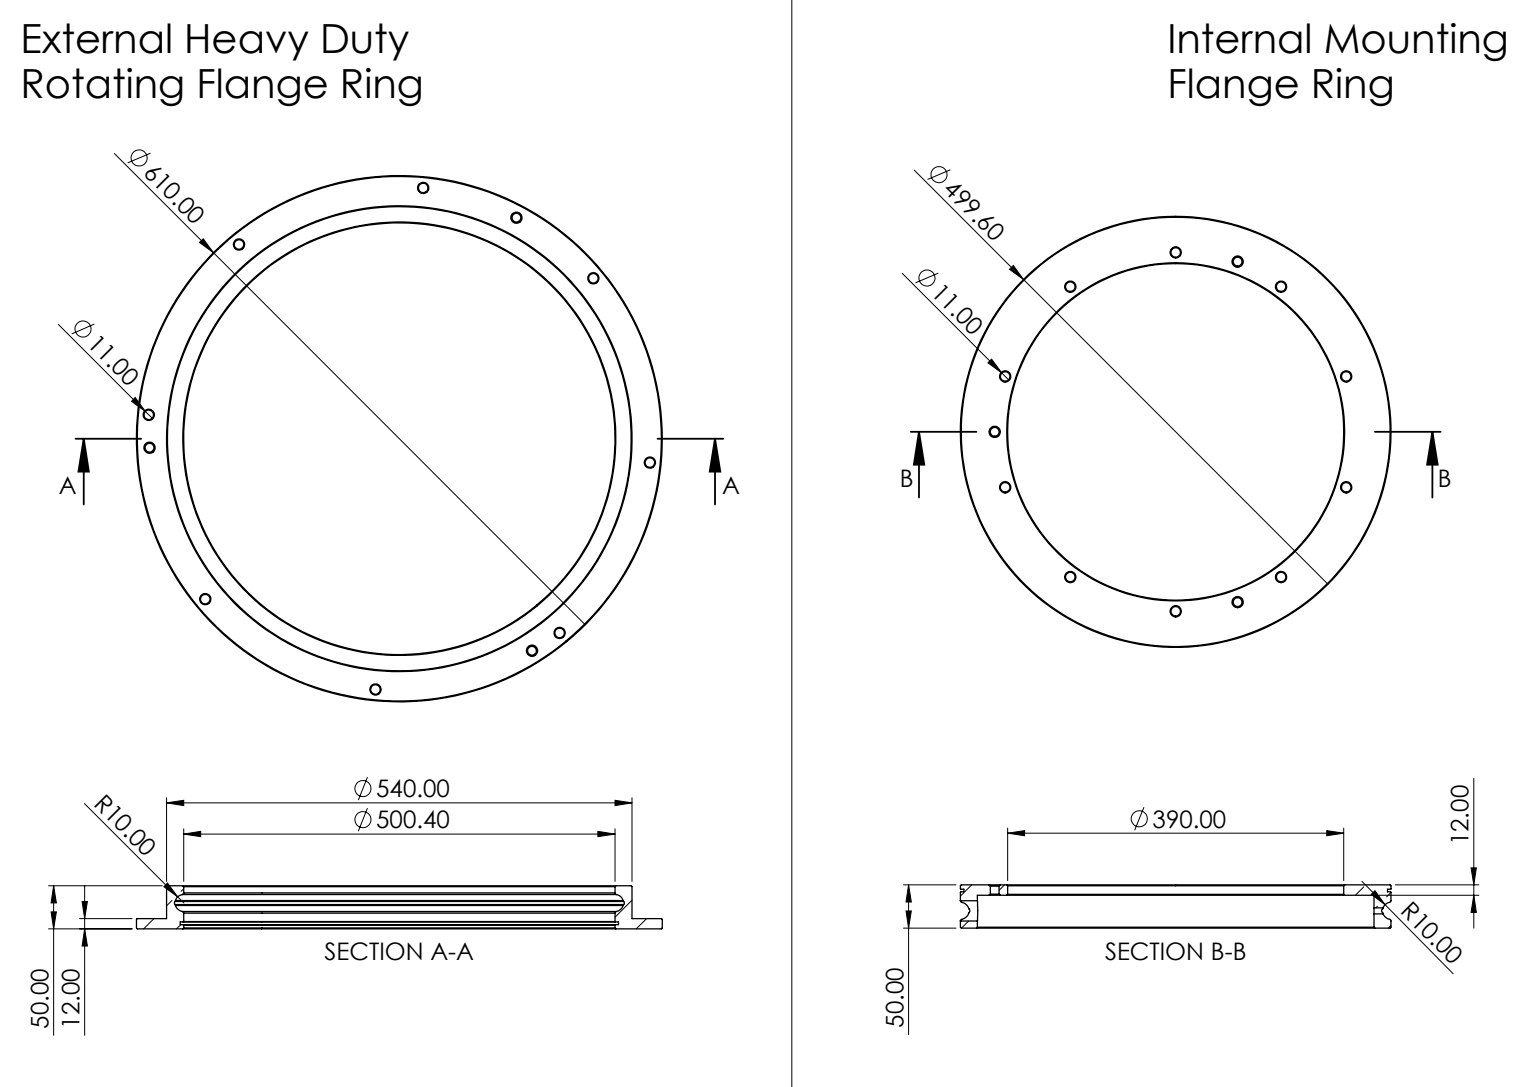
ISO-10303-21;
HEADER;
FILE_DESCRIPTION (('STEP AP214'),
    '1' );
FILE_NAME ('Internal Mounting Flange Ring.step',
    '2026-10-09T12:49:55',
    ( '' ),
    ( '' ),
    'SwSTEP 2.0',
    'SolidWorks 2026',
    '' );
FILE_SCHEMA (( 'AUTOMOTIVE_DESIGN' ));
ENDSEC;

DATA;
#5=TOROIDAL_SURFACE ( 'NONE', #5776, 250.0000000000000000, 10.00000000000000000 ) ;
#9=ORIENTED_EDGE ( 'NONE', *, *, #8914, .T. ) ;
#13=ADVANCED_FACE ( 'NONE', ( #7160 ), #9859, .F. ) ;
#18=CYLINDRICAL_SURFACE ( 'NONE', #6462, 5.500000000000005329 ) ;
#20=CARTESIAN_POINT ( 'NONE',  ( -243.1949234122827193, -7.480730365350286348, 9.061063672199042074 ) ) ;
#22=ORIENTED_EDGE ( 'NONE', *, *, #3438, .F. ) ;
#23=CARTESIAN_POINT ( 'NONE',  ( -230.0000000000000000, 18.00000000000000000, 0.000000000000000000 ) ) ;
#24=LINE ( 'NONE', #4986, #10827 ) ;
#25=CARTESIAN_POINT ( 'NONE',  ( 0.000000000000000000, 22.00000000000000000, 0.000000000000000000 ) ) ;
#28=DIRECTION ( 'NONE',  ( 0.000000000000000000, 1.000000000000000000, 0.000000000000000000 ) ) ;
#29=PLANE ( 'NONE',  #10608 ) ;
#33=CARTESIAN_POINT ( 'NONE',  ( 122.2593324768346008, 18.00000000000000000, 161.7755348299889988 ) ) ;
#36=CARTESIAN_POINT ( 'NONE',  ( -244.7823818444411188, 8.610125652527095497, 7.996289171610727387 ) ) ;
#37=EDGE_LOOP ( 'NONE', ( #12294, #12083 ) ) ;
#43=CARTESIAN_POINT ( 'NONE',  ( 6.735557395310442023E-16, 19.00000000000000000, 213.5000000000000000 ) ) ;
#44=ORIENTED_EDGE ( 'NONE', *, *, #3957, .F. ) ;
#49=CYLINDRICAL_SURFACE ( 'NONE', #12751, 249.7999999999999829 ) ;
#50=CARTESIAN_POINT ( 'NONE',  ( 6.735557395310442023E-16, 19.00000000000000000, -202.4999999999999716 ) ) ;
#58=VERTEX_POINT ( 'NONE', #5076 ) ;
#59=EDGE_CURVE ( 'NONE', #2857, #11921, #819, .T. ) ;
#61=CARTESIAN_POINT ( 'NONE',  ( -249.1369139485392168, 10.36343465138863529, -5.538914405136962316 ) ) ;
#68=DIRECTION ( 'NONE',  ( 8.659560562354926695E-17, 0.7071067811865480168, -0.7071067811865470176 ) ) ;
#70=AXIS2_PLACEMENT_3D ( 'NONE', #7490, #8365, #9292 ) ;
#71=CARTESIAN_POINT ( 'NONE',  ( -245.4148443366356389, -8.946846751066603431, -7.616852152915439156 ) ) ;
#73=CARTESIAN_POINT ( 'NONE',  ( -229.7583704989254443, -5.204493534573133573, 10.54155285988093382 ) ) ;
#78=ORIENTED_EDGE ( 'NONE', *, *, #7931, .F. ) ;
#82=FACE_OUTER_BOUND ( 'NONE', #8092, .T. ) ;
#84=CIRCLE ( 'NONE', #11996, 6.500000000000005329 ) ;
#88=CONICAL_SURFACE ( 'NONE', #12605, 5.500000000000005329, 0.7853981633974461696 ) ;
#89=CARTESIAN_POINT ( 'NONE',  ( -243.1551830321760690, -7.446108171798711872, 9.089443071778552152 ) ) ;
#91=FACE_BOUND ( 'NONE', #3077, .T. ) ;
#98=FACE_BOUND ( 'NONE', #10727, .T. ) ;
#102=CARTESIAN_POINT ( 'NONE',  ( -243.6022064859786269, 7.815160994106106429, 8.774769236968495534 ) ) ;
#103=CONICAL_SURFACE ( 'NONE', #1806, 5.500000000000005329, 0.7853981633974461696 ) ;
#105=EDGE_LOOP ( 'NONE', ( #5377, #568, #8957, #6732 ) ) ;
#107=EDGE_CURVE ( 'NONE', #6490, #4415, #2518, .T. ) ;
#108=EDGE_LOOP ( 'NONE', ( #11966, #7349 ) ) ;
#111=ORIENTED_EDGE ( 'NONE', *, *, #3767, .F. ) ;
#116=CARTESIAN_POINT ( 'NONE',  ( 239.1963018252363042, 1.024882057239583366, 3.346595946712579206 ) ) ;
#117=EDGE_CURVE ( 'NONE', #171, #5643, #5501, .T. ) ;
#119=EDGE_CURVE ( 'NONE', #4577, #1020, #8907, .T. ) ;
#120=CARTESIAN_POINT ( 'NONE',  ( -238.7109915777814138, -2.671037648644427152E-08, -11.74999999995326050 ) ) ;
#121=DIRECTION ( 'NONE',  ( 0.000000000000000000, 1.000000000000000000, 0.000000000000000000 ) ) ;
#127=CIRCLE ( 'NONE', #974, 239.8169934640564804 ) ;
#131=EDGE_LOOP ( 'NONE', ( #6897, #5787, #9258, #12917 ) ) ;
#134=DIRECTION ( 'NONE',  ( 0.000000000000000000, 0.000000000000000000, 1.000000000000000000 ) ) ;
#135=EDGE_CURVE ( 'NONE', #12433, #12610, #12359, .T. ) ;
#136=CARTESIAN_POINT ( 'NONE',  ( -243.1925160140377216, -7.478514340598183097, -9.062807757124144103 ) ) ;
#137=ADVANCED_FACE ( 'NONE', ( #98, #7027 ), #29, .F. ) ;
#139=CARTESIAN_POINT ( 'NONE',  ( 240.4181131690920097, 2.891045149275324633, 1.982248008065000233 ) ) ;
#143=ORIENTED_EDGE ( 'NONE', *, *, #1183, .T. ) ;
#144=ORIENTED_EDGE ( 'NONE', *, *, #3305, .F. ) ;
#146=FACE_OUTER_BOUND ( 'NONE', #6350, .T. ) ;
#147=CARTESIAN_POINT ( 'NONE',  ( 239.5387464286556565, -1.581210110862248941, -3.124650852508605858 ) ) ;
#149=DIRECTION ( 'NONE',  ( 0.000000000000000000, 1.000000000000000000, 0.000000000000000000 ) ) ;
#150=CARTESIAN_POINT ( 'NONE',  ( 0.000000000000000000, -9.830508068699650437, 0.000000000000000000 ) ) ;
#152=CARTESIAN_POINT ( 'NONE',  ( -246.6649006625763718, -9.461692665201230312, 6.966985664009688328 ) ) ;
#154=EDGE_LOOP ( 'NONE', ( #1351, #3008, #4241, #9314 ) ) ;
#155=CARTESIAN_POINT ( 'NONE',  ( 240.6084075703383292, -3.437342788167941698, 0.6677429272691086659 ) ) ;
#156=CARTESIAN_POINT ( 'NONE',  ( 229.9948761773756587, -3.146545554286515056, -1.549783278019676303 ) ) ;
#157=VERTEX_POINT ( 'NONE', #8121 ) ;
#158=VERTEX_POINT ( 'NONE', #1956 ) ;
#159=CARTESIAN_POINT ( 'NONE',  ( 122.2593324768334071, 18.00000000000000000, -168.2755348299895104 ) ) ;
#160=DIRECTION ( 'NONE',  ( 0.000000000000000000, 1.000000000000000000, 0.000000000000000000 ) ) ;
#166=CARTESIAN_POINT ( 'NONE',  ( -242.4885533041308179, 6.811171349317773682, 9.574815119040657407 ) ) ;
#167=VERTEX_POINT ( 'NONE', #4213 ) ;
#171=VERTEX_POINT ( 'NONE', #8621 ) ;
#176=ADVANCED_FACE ( 'NONE', ( #6424 ), #11036, .F. ) ;
#178=DIRECTION ( 'NONE',  ( 0.000000000000000000, 0.000000000000000000, 1.000000000000000000 ) ) ;
#180=LINE ( 'NONE', #8188, #691 ) ;
#184=EDGE_LOOP ( 'NONE', ( #4999, #5010, #6703, #1968 ) ) ;
#185=DIRECTION ( 'NONE',  ( 0.000000000000000000, 0.000000000000000000, 1.000000000000000000 ) ) ;
#186=DIRECTION ( 'NONE',  ( 0.000000000000000000, 1.000000000000000000, 0.000000000000000000 ) ) ;
#188=CIRCLE ( 'NONE', #5900, 6.499999999999999112 ) ;
#189=EDGE_LOOP ( 'NONE', ( #9728, #4932, #9679, #1428 ) ) ;
#192=AXIS2_PLACEMENT_3D ( 'NONE', #6124, #12263, #134 ) ;
#196=CARTESIAN_POINT ( 'NONE',  ( -246.9758887735252699, -9.561393943077655777, -6.829510937495726353 ) ) ;
#197=CIRCLE ( 'NONE', #11695, 196.0000000000000000 ) ;
#199=CARTESIAN_POINT ( 'NONE',  ( 240.6075165363340318, 3.437532598196324063, 0.7648284528981581509 ) ) ;
#200=EDGE_CURVE ( 'NONE', #7619, #9887, #12317, .T. ) ;
#201=EDGE_CURVE ( 'NONE', #6448, #6354, #188, .T. ) ;
#203=CIRCLE ( 'NONE', #9142, 2.000000000000001776 ) ;
#207=CARTESIAN_POINT ( 'NONE',  ( -248.9051445890450225, 10.17462340872661741, 5.878044170807267044 ) ) ;
#208=DIRECTION ( 'NONE',  ( 0.000000000000000000, 0.7071067811865480168, 0.7071067811865470176 ) ) ;
#209=DIRECTION ( 'NONE',  ( 8.659560562354913137E-17, -0.7071067811865489050, 0.7071067811865460184 ) ) ;
#211=DIRECTION ( 'NONE',  ( 0.000000000000000000, 0.000000000000000000, 1.000000000000000000 ) ) ;
#215=ORIENTED_EDGE ( 'NONE', *, *, #11212, .T. ) ;
#216=DIRECTION ( 'NONE',  ( 0.000000000000000000, 0.000000000000000000, 1.000000000000000000 ) ) ;
#218=EDGE_CURVE ( 'NONE', #9833, #1462, #5421, .T. ) ;
#221=ORIENTED_EDGE ( 'NONE', *, *, #12738, .T. ) ;
#223=FACE_OUTER_BOUND ( 'NONE', #154, .T. ) ;
#224=DIRECTION ( 'NONE',  ( 0.000000000000000000, 0.000000000000000000, 1.000000000000000000 ) ) ;
#228=DIRECTION ( 'NONE',  ( 0.000000000000000000, 0.000000000000000000, 1.000000000000000000 ) ) ;
#234=ORIENTED_EDGE ( 'NONE', *, *, #10382, .T. ) ;
#238=DIRECTION ( 'NONE',  ( 0.000000000000000000, 1.000000000000000000, 0.000000000000000000 ) ) ;
#243=DIRECTION ( 'NONE',  ( 0.000000000000000000, -0.7071067811865489050, -0.7071067811865460184 ) ) ;
#247=AXIS2_PLACEMENT_3D ( 'NONE', #6656, #10577, #2507 ) ;
#248=CARTESIAN_POINT ( 'NONE',  ( -249.2724874750463755, -10.50618518648515476, 5.261424415983393388 ) ) ;
#249=ORIENTED_EDGE ( 'NONE', *, *, #11663, .F. ) ;
#254=DIRECTION ( 'NONE',  ( 0.000000000000000000, 0.000000000000000000, 1.000000000000000000 ) ) ;
#259=CARTESIAN_POINT ( 'NONE',  ( -229.9627996858143888, 10.99879348686639879, 4.151745503392231029 ) ) ;
#260=AXIS2_PLACEMENT_3D ( 'NONE', #6805, #2654, #10860 ) ;
#261=FILL_AREA_STYLE_COLOUR ( '', #9272 ) ;
#265=AXIS2_PLACEMENT_3D ( 'NONE', #9269, #11198, #3992 ) ;
#267=ORIENTED_EDGE ( 'NONE', *, *, #6171, .T. ) ;
#273=CARTESIAN_POINT ( 'NONE',  ( -249.2624683435426789, 10.49496574114239422, 5.283769351005206616 ) ) ;
#274=CARTESIAN_POINT ( 'NONE',  ( 122.2593324768334071, 30.00000000000000000, -161.7755348299894820 ) ) ;
#281=AXIS2_PLACEMENT_3D ( 'NONE', #8351, #12412, #4459 ) ;
#287=CARTESIAN_POINT ( 'NONE',  ( 0.000000000000000000, 2.772967769359004908, 0.000000000000000000 ) ) ;
#288=EDGE_LOOP ( 'NONE', ( #12624, #10639, #6520, #4840 ) ) ;
#293=AXIS2_PLACEMENT_3D ( 'NONE', #2741, #11961, #3821 ) ;
#295=CIRCLE ( 'NONE', #1567, 239.8169934640465044 ) ;
#297=ADVANCED_FACE ( 'NONE', ( #1482 ), #8875, .F. ) ;
#301=DIRECTION ( 'NONE',  ( 0.000000000000000000, 1.000000000000000000, 0.000000000000000000 ) ) ;
#305=CIRCLE ( 'NONE', #7745, 5.099999999999993427 ) ;
#306=EDGE_CURVE ( 'NONE', #11150, #4193, #9937, .T. ) ;
#309=ORIENTED_EDGE ( 'NONE', *, *, #7048, .F. ) ;
#310=ORIENTED_EDGE ( 'NONE', *, *, #416, .T. ) ;
#311=AXIS2_PLACEMENT_3D ( 'NONE', #3386, #11606, #6408 ) ;
#312=FACE_OUTER_BOUND ( 'NONE', #9369, .T. ) ;
#315=CARTESIAN_POINT ( 'NONE',  ( 239.0883580245759390, 0.7438334345102074474, -3.420275401504354829 ) ) ;
#316=CARTESIAN_POINT ( 'NONE',  ( -238.9443187634071535, 1.049086267421483143, -11.70307442294971345 ) ) ;
#323=DIRECTION ( 'NONE',  ( 0.000000000000000000, 1.000000000000000000, 0.000000000000000000 ) ) ;
#325=CIRCLE ( 'NONE', #4146, 5.500000000000005329 ) ;
#331=FACE_OUTER_BOUND ( 'NONE', #10588, .T. ) ;
#333=( NAMED_UNIT ( * ) PLANE_ANGLE_UNIT ( ) SI_UNIT ( $, .RADIAN. ) );
#334=PRODUCT ( 'Internal Mounting Flange Ring', 'Internal Mounting Flange Ring', '', ( #7461 ) ) ;
#336=CARTESIAN_POINT ( 'NONE',  ( 240.5727840947670870, 3.342302961292221486, -1.043131940273720026 ) ) ;
#338=CARTESIAN_POINT ( 'NONE',  ( -122.2593324768321992, 29.00000000000000000, 168.2755348299905052 ) ) ;
#339=EDGE_LOOP ( 'NONE', ( #8886, #5505, #9, #5827 ) ) ;
#340=CIRCLE ( 'NONE', #3522, 6.500000000000005329 ) ;
#342=CARTESIAN_POINT ( 'NONE',  ( -210.0000000000000000, 30.00000000000000000, -5.100000000000000533 ) ) ;
#343=DIRECTION ( 'NONE',  ( 0.000000000000000000, 1.000000000000000000, 0.000000000000000000 ) ) ;
#345=DIRECTION ( 'NONE',  ( 0.000000000000000000, 0.000000000000000000, -1.000000000000000000 ) ) ;
#349=LINE ( 'NONE', #3328, #6709 ) ;
#351=CARTESIAN_POINT ( 'NONE',  ( 240.5500529090736279, -3.279976618992322734, -1.225241158514834394 ) ) ;
#359=FACE_OUTER_BOUND ( 'NONE', #11465, .T. ) ;
#362=CARTESIAN_POINT ( 'NONE',  ( -240.4375400852135556, 3.701007121351563622, 11.16264886369179443 ) ) ;
#368=VERTEX_POINT ( 'NONE', #8676 ) ;
#369=ORIENTED_EDGE ( 'NONE', *, *, #5052, .F. ) ;
#371=EDGE_CURVE ( 'NONE', #12258, #9610, #11751, .T. ) ;
#374=CARTESIAN_POINT ( 'NONE',  ( 239.0381261355853724, 0.5585874493560030185, -3.455211367196914463 ) ) ;
#375=EDGE_CURVE ( 'NONE', #2492, #808, #9229, .T. ) ;
#376=CARTESIAN_POINT ( 'NONE',  ( -239.2060318623362321, 1.486384198450626526, -11.65560593358670260 ) ) ;
#381=AXIS2_PLACEMENT_3D ( 'NONE', #10792, #6742, #6676 ) ;
#382=ORIENTED_EDGE ( 'NONE', *, *, #554, .T. ) ;
#387=DIRECTION ( 'NONE',  ( 0.000000000000000000, -1.000000000000000000, 0.000000000000000000 ) ) ;
#389=DIRECTION ( 'NONE',  ( 0.000000000000000000, 0.000000000000000000, 1.000000000000000000 ) ) ;
#390=CARTESIAN_POINT ( 'NONE',  ( -240.6618454235819513, -4.173161342500063320, -10.98396364135015801 ) ) ;
#396=B_SPLINE_CURVE_WITH_KNOTS ( 'NONE', 3,
 ( #120, #5441, #9444, #12376, #8383, #5564, #11439, #6316, #7439, #3497, #2434, #11511, #3229, #10634, #316, #12444, #9502, #1502, #2297, #10366, #3424, #12572, #7508, #376, #1376, #7310, #1308, #6515, #11576, #6574, #4424 ),
 .UNSPECIFIED., .F., .F.,
 ( 4, 2, 1, 1, 1, 2, 2, 2, 2, 1, 1, 2, 2, 2, 1, 1, 2, 2, 4 ),
 ( 0.5000762880526811172, 0.5039819420522705373, 0.5078875960518599575, 0.5156989040510386868, 0.5313215200493963675, 0.5625667520461116178, 0.6250572160395442278, 0.7500381440264094479, 0.7578494520255938394, 0.7656607600247783418, 0.7812833760231472358, 0.8125286080198849126, 0.8750190720133503852, 0.8789247260129398054, 0.8828303800125294476, 0.8906416880116931889, 0.9062643040100208935, 0.9375095360066760808, 1.000000000000000000 ),
 .UNSPECIFIED. ) ;
#397=AXIS2_PLACEMENT_3D ( 'NONE', #3303, #10513, #5447 ) ;
#398=AXIS2_PLACEMENT_3D ( 'NONE', #10071, #9274, #3936 ) ;
#400=DIRECTION ( 'NONE',  ( 0.000000000000000000, 1.000000000000000000, 0.000000000000000000 ) ) ;
#404=LINE ( 'NONE', #12663, #505 ) ;
#405=CYLINDRICAL_SURFACE ( 'NONE', #4254, 11.75000000000000000 ) ;
#407=VECTOR ( 'NONE', #3982, 1000.000000000000114 ) ;
#408=FACE_OUTER_BOUND ( 'NONE', #8960, .T. ) ;
#412=CARTESIAN_POINT ( 'NONE',  ( 240.6009466513765176, -3.417710891889066627, 0.7616916526936037268 ) ) ;
#416=EDGE_CURVE ( 'NONE', #3329, #13033, #7804, .T. ) ;
#421=DIRECTION ( 'NONE',  ( 0.000000000000000000, -1.000000000000000000, 0.000000000000000000 ) ) ;
#422=B_SPLINE_CURVE_WITH_KNOTS ( 'NONE', 3,
 ( #8574, #10632, #5371, #1500, #4556, #3352, #6315, #2239, #11641, #2496, #2295, #7568, #6573, #3423, #441, #6379, #10365, #12442, #4490, #4368, #9501, #315, #7375, #5563, #10436, #374, #8447, #12501, #7437 ),
 .UNSPECIFIED., .F., .F.,
 ( 4, 2, 2, 1, 1, 2, 2, 2, 1, 1, 2, 2, 2, 1, 2, 2, 4 ),
 ( 0.000000000000000000, 0.06264877319316634885, 0.09397315978975546991, 0.1096353530880500721, 0.1174664497371907118, 0.1213819980617677902, 0.1252975463863448546, 0.1879463195796756692, 0.2192707061763410903, 0.2349328994746693877, 0.2427639961238378385, 0.2505950927730062894, 0.3132438659663454028, 0.3445682525630119897, 0.3602304458613453941, 0.3758926391596786876, 0.5011901855463575250 ),
 .UNSPECIFIED. ) ;
#428=EDGE_CURVE ( 'NONE', #612, #7121, #6260, .T. ) ;
#430=AXIS2_PLACEMENT_3D ( 'NONE', #11339, #3065, #7146 ) ;
#433=AXIS2_PLACEMENT_3D ( 'NONE', #11650, #1512, #3568 ) ;
#434=ORIENTED_EDGE ( 'NONE', *, *, #4249, .F. ) ;
#437=EDGE_LOOP ( 'NONE', ( #12968, #8052, #6929, #11620 ) ) ;
#441=CARTESIAN_POINT ( 'NONE',  ( 239.2626306339685982, 1.161280184642565771, -3.302084438317430148 ) ) ;
#443=DIRECTION ( 'NONE',  ( 0.000000000000000000, 0.000000000000000000, 1.000000000000000000 ) ) ;
#448=CIRCLE ( 'NONE', #4682, 5.499999999999998224 ) ;
#451=ORIENTED_EDGE ( 'NONE', *, *, #6978, .F. ) ;
#456=CARTESIAN_POINT ( 'NONE',  ( 0.000000000000000000, 25.50000000000000000, 0.000000000000000000 ) ) ;
#457=CARTESIAN_POINT ( 'NONE',  ( -229.8300945347042159, 7.760684502249874051, 8.855560954721353184 ) ) ;
#460=ADVANCED_FACE ( 'NONE', ( #6754 ), #4532, .F. ) ;
#463=CARTESIAN_POINT ( 'NONE',  ( 71.82423009839129691, 30.00000000000000000, -197.3354503650404865 ) ) ;
#464=EDGE_CURVE ( 'NONE', #12890, #3753, #4734, .T. ) ;
#465=CIRCLE ( 'NONE', #8338, 6.500000000000005329 ) ;
#466=DIRECTION ( 'NONE',  ( 0.000000000000000000, 0.000000000000000000, 1.000000000000000000 ) ) ;
#468=VERTEX_POINT ( 'NONE', #9561 ) ;
#470=DIRECTION ( 'NONE',  ( 0.000000000000000000, 0.000000000000000000, 1.000000000000000000 ) ) ;
#473=CIRCLE ( 'NONE', #10902, 5.500000000000005329 ) ;
#476=CARTESIAN_POINT ( 'NONE',  ( -240.1208361041844910, 2.772967769358964940, -11.41810622433052025 ) ) ;
#478=CARTESIAN_POINT ( 'NONE',  ( 229.9948475045917462, 3.144455231364676084, -1.553991905490903713 ) ) ;
#479=CIRCLE ( 'NONE', #696, 5.500000000000005329 ) ;
#482=FACE_OUTER_BOUND ( 'NONE', #9432, .T. ) ;
#483=DIRECTION ( 'NONE',  ( 8.659560562354939021E-17, 0.7071067811865470176, -0.7071067811865480168 ) ) ;
#485=ORIENTED_EDGE ( 'NONE', *, *, #1724, .F. ) ;
#486=ORIENTED_EDGE ( 'NONE', *, *, #7148, .F. ) ;
#492=DIRECTION ( 'NONE',  ( 0.000000000000000000, 0.000000000000000000, 1.000000000000000000 ) ) ;
#497=VERTEX_POINT ( 'NONE', #8948 ) ;
#499=ORIENTED_EDGE ( 'NONE', *, *, #7130, .T. ) ;
#501=ORIENTED_EDGE ( 'NONE', *, *, #11632, .T. ) ;
#502=ORIENTED_EDGE ( 'NONE', *, *, #3627, .F. ) ;
#505=VECTOR ( 'NONE', #4454, 1000.000000000000000 ) ;
#506=DIRECTION ( 'NONE',  ( 0.000000000000000000, 0.000000000000000000, -1.000000000000000000 ) ) ;
#508=AXIS2_PLACEMENT_3D ( 'NONE', #7743, #6880, #10941 ) ;
#510=DIRECTION ( 'NONE',  ( 0.000000000000000000, -1.000000000000000000, 0.000000000000000000 ) ) ;
#513=AXIS2_PLACEMENT_3D ( 'NONE', #12749, #7424, #11499 ) ;
#516=ORIENTED_EDGE ( 'NONE', *, *, #3019, .F. ) ;
#517=CARTESIAN_POINT ( 'NONE',  ( -243.5599937619014952, 7.782121691016424592, -8.802892736592429657 ) ) ;
#519=EDGE_CURVE ( 'NONE', #3488, #167, #5232, .T. ) ;
#524=DIRECTION ( 'NONE',  ( 0.000000000000000000, 0.000000000000000000, -1.000000000000000000 ) ) ;
#528=AXIS2_PLACEMENT_3D ( 'NONE', #5634, #4617, #3756 ) ;
#532=ORIENTED_EDGE ( 'NONE', *, *, #8990, .T. ) ;
#533=CARTESIAN_POINT ( 'NONE',  ( -122.2593324768359935, 29.00000000000000000, -162.7755348299880040 ) ) ;
#534=VERTEX_POINT ( 'NONE', #9137 ) ;
#540=DIRECTION ( 'NONE',  ( 1.000000000000000000, 0.000000000000000000, 0.000000000000000000 ) ) ;
#544=DIRECTION ( 'NONE',  ( 0.000000000000000000, 0.7071067811865280328, 0.7071067811865670016 ) ) ;
#546=CARTESIAN_POINT ( 'NONE',  ( 229.9884017560907807, 2.634578860511305631, -2.315394940318573624 ) ) ;
#548=AXIS2_PLACEMENT_3D ( 'NONE', #622, #3812, #2548 ) ;
#550=DIRECTION ( 'NONE',  ( 8.659560562354926695E-17, 0.7071067811865480168, -0.7071067811865470176 ) ) ;
#551=EDGE_LOOP ( 'NONE', ( #10115, #7698 ) ) ;
#552=VERTEX_POINT ( 'NONE', #6014 ) ;
#553=CARTESIAN_POINT ( 'NONE',  ( 7.347880794884118750E-16, 29.00000000000000000, 202.4999999999999716 ) ) ;
#554=EDGE_CURVE ( 'NONE', #12610, #6169, #9285, .T. ) ;
#560=FACE_OUTER_BOUND ( 'NONE', #6115, .T. ) ;
#563=FACE_OUTER_BOUND ( 'NONE', #5860, .T. ) ;
#568=ORIENTED_EDGE ( 'NONE', *, *, #1085, .T. ) ;
#569=DIRECTION ( 'NONE',  ( 0.000000000000000000, 0.000000000000000000, 1.000000000000000000 ) ) ;
#570=FACE_OUTER_BOUND ( 'NONE', #8193, .T. ) ;
#572=ORIENTED_EDGE ( 'NONE', *, *, #10231, .F. ) ;
#573=DIRECTION ( 'NONE',  ( 0.000000000000000000, 0.000000000000000000, 1.000000000000000000 ) ) ;
#574=EDGE_LOOP ( 'NONE', ( #7370, #1369 ) ) ;
#576=CARTESIAN_POINT ( 'NONE',  ( -244.2253259530033063, 8.263305842943061919, -8.353459642338018298 ) ) ;
#578=ADVANCED_FACE ( 'NONE', ( #10195 ), #8912, .T. ) ;
#579=EDGE_CURVE ( 'NONE', #3020, #10014, #12322, .T. ) ;
#580=CARTESIAN_POINT ( 'NONE',  ( 240.3599429726558299, -2.697249171038460069, -2.233886006210043629 ) ) ;
#583=DIRECTION ( 'NONE',  ( 0.000000000000000000, 1.000000000000000000, 0.000000000000000000 ) ) ;
#588=DIRECTION ( 'NONE',  ( 0.000000000000000000, 1.000000000000000000, 0.000000000000000000 ) ) ;
#589=ORIENTED_EDGE ( 'NONE', *, *, #10916, .T. ) ;
#590=ORIENTED_EDGE ( 'NONE', *, *, #10836, .F. ) ;
#593=AXIS2_PLACEMENT_3D ( 'NONE', #7570, #8695, #1632 ) ;
#596=CARTESIAN_POINT ( 'NONE',  ( 0.000000000000000000, 9.830508068699479907, 0.000000000000000000 ) ) ;
#602=ADVANCED_FACE ( 'NONE', ( #12211 ), #1031, .T. ) ;
#608=CARTESIAN_POINT ( 'NONE',  ( -248.8555022324198092, 10.14371006999433789, -5.930260235961137383 ) ) ;
#610=CARTESIAN_POINT ( 'NONE',  ( 197.8197553893920144, 18.00000000000000000, 64.27553482998850143 ) ) ;
#611=EDGE_LOOP ( 'NONE', ( #7240, #5539, #12625, #572 ) ) ;
#612=VERTEX_POINT ( 'NONE', #7075 ) ;
#618=AXIS2_PLACEMENT_3D ( 'NONE', #4311, #11452, #1830 ) ;
#621=DIRECTION ( 'NONE',  ( 0.000000000000000000, 1.000000000000000000, 0.000000000000000000 ) ) ;
#622=CARTESIAN_POINT ( 'NONE',  ( 0.000000000000000000, -2.957522019940860139E-14, 0.000000000000000000 ) ) ;
#623=AXIS2_PLACEMENT_3D ( 'NONE', #5398, #3520, #1527 ) ;
#624=EDGE_CURVE ( 'NONE', #1954, #9495, #12952, .T. ) ;
#625=ORIENTED_EDGE ( 'NONE', *, *, #1514, .F. ) ;
#627=DIRECTION ( 'NONE',  ( 0.000000000000000000, 1.000000000000000000, 0.000000000000000000 ) ) ;
#629=ORIENTED_EDGE ( 'NONE', *, *, #6249, .T. ) ;
#632=AXIS2_PLACEMENT_3D ( 'NONE', #23, #5012, #3948 ) ;
#636=CIRCLE ( 'NONE', #9776, 6.500000000000005329 ) ;
#638=CARTESIAN_POINT ( 'NONE',  ( -247.4721532356705040, 9.698102444925263299, 6.633777139661048317 ) ) ;
#640=EDGE_LOOP ( 'NONE', ( #3400, #6010, #3951, #10562, #8054 ) ) ;
#642=ORIENTED_EDGE ( 'NONE', *, *, #9370, .T. ) ;
#643=CARTESIAN_POINT ( 'NONE',  ( -242.9854649084194023, 7.295305385232032869, -9.211094753746992936 ) ) ;
#646=CARTESIAN_POINT ( 'NONE',  ( 122.2593324768346008, 18.00000000000000000, 168.2755348299889988 ) ) ;
#649=CARTESIAN_POINT ( 'NONE',  ( 0.000000000000000000, -2.957522019940860139E-14, -241.5000000000000000 ) ) ;
#650=CARTESIAN_POINT ( 'NONE',  ( -230.0000324180956568, 11.75063456719393606, -0.7654011193310154004 ) ) ;
#651=CONICAL_SURFACE ( 'NONE', #1504, 5.099999999999993427, 0.7853981633974461696 ) ;
#654=ORIENTED_EDGE ( 'NONE', *, *, #2803, .T. ) ;
#659=TOROIDAL_SURFACE ( 'NONE', #5728, 241.5000000000000000, 2.500000000000000000 ) ;
#661=ORIENTED_EDGE ( 'NONE', *, *, #5302, .F. ) ;
#662=DIRECTION ( 'NONE',  ( 0.000000000000000000, -1.000000000000000000, 0.000000000000000000 ) ) ;
#672=CARTESIAN_POINT ( 'NONE',  ( -229.9566917300585942, -10.87227007594808192, -4.504975736512506046 ) ) ;
#674=CARTESIAN_POINT ( 'NONE',  ( -249.7825649081718780, 11.59499477621177910, 1.902498382194837578 ) ) ;
#675=CARTESIAN_POINT ( 'NONE',  ( 0.000000000000000000, 2.772967769359004908, -240.3921568627450256 ) ) ;
#677=DIRECTION ( 'NONE',  ( 0.000000000000000000, 0.000000000000000000, -1.000000000000000000 ) ) ;
#678=VERTEX_POINT ( 'NONE', #11072 ) ;
#682=ADVANCED_FACE ( 'NONE', ( #146 ), #11138, .F. ) ;
#687=CARTESIAN_POINT ( 'NONE',  ( 240.3826708216974737, -2.772967769359219847, 2.135567781667135012 ) ) ;
#691=VECTOR ( 'NONE', #2042, 1000.000000000000000 ) ;
#692=LINE ( 'NONE', #9946, #1305 ) ;
#694=ORIENTED_EDGE ( 'NONE', *, *, #9006, .T. ) ;
#696=AXIS2_PLACEMENT_3D ( 'NONE', #9666, #11747, #10546 ) ;
#698=ORIENTED_EDGE ( 'NONE', *, *, #11298, .T. ) ;
#700=AXIS2_PLACEMENT_3D ( 'NONE', #1617, #9734, #9880 ) ;
#703=CARTESIAN_POINT ( 'NONE',  ( -239.6752751780965411, 1.974315850608226564, -11.58364238450999828 ) ) ;
#704=VECTOR ( 'NONE', #243, 1000.000000000000114 ) ;
#709=ORIENTED_EDGE ( 'NONE', *, *, #6978, .T. ) ;
#714=CARTESIAN_POINT ( 'NONE',  ( -243.2974363841306342, 7.571041528465444870, -8.986772684112915854 ) ) ;
#717=CARTESIAN_POINT ( 'NONE',  ( 0.000000000000000000, -9.830508068699650437, 0.000000000000000000 ) ) ;
#719=FACE_OUTER_BOUND ( 'NONE', #9816, .T. ) ;
#721=CARTESIAN_POINT ( 'NONE',  ( -229.8304973814411198, 7.772590954318897793, -8.845180372341092223 ) ) ;
#722=FACE_BOUND ( 'NONE', #905, .T. ) ;
#731=AXIS2_PLACEMENT_3D ( 'NONE', #10333, #9339, #1339 ) ;
#732=CARTESIAN_POINT ( 'NONE',  ( -249.5790707039662948, -10.95560708710130271, -4.250203459824828833 ) ) ;
#733=ORIENTED_EDGE ( 'NONE', *, *, #1557, .F. ) ;
#734=CIRCLE ( 'NONE', #3057, 245.7999999999999829 ) ;
#737=CARTESIAN_POINT ( 'NONE',  ( 0.000000000000000000, -9.830508068699650437, 248.1666666666509968 ) ) ;
#739=CARTESIAN_POINT ( 'NONE',  ( -240.1208361041844910, 2.772967769358974710, 11.41810622433049893 ) ) ;
#742=CARTESIAN_POINT ( 'NONE',  ( 71.82423009839129691, 30.00000000000000000, 202.4354503650404808 ) ) ;
#744=CARTESIAN_POINT ( 'NONE',  ( 230.0000029335025147, 3.500192773088487641, 0.2278275254128714344 ) ) ;
#746=CARTESIAN_POINT ( 'NONE',  ( -249.7834965322842322, 11.60135170607461319, 1.863160430829968517 ) ) ;
#749=ORIENTED_EDGE ( 'NONE', *, *, #1670, .T. ) ;
#754=ADVANCED_FACE ( 'NONE', ( #2461 ), #10175, .T. ) ;
#755=EDGE_CURVE ( 'NONE', #10156, #9288, #11337, .T. ) ;
#759=CYLINDRICAL_SURFACE ( 'NONE', #5399, 5.499999999999998224 ) ;
#760=CARTESIAN_POINT ( 'NONE',  ( 240.1689872792136384, 2.295088600363839770, -2.642490611638467879 ) ) ;
#762=EDGE_LOOP ( 'NONE', ( #5995, #10511, #5433, #10109 ) ) ;
#763=EDGE_CURVE ( 'NONE', #157, #9833, #7746, .T. ) ;
#765=ORIENTED_EDGE ( 'NONE', *, *, #8990, .F. ) ;
#766=ORIENTED_EDGE ( 'NONE', *, *, #2370, .F. ) ;
#768=ORIENTED_EDGE ( 'NONE', *, *, #6579, .T. ) ;
#771=DIRECTION ( 'NONE',  ( 0.000000000000000000, 0.7071067811865480168, 0.7071067811865470176 ) ) ;
#772=CARTESIAN_POINT ( 'NONE',  ( -247.3964713742791446, 9.678883351029913484, 6.661754107376391509 ) ) ;
#773=ORIENTED_EDGE ( 'NONE', *, *, #9622, .T. ) ;
#777=ADVANCED_FACE ( 'NONE', ( #6476 ), #6340, .T. ) ;
#778=CARTESIAN_POINT ( 'NONE',  ( -238.7109915794538892, 0.3295697628469637097, 11.74999996399578350 ) ) ;
#781=DIRECTION ( 'NONE',  ( 0.000000000000000000, 1.000000000000000000, 0.000000000000000000 ) ) ;
#782=FACE_OUTER_BOUND ( 'NONE', #10358, .T. ) ;
#783=FACE_BOUND ( 'NONE', #7105, .T. ) ;
#787=ORIENTED_EDGE ( 'NONE', *, *, #3681, .T. ) ;
#789=VERTEX_POINT ( 'NONE', #6537 ) ;
#790=EDGE_CURVE ( 'NONE', #1462, #3155, #6053, .T. ) ;
#792=CARTESIAN_POINT ( 'NONE',  ( -248.3468897632307062, -9.892776367366600709, -6.340645126513342333 ) ) ;
#793=ORIENTED_EDGE ( 'NONE', *, *, #10673, .F. ) ;
#796=CARTESIAN_POINT ( 'NONE',  ( 122.2593324768334071, 18.00000000000000000, -174.7755348299895104 ) ) ;
#799=CIRCLE ( 'NONE', #8038, 5.499999999999998224 ) ;
#800=CARTESIAN_POINT ( 'NONE',  ( 2.400307726328812375E-14, 30.00000000000000000, -196.0000000000000000 ) ) ;
#802=CARTESIAN_POINT ( 'NONE',  ( 2.822810872034648951E-14, -19.00000000000000000, 230.0000000000000000 ) ) ;
#804=CARTESIAN_POINT ( 'NONE',  ( -249.7894049735008650, 11.64306034551006164, 1.598052593220072648 ) ) ;
#805=AXIS2_PLACEMENT_3D ( 'NONE', #6711, #10765, #10635 ) ;
#808=VERTEX_POINT ( 'NONE', #10590 ) ;
#812=DIRECTION ( 'NONE',  ( 0.000000000000000000, 0.000000000000000000, 1.000000000000000000 ) ) ;
#816=EDGE_CURVE ( 'NONE', #2672, #10498, #2429, .T. ) ;
#817=FACE_BOUND ( 'NONE', #8599, .T. ) ;
#818=ADVANCED_FACE ( 'NONE', ( #7398, #11406 ), #2262, .F. ) ;
#819=CIRCLE ( 'NONE', #1885, 248.7999999999999829 ) ;
#822=CIRCLE ( 'NONE', #397, 6.500000000000005329 ) ;
#826=FACE_OUTER_BOUND ( 'NONE', #9682, .T. ) ;
#827=ORIENTED_EDGE ( 'NONE', *, *, #946, .T. ) ;
#835=CIRCLE ( 'NONE', #6157, 248.1666666666679930 ) ;
#839=AXIS2_PLACEMENT_3D ( 'NONE', #4366, #3158, #8314 ) ;
#840=CARTESIAN_POINT ( 'NONE',  ( -239.1986675888292382, 1.476433811303769383, 11.65687006326614039 ) ) ;
#841=ORIENTED_EDGE ( 'NONE', *, *, #4349, .T. ) ;
#843=CARTESIAN_POINT ( 'NONE',  ( 240.3318468624802620, -2.620158398456138737, -2.323190430600380108 ) ) ;
#844=CARTESIAN_POINT ( 'NONE',  ( 0.000000000000000000, -19.00000000000000000, 0.000000000000000000 ) ) ;
#845=CARTESIAN_POINT ( 'NONE',  ( 0.000000000000000000, 21.50000000000000000, 0.000000000000000000 ) ) ;
#846=EDGE_CURVE ( 'NONE', #5331, #11051, #9586, .T. ) ;
#847=CARTESIAN_POINT ( 'NONE',  ( -229.6996680450365886, 0.7763087779090785956, -11.75000000000000178 ) ) ;
#849=DIRECTION ( 'NONE',  ( 0.000000000000000000, -1.000000000000000000, 0.000000000000000000 ) ) ;
#854=CARTESIAN_POINT ( 'NONE',  ( -238.7109915777963636, -0.006372640623321836582, -11.74999999916455984 ) ) ;
#858=CARTESIAN_POINT ( 'NONE',  ( -249.2136238162158577, -10.44210856422258082, -5.387711592263697113 ) ) ;
#861=LINE ( 'NONE', #4921, #12650 ) ;
#869=CARTESIAN_POINT ( 'NONE',  ( -229.9163789481184494, -9.982432720316847252, 6.209677335868705406 ) ) ;
#870=EDGE_CURVE ( 'NONE', #678, #3753, #734, .T. ) ;
#872=DIRECTION ( 'NONE',  ( 0.000000000000000000, -1.000000000000000000, 0.000000000000000000 ) ) ;
#874=ORIENTED_EDGE ( 'NONE', *, *, #3863, .F. ) ;
#880=CARTESIAN_POINT ( 'NONE',  ( 0.000000000000000000, 30.00000000000000000, -208.0000000000000000 ) ) ;
#882=CARTESIAN_POINT ( 'NONE',  ( -245.3969493176729486, -8.938055201230712399, 7.627167029050283986 ) ) ;
#889=VERTEX_POINT ( 'NONE', #7468 ) ;
#892=DIRECTION ( 'NONE',  ( 0.000000000000000000, -1.000000000000000000, 0.000000000000000000 ) ) ;
#897=DIRECTION ( 'NONE',  ( 0.000000000000000000, 0.000000000000000000, 1.000000000000000000 ) ) ;
#899=CARTESIAN_POINT ( 'NONE',  ( -246.6923348789300974, 9.470909649984781353, 6.954450552248236050 ) ) ;
#901=DIRECTION ( 'NONE',  ( 0.000000000000000000, 1.000000000000000000, 0.000000000000000000 ) ) ;
#902=VECTOR ( 'NONE', #1414, 1000.000000000000000 ) ;
#904=CARTESIAN_POINT ( 'NONE',  ( -245.6300371787731365, 9.052739546773430845, -7.492707602044229809 ) ) ;
#905=EDGE_LOOP ( 'NONE', ( #12477, #7810 ) ) ;
#906=VECTOR ( 'NONE', #7554, 1000.000000000000000 ) ;
#909=DIRECTION ( 'NONE',  ( 0.000000000000000000, 0.000000000000000000, 1.000000000000000000 ) ) ;
#912=DIRECTION ( 'NONE',  ( 0.000000000000000000, -1.000000000000000000, 0.000000000000000000 ) ) ;
#913=CARTESIAN_POINT ( 'NONE',  ( 0.000000000000000000, 30.00000000000000000, 214.5000000000000000 ) ) ;
#917=AXIS2_PLACEMENT_3D ( 'NONE', #6215, #3326, #2401 ) ;
#921=CARTESIAN_POINT ( 'NONE',  ( 0.000000000000000000, -2.772967769359314882, 0.000000000000000000 ) ) ;
#923=ADVANCED_FACE ( 'NONE', ( #5595 ), #11154, .F. ) ;
#924=ORIENTED_EDGE ( 'NONE', *, *, #10395, .F. ) ;
#925=CARTESIAN_POINT ( 'NONE',  ( -249.7854625206820174, -11.61528754001802000, 1.774251678600656579 ) ) ;
#928=CIRCLE ( 'NONE', #6884, 6.500000000000005329 ) ;
#937=CARTESIAN_POINT ( 'NONE',  ( -229.7834611933087103, -6.213105212076664330, 9.980295640892103748 ) ) ;
#939=ADVANCED_FACE ( 'NONE', ( #6672 ), #10407, .F. ) ;
#940=DIRECTION ( 'NONE',  ( 0.000000000000000000, 1.000000000000000000, 0.000000000000000000 ) ) ;
#946=EDGE_CURVE ( 'NONE', #9833, #6599, #2775, .T. ) ;
#947=CARTESIAN_POINT ( 'NONE',  ( 122.2593324768334071, 30.00000000000000000, -174.7755348299895104 ) ) ;
#948=CYLINDRICAL_SURFACE ( 'NONE', #11772, 5.500000000000005329 ) ;
#951=CARTESIAN_POINT ( 'NONE',  ( -245.1951802402266196, -8.836085397833034705, 7.745290892887734202 ) ) ;
#956=EDGE_CURVE ( 'NONE', #1185, #6599, #12116, .T. ) ;
#961=ORIENTED_EDGE ( 'NONE', *, *, #1670, .F. ) ;
#962=CARTESIAN_POINT ( 'NONE',  ( -248.5304950464277454, 9.965644880941075812, 6.224989825353040018 ) ) ;
#966=CARTESIAN_POINT ( 'NONE',  ( -241.4660365534715822, 5.559932089232387575, 10.35152193433334311 ) ) ;
#967=EDGE_LOOP ( 'NONE', ( #4621, #2287, #10425, #1560 ) ) ;
#970=CARTESIAN_POINT ( 'NONE',  ( -238.9359159396491634, 1.030912813916464055, 11.70469087026479826 ) ) ;
#972=TOROIDAL_SURFACE ( 'NONE', #548, 241.5000000000000000, 2.500000000000000000 ) ;
#974=AXIS2_PLACEMENT_3D ( 'NONE', #10227, #10426, #7369 ) ;
#976=CARTESIAN_POINT ( 'NONE',  ( 0.000000000000000000, -2.772967769359314882, 0.000000000000000000 ) ) ;
#977=CARTESIAN_POINT ( 'NONE',  ( 239.1385365879787344, 0.8886010998292401819, 3.385772393335270358 ) ) ;
#979=FACE_OUTER_BOUND ( 'NONE', #7181, .T. ) ;
#982=VERTEX_POINT ( 'NONE', #9713 ) ;
#988=CARTESIAN_POINT ( 'NONE',  ( -249.4432382448479473, -10.72467464912286239, 4.802290507069141512 ) ) ;
#992=CYLINDRICAL_SURFACE ( 'NONE', #8296, 11.75000000000000000 ) ;
#993=CARTESIAN_POINT ( 'NONE',  ( -245.4266968893038268, -8.952647108764159256, -7.610034336731980709 ) ) ;
#1001=VERTEX_POINT ( 'NONE', #9655 ) ;
#1002=ORIENTED_EDGE ( 'NONE', *, *, #11588, .T. ) ;
#1006=EDGE_CURVE ( 'NONE', #5643, #171, #9763, .T. ) ;
#1008=EDGE_CURVE ( 'NONE', #3488, #5812, #6737, .T. ) ;
#1009=LINE ( 'NONE', #4940, #1131 ) ;
#1014=EDGE_LOOP ( 'NONE', ( #2566, #12900, #7199, #5656 ) ) ;
#1015=DIRECTION ( 'NONE',  ( 1.224646799147349509E-16, 0.000000000000000000, -1.000000000000000000 ) ) ;
#1016=CARTESIAN_POINT ( 'NONE',  ( 229.9799723853240039, -1.753250733347112345, 3.037834540539402717 ) ) ;
#1017=VERTEX_POINT ( 'NONE', #7790 ) ;
#1020=VERTEX_POINT ( 'NONE', #10729 ) ;
#1026=CARTESIAN_POINT ( 'NONE',  ( -246.7886136405148818, 9.502664448782068618, 6.911022175809039325 ) ) ;
#1030=EDGE_CURVE ( 'NONE', #3384, #7222, #197, .T. ) ;
#1031=TOROIDAL_SURFACE ( 'NONE', #11888, 238.4705882352940307, 2.000000000000000000 ) ;
#1034=CARTESIAN_POINT ( 'NONE',  ( -245.3907676186766764, 8.935007734144498670, -7.630737089751100655 ) ) ;
#1036=CARTESIAN_POINT ( 'NONE',  ( 3.059167704270088292E-14, -19.00000000000000000, -249.7999999999999545 ) ) ;
#1038=CARTESIAN_POINT ( 'NONE',  ( 239.3703217814042716, 1.345486616892404230, 3.231439195586080171 ) ) ;
#1045=VERTEX_POINT ( 'NONE', #7723 ) ;
#1046=CARTESIAN_POINT ( 'NONE',  ( -239.2239471121744998, -1.510219381902923264, -11.65254212220749075 ) ) ;
#1048=ORIENTED_EDGE ( 'NONE', *, *, #200, .T. ) ;
#1049=CARTESIAN_POINT ( 'NONE',  ( -249.3105109839077045, 10.55009524027425982, -5.172972615342095182 ) ) ;
#1051=VECTOR ( 'NONE', #5097, 1000.000000000000114 ) ;
#1052=CARTESIAN_POINT ( 'NONE',  ( -249.7763361841028882, -11.55065150920177075, 2.186104016062915711 ) ) ;
#1056=VECTOR ( 'NONE', #2935, 1000.000000000000114 ) ;
#1057=DIRECTION ( 'NONE',  ( 0.000000000000000000, 1.000000000000000000, 0.000000000000000000 ) ) ;
#1058=CARTESIAN_POINT ( 'NONE',  ( -245.0777337248563299, -8.776737537879517603, -7.814324104198428600 ) ) ;
#1063=CARTESIAN_POINT ( 'NONE',  ( -229.9700272232702503, -11.15178693234673801, 3.780588754129759810 ) ) ;
#1066=ORIENTED_EDGE ( 'NONE', *, *, #7505, .F. ) ;
#1069=DIRECTION ( 'NONE',  ( 0.000000000000000000, 0.000000000000000000, -1.000000000000000000 ) ) ;
#1072=DIRECTION ( 'NONE',  ( 0.000000000000000000, 1.000000000000000000, 0.000000000000000000 ) ) ;
#1078=CARTESIAN_POINT ( 'NONE',  ( -242.9854649072008783, -7.295305384121596681, 9.211094754432867404 ) ) ;
#1080=FACE_BOUND ( 'NONE', #12639, .T. ) ;
#1082=DIRECTION ( 'NONE',  ( 0.000000000000000000, 1.000000000000000000, 0.000000000000000000 ) ) ;
#1083=EDGE_LOOP ( 'NONE', ( #9380, #8970, #4045, #3801 ) ) ;
#1084=ORIENTED_EDGE ( 'NONE', *, *, #1420, .T. ) ;
#1085=EDGE_CURVE ( 'NONE', #5993, #10156, #1895, .T. ) ;
#1088=CARTESIAN_POINT ( 'NONE',  ( 122.2593324768346008, 29.00000000000000000, 168.2755348299889988 ) ) ;
#1090=CIRCLE ( 'NONE', #4284, 249.7999999999999829 ) ;
#1091=CIRCLE ( 'NONE', #7432, 5.500000000000005329 ) ;
#1094=CARTESIAN_POINT ( 'NONE',  ( -243.8684449385701498, 8.017730970305375848, 8.590997659349747906 ) ) ;
#1099=DIRECTION ( 'NONE',  ( 0.000000000000000000, 1.000000000000000000, 0.000000000000000000 ) ) ;
#1103=ADVANCED_FACE ( 'NONE', ( #5357 ), #6495, .F. ) ;
#1111=DIRECTION ( 'NONE',  ( 0.000000000000000000, 1.000000000000000000, 0.000000000000000000 ) ) ;
#1116=AXIS2_PLACEMENT_3D ( 'NONE', #8493, #3406, #7418 ) ;
#1117=EDGE_LOOP ( 'NONE', ( #10369, #10140, #8988, #2393 ) ) ;
#1126=CARTESIAN_POINT ( 'NONE',  ( -242.2132964870661453, -6.511711374284875120, -9.780601349847026782 ) ) ;
#1128=CARTESIAN_POINT ( 'NONE',  ( -210.0000000000000000, 28.60000000000000142, 5.100000000000000533 ) ) ;
#1131=VECTOR ( 'NONE', #10947, 1000.000000000000000 ) ;
#1134=CONICAL_SURFACE ( 'NONE', #2404, 6.499999999999999112, 0.7853981633974476129 ) ;
#1136=ORIENTED_EDGE ( 'NONE', *, *, #7872, .T. ) ;
#1142=DIRECTION ( 'NONE',  ( 0.000000000000000000, -1.000000000000000000, 0.000000000000000000 ) ) ;
#1145=FACE_OUTER_BOUND ( 'NONE', #9493, .T. ) ;
#1147=CARTESIAN_POINT ( 'NONE',  ( -242.4218346680387697, -6.744440866289951764, 9.622654848396397398 ) ) ;
#1151=CARTESIAN_POINT ( 'NONE',  ( 240.6264023546199553, -3.484414313218967774, 0.3842028182350827881 ) ) ;
#1152=CARTESIAN_POINT ( 'NONE',  ( 229.9831877374639646, -2.133736550081812844, 2.783791508809775550 ) ) ;
#1157=CIRCLE ( 'NONE', #6908, 2.000000000000001776 ) ;
#1158=DIRECTION ( 'NONE',  ( 0.000000000000000000, 1.000000000000000000, 0.000000000000000000 ) ) ;
#1163=CARTESIAN_POINT ( 'NONE',  ( -241.0949697661349376, 4.988078589341720992, 10.64105268566328100 ) ) ;
#1165=EDGE_CURVE ( 'NONE', #5784, #12886, #861, .T. ) ;
#1167=CIRCLE ( 'NONE', #2642, 249.2999999999999829 ) ;
#1168=ORIENTED_EDGE ( 'NONE', *, *, #10750, .F. ) ;
#1172=VERTEX_POINT ( 'NONE', #10057 ) ;
#1173=ORIENTED_EDGE ( 'NONE', *, *, #3195, .F. ) ;
#1174=CONICAL_SURFACE ( 'NONE', #11826, 196.0000000000000000, 0.7853981633974758125 ) ;
#1178=CARTESIAN_POINT ( 'NONE',  ( 239.4581646394653944, 1.471889791882278198, 3.175461175233341926 ) ) ;
#1179=DIRECTION ( 'NONE',  ( 0.000000000000000000, 1.000000000000000000, 0.000000000000000000 ) ) ;
#1183=EDGE_CURVE ( 'NONE', #8254, #10706, #5194, .T. ) ;
#1185=VERTEX_POINT ( 'NONE', #8396 ) ;
#1191=DIRECTION ( 'NONE',  ( 0.000000000000000000, 1.000000000000000000, 0.000000000000000000 ) ) ;
#1192=CARTESIAN_POINT ( 'NONE',  ( -249.6835501129397983, -11.19967427123757453, 3.553901704592668853 ) ) ;
#1197=CARTESIAN_POINT ( 'NONE',  ( -246.2885828969133684, -9.329251179348061029, -7.144935779693829758 ) ) ;
#1202=CARTESIAN_POINT ( 'NONE',  ( 240.6009466513641541, 3.417710891856967859, -0.7616916529149476700 ) ) ;
#1204=ORIENTED_EDGE ( 'NONE', *, *, #8795, .F. ) ;
#1206=DIRECTION ( 'NONE',  ( 0.000000000000000000, 1.000000000000000000, 0.000000000000000000 ) ) ;
#1207=CARTESIAN_POINT ( 'NONE',  ( -249.6746543471935809, 11.17527903294265279, 3.629830555898323929 ) ) ;
#1209=CARTESIAN_POINT ( 'NONE',  ( 0.000000000000000000, 0.000000000000000000, 0.000000000000000000 ) ) ;
#1213=FACE_OUTER_BOUND ( 'NONE', #9627, .T. ) ;
#1215=ORIENTED_EDGE ( 'NONE', *, *, #6502, .F. ) ;
#1217=CARTESIAN_POINT ( 'NONE',  ( 229.9799928493307846, -1.755858631984955398, -3.036273278599403103 ) ) ;
#1219=ORIENTED_EDGE ( 'NONE', *, *, #10968, .T. ) ;
#1220=CARTESIAN_POINT ( 'NONE',  ( 240.2701176883056178, -2.464548987107058942, 2.493043655918042667 ) ) ;
#1226=CARTESIAN_POINT ( 'NONE',  ( -240.1208361041844910, 2.772967769358974710, 11.41810622433049893 ) ) ;
#1227=EDGE_CURVE ( 'NONE', #6293, #12220, #7581, .T. ) ;
#1229=EDGE_LOOP ( 'NONE', ( #13019, #234 ) ) ;
#1232=CARTESIAN_POINT ( 'NONE',  ( 0.000000000000000000, -2.772967769359314882, -240.3921568627448551 ) ) ;
#1235=( GEOMETRIC_REPRESENTATION_CONTEXT ( 3 ) GLOBAL_UNCERTAINTY_ASSIGNED_CONTEXT ( ( #7985 ) ) GLOBAL_UNIT_ASSIGNED_CONTEXT ( ( #9750, #8765, #5565 ) ) REPRESENTATION_CONTEXT ( 'NONE', 'WORKASPACE' ) );
#1241=DIRECTION ( 'NONE',  ( 0.000000000000000000, 0.000000000000000000, 1.000000000000000000 ) ) ;
#1245=CARTESIAN_POINT ( 'NONE',  ( 71.82423009839129691, 28.60000000000000142, -197.3354503650404865 ) ) ;
#1253=VECTOR ( 'NONE', #12788, 1000.000000000000000 ) ;
#1259=CARTESIAN_POINT ( 'NONE',  ( -244.2871807278710889, -8.304201005131382374, -8.312831358495099465 ) ) ;
#1261=VECTOR ( 'NONE', #7857, 1000.000000000000000 ) ;
#1267=DIRECTION ( 'NONE',  ( 0.000000000000000000, -1.000000000000000000, 0.000000000000000000 ) ) ;
#1270=EDGE_CURVE ( 'NONE', #7994, #1045, #2778, .T. ) ;
#1271=DIRECTION ( 'NONE',  ( 0.000000000000000000, 0.000000000000000000, -1.000000000000000000 ) ) ;
#1276=AXIS2_PLACEMENT_3D ( 'NONE', #2445, #9456, #4381 ) ;
#1278=DIRECTION ( 'NONE',  ( 0.000000000000000000, 0.000000000000000000, 1.000000000000000000 ) ) ;
#1283=CARTESIAN_POINT ( 'NONE',  ( 71.82423009839129691, 18.00000000000000000, -197.3354503650404865 ) ) ;
#1286=CARTESIAN_POINT ( 'NONE',  ( 230.0000012283371973, -3.500080719304503596, -0.2270454585753299837 ) ) ;
#1288=EDGE_LOOP ( 'NONE', ( #7427, #8375, #2289, #5621 ) ) ;
#1291=AXIS2_PLACEMENT_3D ( 'NONE', #4047, #3040, #8259 ) ;
#1295=LINE ( 'NONE', #4355, #1995 ) ;
#1297=ORIENTED_EDGE ( 'NONE', *, *, #6841, .F. ) ;
#1298=CARTESIAN_POINT ( 'NONE',  ( 0.000000000000000000, 11.79660968244690089, 247.7999999999999829 ) ) ;
#1299=ORIENTED_EDGE ( 'NONE', *, *, #201, .F. ) ;
#1305=VECTOR ( 'NONE', #8021, 1000.000000000000000 ) ;
#1308=CARTESIAN_POINT ( 'NONE',  ( -239.2756820386164804, 1.575831832474349437, -11.64383448413514976 ) ) ;
#1320=ORIENTED_EDGE ( 'NONE', *, *, #10196, .T. ) ;
#1326=CIRCLE ( 'NONE', #9834, 5.500000000000005329 ) ;
#1332=DIRECTION ( 'NONE',  ( 0.000000000000000000, 1.000000000000000000, 0.000000000000000000 ) ) ;
#1335=DIRECTION ( 'NONE',  ( 0.000000000000000000, 0.000000000000000000, 1.000000000000000000 ) ) ;
#1336=CARTESIAN_POINT ( 'NONE',  ( 71.82423009839129691, 30.00000000000000000, -202.4354503650404808 ) ) ;
#1339=DIRECTION ( 'NONE',  ( 0.000000000000000000, 0.000000000000000000, -1.000000000000000000 ) ) ;
#1340=DIRECTION ( 'NONE',  ( 0.000000000000000000, -1.000000000000000000, 0.000000000000000000 ) ) ;
#1343=ADVANCED_FACE ( 'NONE', ( #3765 ), #8341, .F. ) ;
#1349=CARTESIAN_POINT ( 'NONE',  ( 240.5727840947570826, -3.342302961263916572, 1.043131940311951888 ) ) ;
#1351=ORIENTED_EDGE ( 'NONE', *, *, #7739, .F. ) ;
#1354=CARTESIAN_POINT ( 'NONE',  ( 240.1689872792144627, -2.295088600365091214, 2.642490611637378972 ) ) ;
#1355=CARTESIAN_POINT ( 'NONE',  ( 197.8197553893915028, 30.00000000000000000, -64.27553482998990830 ) ) ;
#1356=CONICAL_SURFACE ( 'NONE', #4960, 6.499999999999999112, 0.7853981633974476129 ) ;
#1357=AXIS2_PLACEMENT_3D ( 'NONE', #1245, #5311, #10510 ) ;
#1361=CARTESIAN_POINT ( 'NONE',  ( 2.388061258337338860E-14, 0.000000000000000000, 195.0000000000000000 ) ) ;
#1364=ORIENTED_EDGE ( 'NONE', *, *, #10626, .T. ) ;
#1366=CIRCLE ( 'NONE', #2001, 2.000000000000001776 ) ;
#1367=ORIENTED_EDGE ( 'NONE', *, *, #1628, .F. ) ;
#1368=CARTESIAN_POINT ( 'NONE',  ( -248.0831933713610056, -9.830508068705260172, -6.436117704883899115 ) ) ;
#1369=ORIENTED_EDGE ( 'NONE', *, *, #2578, .T. ) ;
#1370=VERTEX_POINT ( 'NONE', #8711 ) ;
#1374=CARTESIAN_POINT ( 'NONE',  ( 0.000000000000000000, 19.00000000000000000, -208.0000000000000000 ) ) ;
#1375=CONICAL_SURFACE ( 'NONE', #4547, 249.7999999999999829, 0.7853981633975309906 ) ;
#1376=CARTESIAN_POINT ( 'NONE',  ( -239.2239425775430561, 1.510213393934768833, -11.65254303168215522 ) ) ;
#1380=EDGE_LOOP ( 'NONE', ( #12699, #5639, #6225, #9706 ) ) ;
#1383=CARTESIAN_POINT ( 'NONE',  ( 0.000000000000000000, 0.000000000000000000, -195.0000000000000000 ) ) ;
#1385=AXIS2_PLACEMENT_3D ( 'NONE', #2580, #5716, #2641 ) ;
#1389=CARTESIAN_POINT ( 'NONE',  ( 0.000000000000000000, 18.00000000000000000, 208.0000000000000000 ) ) ;
#1390=CARTESIAN_POINT ( 'NONE',  ( -239.5361044668159991, -1.848645179572815156, -11.60366368868215758 ) ) ;
#1391=AXIS2_PLACEMENT_3D ( 'NONE', #6939, #11192, #2057 ) ;
#1392=LINE ( 'NONE', #8528, #8634 ) ;
#1395=CIRCLE ( 'NONE', #9275, 245.7999999999999829 ) ;
#1396=EDGE_CURVE ( 'NONE', #9887, #982, #5515, .T. ) ;
#1401=VERTEX_POINT ( 'NONE', #9042 ) ;
#1404=DIRECTION ( 'NONE',  ( 0.000000000000000000, -1.000000000000000000, 0.000000000000000000 ) ) ;
#1407=FACE_OUTER_BOUND ( 'NONE', #12837, .T. ) ;
#1411=CARTESIAN_POINT ( 'NONE',  ( -246.1720478449190637, -9.282004955874285201, 7.205195110361622746 ) ) ;
#1414=DIRECTION ( 'NONE',  ( 8.659560562354926695E-17, 0.7071067811865480168, -0.7071067811865470176 ) ) ;
#1417=LINE ( 'NONE', #12611, #8489 ) ;
#1419=EDGE_CURVE ( 'NONE', #10498, #2672, #1090, .T. ) ;
#1420=EDGE_CURVE ( 'NONE', #2835, #10938, #4844, .T. ) ;
#1422=DIRECTION ( 'NONE',  ( 0.000000000000000000, 0.000000000000000000, -1.000000000000000000 ) ) ;
#1424=CARTESIAN_POINT ( 'NONE',  ( -240.8352866734745419, 4.521734055696428278, 10.84609021980019250 ) ) ;
#1426=ORIENTED_EDGE ( 'NONE', *, *, #3118, .T. ) ;
#1428=ORIENTED_EDGE ( 'NONE', *, *, #4125, .T. ) ;
#1430=FACE_OUTER_BOUND ( 'NONE', #10359, .T. ) ;
#1432=VERTEX_POINT ( 'NONE', #6975 ) ;
#1435=CARTESIAN_POINT ( 'NONE',  ( -210.0000000000000000, 30.00000000000000000, 6.500000000000000000 ) ) ;
#1438=DIRECTION ( 'NONE',  ( 0.000000000000000000, -1.000000000000000000, 0.000000000000000000 ) ) ;
#1442=CARTESIAN_POINT ( 'NONE',  ( 71.82423009839129691, 19.40000000000000213, -197.3354503650404865 ) ) ;
#1443=VECTOR ( 'NONE', #8797, 1000.000000000000000 ) ;
#1444=ORIENTED_EDGE ( 'NONE', *, *, #4920, .T. ) ;
#1445=CARTESIAN_POINT ( 'NONE',  ( 0.000000000000000000, 0.000000000000000000, -230.0000000000000000 ) ) ;
#1448=DIRECTION ( 'NONE',  ( 0.000000000000000000, 0.000000000000000000, 1.000000000000000000 ) ) ;
#1450=CARTESIAN_POINT ( 'NONE',  ( -229.7744328040709263, 5.870883422401756313, 10.18542137201373166 ) ) ;
#1455=AXIS2_PLACEMENT_3D ( 'NONE', #2024, #7289, #3140 ) ;
#1458=AXIS2_PLACEMENT_3D ( 'NONE', #11202, #7145, #2922 ) ;
#1460=DIRECTION ( 'NONE',  ( 0.000000000000000000, -1.000000000000000000, 0.000000000000000000 ) ) ;
#1462=VERTEX_POINT ( 'NONE', #3835 ) ;
#1464=DIRECTION ( 'NONE',  ( 0.000000000000000000, 0.000000000000000000, 1.000000000000000000 ) ) ;
#1466=EDGE_CURVE ( 'NONE', #4307, #889, #11101, .T. ) ;
#1467=FACE_OUTER_BOUND ( 'NONE', #967, .T. ) ;
#1468=CARTESIAN_POINT ( 'NONE',  ( 0.000000000000000000, 0.000000000000000000, 3.499999999999964917 ) ) ;
#1469=VECTOR ( 'NONE', #10856, 1000.000000000000000 ) ;
#1472=CARTESIAN_POINT ( 'NONE',  ( -229.6996680450365034, 7.200459016985159977E-17, -11.75000000000000000 ) ) ;
#1473=AXIS2_PLACEMENT_3D ( 'NONE', #5369, #5234, #10298 ) ;
#1475=CIRCLE ( 'NONE', #3813, 5.500000000000005329 ) ;
#1477=CARTESIAN_POINT ( 'NONE',  ( 0.000000000000000000, 25.00000000000000000, 0.000000000000000000 ) ) ;
#1478=ORIENTED_EDGE ( 'NONE', *, *, #3171, .F. ) ;
#1479=ORIENTED_EDGE ( 'NONE', *, *, #5493, .F. ) ;
#1480=CIRCLE ( 'NONE', #2326, 2.500000000000002220 ) ;
#1481=DIRECTION ( 'NONE',  ( 0.000000000000000000, 1.000000000000000000, 0.000000000000000000 ) ) ;
#1482=FACE_OUTER_BOUND ( 'NONE', #7898, .T. ) ;
#1483=EDGE_CURVE ( 'NONE', #10156, #5993, #12381, .T. ) ;
#1485=DIRECTION ( 'NONE',  ( 0.000000000000000000, 0.000000000000000000, -1.000000000000000000 ) ) ;
#1487=FACE_OUTER_BOUND ( 'NONE', #6503, .T. ) ;
#1490=ORIENTED_EDGE ( 'NONE', *, *, #4901, .F. ) ;
#1491=CARTESIAN_POINT ( 'NONE',  ( -245.7999999999999829, 25.00000000000000000, 0.000000000000000000 ) ) ;
#1492=EDGE_CURVE ( 'NONE', #13031, #5207, #5774, .T. ) ;
#1497=EDGE_LOOP ( 'NONE', ( #1168, #4643, #11486, #3417 ) ) ;
#1498=DIRECTION ( 'NONE',  ( 0.000000000000000000, 0.000000000000000000, 1.000000000000000000 ) ) ;
#1500=CARTESIAN_POINT ( 'NONE',  ( 239.5749691958646963, 1.619550704603064384, -3.102778355204328875 ) ) ;
#1502=CARTESIAN_POINT ( 'NONE',  ( -239.0190616670419672, 1.196899100009489958, -11.68891583568077763 ) ) ;
#1503=DIRECTION ( 'NONE',  ( 0.000000000000000000, 1.000000000000000000, 0.000000000000000000 ) ) ;
#1504=AXIS2_PLACEMENT_3D ( 'NONE', #5276, #10479, #6351 ) ;
#1505=VERTEX_POINT ( 'NONE', #7043 ) ;
#1510=EDGE_CURVE ( 'NONE', #10886, #4193, #11315, .T. ) ;
#1511=CARTESIAN_POINT ( 'NONE',  ( -242.2606306443440758, 6.568547307491611420, -9.743049585709520954 ) ) ;
#1512=DIRECTION ( 'NONE',  ( 0.000000000000000000, 1.000000000000000000, 0.000000000000000000 ) ) ;
#1514=EDGE_CURVE ( 'NONE', #1648, #171, #11908, .T. ) ;
#1517=CARTESIAN_POINT ( 'NONE',  ( -240.6986105848272359, -4.249529545660171159, -10.95469206485073421 ) ) ;
#1527=DIRECTION ( 'NONE',  ( 0.000000000000000000, 0.000000000000000000, -1.000000000000000000 ) ) ;
#1528=ORIENTED_EDGE ( 'NONE', *, *, #7224, .T. ) ;
#1530=DIRECTION ( 'NONE',  ( 0.000000000000000000, 1.000000000000000000, 0.000000000000000000 ) ) ;
#1533=CIRCLE ( 'NONE', #7915, 230.0000000000000000 ) ;
#1535=FACE_BOUND ( 'NONE', #1229, .T. ) ;
#1538=CARTESIAN_POINT ( 'NONE',  ( -229.7304253443789435, -3.777178360538905544, -11.13302378334960885 ) ) ;
#1542=CARTESIAN_POINT ( 'NONE',  ( 7.960204194457795477E-16, 30.00000000000000000, 201.4999999999999716 ) ) ;
#1543=AXIS2_PLACEMENT_3D ( 'NONE', #6251, #121, #1241 ) ;
#1544=ORIENTED_EDGE ( 'NONE', *, *, #3118, .F. ) ;
#1545=ORIENTED_EDGE ( 'NONE', *, *, #11108, .T. ) ;
#1549=CIRCLE ( 'NONE', #6881, 248.7999999999999829 ) ;
#1553=AXIS2_PLACEMENT_3D ( 'NONE', #8451, #1503, #4561 ) ;
#1556=ORIENTED_EDGE ( 'NONE', *, *, #6654, .F. ) ;
#1557=EDGE_CURVE ( 'NONE', #12455, #789, #9358, .T. ) ;
#1560=ORIENTED_EDGE ( 'NONE', *, *, #2957, .F. ) ;
#1565=VECTOR ( 'NONE', #3299, 1000.000000000000000 ) ;
#1566=ORIENTED_EDGE ( 'NONE', *, *, #7009, .F. ) ;
#1567=AXIS2_PLACEMENT_3D ( 'NONE', #5618, #8750, #2731 ) ;
#1571=EDGE_CURVE ( 'NONE', #10870, #1370, #4875, .T. ) ;
#1575=AXIS2_PLACEMENT_3D ( 'NONE', #1298, #11430, #3150 ) ;
#1578=CARTESIAN_POINT ( 'NONE',  ( -238.7807274243665461, -0.5894492284128681758, 11.73530801150233316 ) ) ;
#1580=CARTESIAN_POINT ( 'NONE',  ( -244.2185274279607938, 8.258776625958384798, -8.357937759674365807 ) ) ;
#1582=VECTOR ( 'NONE', #7908, 1000.000000000000000 ) ;
#1583=DIRECTION ( 'NONE',  ( 0.000000000000000000, 0.000000000000000000, -1.000000000000000000 ) ) ;
#1585=DIRECTION ( 'NONE',  ( 0.000000000000000000, 0.000000000000000000, -1.000000000000000000 ) ) ;
#1587=CARTESIAN_POINT ( 'NONE',  ( -229.8981953685927806, 9.554487809903291051, 6.849951329038304948 ) ) ;
#1588=ADVANCED_FACE ( 'NONE', ( #9441 ), #4657, .F. ) ;
#1592=DIRECTION ( 'NONE',  ( 0.000000000000000000, 0.000000000000000000, 1.000000000000000000 ) ) ;
#1593=AXIS2_PLACEMENT_3D ( 'NONE', #9413, #8353, #4338 ) ;
#1595=ORIENTED_EDGE ( 'NONE', *, *, #3607, .T. ) ;
#1596=CARTESIAN_POINT ( 'NONE',  ( -249.7276455222450693, -11.33491751920159452, -3.110604573866400102 ) ) ;
#1599=CARTESIAN_POINT ( 'NONE',  ( 0.000000000000000000, 30.00000000000000000, 0.000000000000000000 ) ) ;
#1600=DIRECTION ( 'NONE',  ( 0.000000000000000000, 1.000000000000000000, 0.000000000000000000 ) ) ;
#1607=CARTESIAN_POINT ( 'NONE',  ( 229.9849294743239625, 2.311676612556695876, -2.637842061394937598 ) ) ;
#1608=CARTESIAN_POINT ( 'NONE',  ( -248.9237871407440252, 10.19078078260020170, -5.849051582844395192 ) ) ;
#1612=DIRECTION ( 'NONE',  ( 0.000000000000000000, 0.000000000000000000, -1.000000000000000000 ) ) ;
#1614=VERTEX_POINT ( 'NONE', #12499 ) ;
#1617=CARTESIAN_POINT ( 'NONE',  ( -210.0000000000000000, 18.00000000000000000, 0.000000000000000000 ) ) ;
#1620=ORIENTED_EDGE ( 'NONE', *, *, #8210, .F. ) ;
#1623=EDGE_LOOP ( 'NONE', ( #874, #501, #6489, #6780 ) ) ;
#1625=ORIENTED_EDGE ( 'NONE', *, *, #1483, .T. ) ;
#1626=CARTESIAN_POINT ( 'NONE',  ( 0.000000000000000000, 25.00000000000000000, 0.000000000000000000 ) ) ;
#1627=CARTESIAN_POINT ( 'NONE',  ( 0.000000000000000000, 18.00000000000000000, -196.0000000000000000 ) ) ;
#1628=EDGE_CURVE ( 'NONE', #6909, #12286, #12124, .T. ) ;
#1629=ADVANCED_FACE ( 'NONE', ( #8380, #12440, #3290, #7373, #91, #10207, #11148, #10141, #817, #1080, #4078, #8751, #8088, #13017, #6024 ), #9022, .F. ) ;
#1631=CARTESIAN_POINT ( 'NONE',  ( -197.8197553893924976, 30.00000000000000000, -57.77553482998720114 ) ) ;
#1632=DIRECTION ( 'NONE',  ( 0.000000000000000000, 0.000000000000000000, 1.000000000000000000 ) ) ;
#1635=VERTEX_POINT ( 'NONE', #6954 ) ;
#1637=CARTESIAN_POINT ( 'NONE',  ( -241.3417439075342656, 5.375691555194026527, -10.44818116087475879 ) ) ;
#1642=CARTESIAN_POINT ( 'NONE',  ( 0.000000000000000000, -19.00000000000000000, 0.000000000000000000 ) ) ;
#1645=AXIS2_PLACEMENT_3D ( 'NONE', #2829, #7776, #7980 ) ;
#1646=CARTESIAN_POINT ( 'NONE',  ( -210.0000000000000000, 19.40000000000000213, 5.100000000000000533 ) ) ;
#1648=VERTEX_POINT ( 'NONE', #5141 ) ;
#1655=CARTESIAN_POINT ( 'NONE',  ( -249.7806011017298715, -11.58204051041879801, -1.980500725180536659 ) ) ;
#1665=CARTESIAN_POINT ( 'NONE',  ( -229.9415104875559734, -10.54483369259275349, -5.197775207300905365 ) ) ;
#1668=CARTESIAN_POINT ( 'NONE',  ( -248.8244828231558472, 10.12360735459614602, -5.964490512238578290 ) ) ;
#1669=DIRECTION ( 'NONE',  ( 0.000000000000000000, 0.000000000000000000, -1.000000000000000000 ) ) ;
#1670=EDGE_CURVE ( 'NONE', #2427, #8254, #1884, .T. ) ;
#1674=CARTESIAN_POINT ( 'NONE',  ( 0.000000000000000000, 30.00000000000000000, -202.4999999999999716 ) ) ;
#1676=AXIS2_PLACEMENT_3D ( 'NONE', #6963, #8111, #8096 ) ;
#1678=EDGE_CURVE ( 'NONE', #10191, #5629, #203, .T. ) ;
#1682=AXIS2_PLACEMENT_3D ( 'NONE', #4014, #6899, #9951 ) ;
#1683=CARTESIAN_POINT ( 'NONE',  ( -240.0143494547951377, -2.418590316237056115, -11.50416929261772303 ) ) ;
#1686=CARTESIAN_POINT ( 'NONE',  ( 240.1560849993289537, 2.274296953688199618, -2.660406300278597591 ) ) ;
#1687=CONICAL_SURFACE ( 'NONE', #7433, 6.500000000000005329, 0.7853981633974476129 ) ;
#1688=EDGE_LOOP ( 'NONE', ( #1790, #6635, #590, #6451, #1919, #7286 ) ) ;
#1690=DIRECTION ( 'NONE',  ( 0.000000000000000000, 1.000000000000000000, 0.000000000000000000 ) ) ;
#1694=ORIENTED_EDGE ( 'NONE', *, *, #2415, .F. ) ;
#1697=CARTESIAN_POINT ( 'NONE',  ( 238.9791647118778144, -0.1781744853868436618, -3.496576182273237077 ) ) ;
#1699=TOROIDAL_SURFACE ( 'NONE', #12760, 250.0000000000000000, 10.00000000000000000 ) ;
#1701=CARTESIAN_POINT ( 'NONE',  ( -247.9656915555145815, 9.808762669553802382, 6.469331566347206852 ) ) ;
#1704=CARTESIAN_POINT ( 'NONE',  ( 3.056106087272219914E-14, 25.00000000000000000, -249.2999999999999829 ) ) ;
#1706=CARTESIAN_POINT ( 'NONE',  ( -243.1580368188211310, 7.448595192303357315, -9.087405006429683851 ) ) ;
#1707=VERTEX_POINT ( 'NONE', #5956 ) ;
#1708=EDGE_CURVE ( 'NONE', #497, #7072, #7645, .T. ) ;
#1714=CARTESIAN_POINT ( 'NONE',  ( -229.8895716818989285, 9.351917924694065576, -7.154906690919313306 ) ) ;
#1715=VECTOR ( 'NONE', #9476, 1000.000000000000114 ) ;
#1720=DIRECTION ( 'NONE',  ( 0.000000000000000000, 0.000000000000000000, 1.000000000000000000 ) ) ;
#1724=EDGE_CURVE ( 'NONE', #497, #1707, #4946, .T. ) ;
#1726=CARTESIAN_POINT ( 'NONE',  ( -249.4468820693415410, -10.72473316041474334, -4.809560399683298293 ) ) ;
#1727=EDGE_LOOP ( 'NONE', ( #12687, #9600, #8517, #4341 ) ) ;
#1729=CARTESIAN_POINT ( 'NONE',  ( -210.0000000000000000, 19.40000000000000213, 0.000000000000000000 ) ) ;
#1732=AXIS2_PLACEMENT_3D ( 'NONE', #4628, #9767, #1448 ) ;
#1738=CARTESIAN_POINT ( 'NONE',  ( 229.9733680233430277, 0.4624089970348260192, 3.499999999999964917 ) ) ;
#1739=VECTOR ( 'NONE', #3289, 1000.000000000000000 ) ;
#1740=CARTESIAN_POINT ( 'NONE',  ( -249.7266004383521079, 11.33448610545603685, -3.100135285984364053 ) ) ;
#1742=EDGE_CURVE ( 'NONE', #1954, #10191, #6558, .T. ) ;
#1744=ORIENTED_EDGE ( 'NONE', *, *, #7425, .F. ) ;
#1746=DIRECTION ( 'NONE',  ( 8.659560562354963673E-17, 0.7071067811865450192, -0.7071067811865500152 ) ) ;
#1750=EDGE_CURVE ( 'NONE', #1635, #12270, #7019, .T. ) ;
#1753=DIRECTION ( 'NONE',  ( 0.000000000000000000, 0.000000000000000000, 1.000000000000000000 ) ) ;
#1757=CIRCLE ( 'NONE', #1543, 5.500000000000005329 ) ;
#1760=VERTEX_POINT ( 'NONE', #7155 ) ;
#1762=CARTESIAN_POINT ( 'NONE',  ( 239.8763759935506528, -1.918973793115196225, 2.928207549569424195 ) ) ;
#1766=CARTESIAN_POINT ( 'NONE',  ( 0.000000000000000000, -20.00000000000000000, 248.7999999999999829 ) ) ;
#1767=AXIS2_PLACEMENT_3D ( 'NONE', #5566, #3355, #7441 ) ;
#1769=EDGE_CURVE ( 'NONE', #9162, #1505, #1905, .T. ) ;
#1770=FACE_OUTER_BOUND ( 'NONE', #2245, .T. ) ;
#1774=CARTESIAN_POINT ( 'NONE',  ( 2.400307726328812059E-14, 18.00000000000000000, 196.0000000000000000 ) ) ;
#1778=CARTESIAN_POINT ( 'NONE',  ( -245.3834146146978981, 8.931379171135056083, -7.634986101342768450 ) ) ;
#1784=CARTESIAN_POINT ( 'NONE',  ( -229.7150392099732414, 2.684421947324201252, -11.44580934118247662 ) ) ;
#1787=VECTOR ( 'NONE', #343, 1000.000000000000000 ) ;
#1790=ORIENTED_EDGE ( 'NONE', *, *, #8838, .F. ) ;
#1791=DIRECTION ( 'NONE',  ( 0.000000000000000000, 1.000000000000000000, 0.000000000000000000 ) ) ;
#1792=ORIENTED_EDGE ( 'NONE', *, *, #6213, .F. ) ;
#1796=CARTESIAN_POINT ( 'NONE',  ( -249.7621493473840815, -11.48044694427989931, -2.508021710844266394 ) ) ;
#1797=ORIENTED_EDGE ( 'NONE', *, *, #7193, .F. ) ;
#1799=CARTESIAN_POINT ( 'NONE',  ( -210.0000000000000000, 30.00000000000000000, 0.000000000000000000 ) ) ;
#1802=CARTESIAN_POINT ( 'NONE',  ( -197.8197553893909912, 29.00000000000000000, 64.27553482999130097 ) ) ;
#1804=FACE_OUTER_BOUND ( 'NONE', #7248, .T. ) ;
#1805=EDGE_CURVE ( 'NONE', #1707, #6121, #10843, .T. ) ;
#1806=AXIS2_PLACEMENT_3D ( 'NONE', #5372, #510, #8449 ) ;
#1809=CARTESIAN_POINT ( 'NONE',  ( -229.7747724777948122, -5.884216672786659608, 10.17777400990889447 ) ) ;
#1812=CARTESIAN_POINT ( 'NONE',  ( -249.7095932329616517, 11.27773618852464743, -3.298468580809413186 ) ) ;
#1814=ORIENTED_EDGE ( 'NONE', *, *, #9154, .F. ) ;
#1818=FACE_OUTER_BOUND ( 'NONE', #12368, .T. ) ;
#1821=ORIENTED_EDGE ( 'NONE', *, *, #5754, .F. ) ;
#1822=AXIS2_PLACEMENT_3D ( 'NONE', #11165, #6104, #10155 ) ;
#1823=DIRECTION ( 'NONE',  ( 1.000000000000000000, -0.000000000000000000, 1.224646799147353207E-16 ) ) ;
#1826=ORIENTED_EDGE ( 'NONE', *, *, #428, .F. ) ;
#1829=EDGE_CURVE ( 'NONE', #3502, #1020, #7408, .T. ) ;
#1830=DIRECTION ( 'NONE',  ( 0.000000000000000000, 0.000000000000000000, 1.000000000000000000 ) ) ;
#1833=CARTESIAN_POINT ( 'NONE',  ( 71.82423009839129691, 30.00000000000000000, -197.3354503650404865 ) ) ;
#1837=DIRECTION ( 'NONE',  ( 0.000000000000000000, 1.000000000000000000, 0.000000000000000000 ) ) ;
#1840=DIRECTION ( 'NONE',  ( 0.000000000000000000, 0.000000000000000000, -1.000000000000000000 ) ) ;
#1842=CARTESIAN_POINT ( 'NONE',  ( -239.0190678720388178, 1.196910331790569160, 11.68891451185957031 ) ) ;
#1843=EDGE_LOOP ( 'NONE', ( #3886, #8579, #654, #10406 ) ) ;
#1844=ADVANCED_FACE ( 'NONE', ( #10276 ), #6418, .F. ) ;
#1846=CARTESIAN_POINT ( 'NONE',  ( 240.2035656452229091, -2.353769564549843984, -2.590352657762025501 ) ) ;
#1850=EDGE_CURVE ( 'NONE', #7200, #2165, #8357, .T. ) ;
#1851=FACE_BOUND ( 'NONE', #4535, .T. ) ;
#1856=CARTESIAN_POINT ( 'NONE',  ( -238.8528738665295350, -0.8456521594436280376, -11.72073125521067638 ) ) ;
#1857=ORIENTED_EDGE ( 'NONE', *, *, #9342, .F. ) ;
#1860=CARTESIAN_POINT ( 'NONE',  ( -249.3654635700585800, -10.61071050137281091, -5.052935793542020271 ) ) ;
#1861=ORIENTED_EDGE ( 'NONE', *, *, #9054, .F. ) ;
#1863=CARTESIAN_POINT ( 'NONE',  ( -210.0000000000000000, 19.40000000000000213, 0.000000000000000000 ) ) ;
#1864=CARTESIAN_POINT ( 'NONE',  ( 0.000000000000000000, 18.00000000000000000, -208.0000000000000000 ) ) ;
#1874=EDGE_CURVE ( 'NONE', #2184, #6551, #5763, .T. ) ;
#1877=FACE_OUTER_BOUND ( 'NONE', #6763, .T. ) ;
#1881=CARTESIAN_POINT ( 'NONE',  ( -245.3956592408875395, -8.937419274662552482, 7.627912038472048906 ) ) ;
#1883=ORIENTED_EDGE ( 'NONE', *, *, #7660, .F. ) ;
#1884=LINE ( 'NONE', #3073, #2535 ) ;
#1885=AXIS2_PLACEMENT_3D ( 'NONE', #6029, #5018, #6159 ) ;
#1886=CARTESIAN_POINT ( 'NONE',  ( -122.2593324768321992, 30.00000000000000000, 161.7755348299905052 ) ) ;
#1890=CIRCLE ( 'NONE', #2310, 5.500000000000005329 ) ;
#1891=LINE ( 'NONE', #8094, #8068 ) ;
#1894=CARTESIAN_POINT ( 'NONE',  ( -248.5901226953540402, 9.992747119206066841, 6.181484274903534804 ) ) ;
#1895=CIRCLE ( 'NONE', #7006, 5.100000000000000533 ) ;
#1899=EDGE_CURVE ( 'NONE', #9833, #157, #448, .T. ) ;
#1901=EDGE_CURVE ( 'NONE', #10068, #9249, #11935, .T. ) ;
#1902=ORIENTED_EDGE ( 'NONE', *, *, #2369, .T. ) ;
#1903=DIRECTION ( 'NONE',  ( 0.000000000000000000, 0.000000000000000000, 1.000000000000000000 ) ) ;
#1904=VERTEX_POINT ( 'NONE', #8420 ) ;
#1905=CIRCLE ( 'NONE', #12756, 5.099999999999993427 ) ;
#1906=FACE_OUTER_BOUND ( 'NONE', #640, .T. ) ;
#1907=EDGE_LOOP ( 'NONE', ( #12689, #8704, #2989, #589 ) ) ;
#1908=CONICAL_SURFACE ( 'NONE', #4044, 5.500000000000005329, 0.7853981633974461696 ) ;
#1910=CARTESIAN_POINT ( 'NONE',  ( 240.1928509381578465, 2.335100009138994182, 2.607195044851006394 ) ) ;
#1912=CARTESIAN_POINT ( 'NONE',  ( -229.7584495954988881, 5.207945372205803558, -10.53982534208329191 ) ) ;
#1915=ADVANCED_FACE ( 'NONE', ( #2272 ), #651, .F. ) ;
#1916=EDGE_CURVE ( 'NONE', #5028, #10886, #3317, .T. ) ;
#1919=ORIENTED_EDGE ( 'NONE', *, *, #5637, .F. ) ;
#1920=CARTESIAN_POINT ( 'NONE',  ( -238.9443119694662414, -1.049071734835953063, -11.70307552047284894 ) ) ;
#1924=CARTESIAN_POINT ( 'NONE',  ( -248.8393377456389146, -10.13317597119169911, 5.948217566906608411 ) ) ;
#1928=CARTESIAN_POINT ( 'NONE',  ( -197.8197553893924976, 30.00000000000000000, -57.77553482998720114 ) ) ;
#1929=AXIS2_PLACEMENT_3D ( 'NONE', #5537, #8739, #3733 ) ;
#1938=ORIENTED_EDGE ( 'NONE', *, *, #7739, .T. ) ;
#1940=DIRECTION ( 'NONE',  ( 0.000000000000000000, 1.000000000000000000, 0.000000000000000000 ) ) ;
#1942=CARTESIAN_POINT ( 'NONE',  ( 239.1158061866276228, -0.8260238041387650831, -3.401362076983990512 ) ) ;
#1945=CARTESIAN_POINT ( 'NONE',  ( 71.82423009839129691, 28.60000000000000142, -192.2354503650404922 ) ) ;
#1947=CARTESIAN_POINT ( 'NONE',  ( -240.2520669369934865, -3.209691514237213106, 11.31204477728637769 ) ) ;
#1950=ORIENTED_EDGE ( 'NONE', *, *, #1483, .F. ) ;
#1954=VERTEX_POINT ( 'NONE', #675 ) ;
#1956=CARTESIAN_POINT ( 'NONE',  ( 229.9733680233431130, 4.286263893147487610E-16, -3.499999999999964917 ) ) ;
#1957=CARTESIAN_POINT ( 'NONE',  ( -249.6681481789079555, 11.15796663570597147, 3.682817569140960146 ) ) ;
#1962=CARTESIAN_POINT ( 'NONE',  ( -244.0507507057267844, 8.147415050171824547, 8.468315434219642057 ) ) ;
#1964=ADVANCED_FACE ( 'NONE', ( #482 ), #12776, .F. ) ;
#1965=VERTEX_POINT ( 'NONE', #9594 ) ;
#1966=CARTESIAN_POINT ( 'NONE',  ( -122.2593324768321992, 30.00000000000000000, 168.2755348299905052 ) ) ;
#1968=ORIENTED_EDGE ( 'NONE', *, *, #11546, .F. ) ;
#1969=CARTESIAN_POINT ( 'NONE',  ( -245.3661487636251479, 8.922833484245296987, -7.644980496657460378 ) ) ;
#1971=AXIS2_PLACEMENT_3D ( 'NONE', #12742, #8623, #492 ) ;
#1975=DIRECTION ( 'NONE',  ( 0.000000000000000000, 0.000000000000000000, 1.000000000000000000 ) ) ;
#1976=CARTESIAN_POINT ( 'NONE',  ( 239.7985776503625175, 1.848645179571945185, 2.971954070985139751 ) ) ;
#1978=CARTESIAN_POINT ( 'NONE',  ( -197.8197553893909912, 29.00000000000000000, 58.77553482999130807 ) ) ;
#1982=CIRCLE ( 'NONE', #7938, 5.099999999999993427 ) ;
#1986=CARTESIAN_POINT ( 'NONE',  ( -249.2714863791443065, -10.50505558484817925, 5.263680432588698110 ) ) ;
#1987=ORIENTED_EDGE ( 'NONE', *, *, #10581, .F. ) ;
#1990=VECTOR ( 'NONE', #3630, 1000.000000000000000 ) ;
#1992=EDGE_CURVE ( 'NONE', #7634, #12239, #7667, .T. ) ;
#1995=VECTOR ( 'NONE', #3341, 1000.000000000000114 ) ;
#1996=CARTESIAN_POINT ( 'NONE',  ( -244.2512373977512539, -8.280505324001138590, -8.336413190374162951 ) ) ;
#1998=DIRECTION ( 'NONE',  ( 0.000000000000000000, 1.000000000000000000, 0.000000000000000000 ) ) ;
#2000=CARTESIAN_POINT ( 'NONE',  ( -229.6996680450366171, 1.438960022146944131E-15, 11.75000000000000000 ) ) ;
#2001=AXIS2_PLACEMENT_3D ( 'NONE', #7473, #2137, #8220 ) ;
#2002=AXIS2_PLACEMENT_3D ( 'NONE', #4263, #10392, #7336 ) ;
#2003=CARTESIAN_POINT ( 'NONE',  ( -122.2593324768359935, 30.00000000000000000, -168.2755348299880040 ) ) ;
#2007=ADVANCED_FACE ( 'NONE', ( #12729 ), #4054, .T. ) ;
#2012=EDGE_CURVE ( 'NONE', #3737, #7634, #3665, .T. ) ;
#2015=CARTESIAN_POINT ( 'NONE',  ( -243.6657757798965349, -7.864920284775232417, 8.729522416371102267 ) ) ;
#2019=DIRECTION ( 'NONE',  ( 0.000000000000000000, 0.7071067811865480168, 0.7071067811865470176 ) ) ;
#2020=CARTESIAN_POINT ( 'NONE',  ( 229.9973251412452839, -3.320720522893729321, 1.129064247440167756 ) ) ;
#2024=CARTESIAN_POINT ( 'NONE',  ( -197.8197553893909912, 18.00000000000000000, 64.27553482999130097 ) ) ;
#2029=CARTESIAN_POINT ( 'NONE',  ( -247.1459274860969231, 9.611803612594441049, 6.758488905887352516 ) ) ;
#2032=ORIENTED_EDGE ( 'NONE', *, *, #11546, .T. ) ;
#2033=CARTESIAN_POINT ( 'NONE',  ( -246.4294064437368093, 9.379184893845605941, -7.077828147084206378 ) ) ;
#2034=ORIENTED_EDGE ( 'NONE', *, *, #3107, .T. ) ;
#2035=CONICAL_SURFACE ( 'NONE', #4796, 5.499999999999998224, 0.7853981633974461696 ) ;
#2040=CARTESIAN_POINT ( 'NONE',  ( -122.2593324768321992, 30.00000000000000000, 161.7755348299905052 ) ) ;
#2042=DIRECTION ( 'NONE',  ( 0.000000000000000000, 1.000000000000000000, 0.000000000000000000 ) ) ;
#2045=CARTESIAN_POINT ( 'NONE',  ( -238.9359159443557701, -1.030912824209149203, -11.70469086939901437 ) ) ;
#2047=CARTESIAN_POINT ( 'NONE',  ( -249.7854625207512527, 11.61528754085123616, -1.774251673167930754 ) ) ;
#2048=DIRECTION ( 'NONE',  ( 8.659560562354913137E-17, -0.7071067811865489050, 0.7071067811865460184 ) ) ;
#2049=CARTESIAN_POINT ( 'NONE',  ( -249.4806725023741478, -10.78221059150020622, 4.672140297554956412 ) ) ;
#2051=EDGE_CURVE ( 'NONE', #3412, #3020, #8534, .T. ) ;
#2055=CARTESIAN_POINT ( 'NONE',  ( -245.6111173992502756, -9.040876194414714462, -7.505250416031252314 ) ) ;
#2057=DIRECTION ( 'NONE',  ( 0.000000000000000000, 0.000000000000000000, -1.000000000000000000 ) ) ;
#2059=EDGE_CURVE ( 'NONE', #4889, #13031, #7123, .T. ) ;
#2062=ADVANCED_FACE ( 'NONE', ( #6117 ), #2182, .F. ) ;
#2065=ORIENTED_EDGE ( 'NONE', *, *, #8041, .F. ) ;
#2067=DIRECTION ( 'NONE',  ( 0.000000000000000000, 0.000000000000000000, 1.000000000000000000 ) ) ;
#2070=DIRECTION ( 'NONE',  ( 0.000000000000000000, 1.000000000000000000, 0.000000000000000000 ) ) ;
#2072=CARTESIAN_POINT ( 'NONE',  ( -244.0876577941736230, -8.170278132102669844, 8.444514123292313101 ) ) ;
#2074=EDGE_CURVE ( 'NONE', #5784, #10046, #8107, .T. ) ;
#2078=LINE ( 'NONE', #1542, #5506 ) ;
#2080=EDGE_LOOP ( 'NONE', ( #11000, #8423, #6628, #1826 ) ) ;
#2083=CARTESIAN_POINT ( 'NONE',  ( -197.8197553893909912, 30.00000000000000000, 70.77553482999131518 ) ) ;
#2087=CARTESIAN_POINT ( 'NONE',  ( -245.8608051595201403, 9.153297356747751579, 7.368056653819033741 ) ) ;
#2089=CONICAL_SURFACE ( 'NONE', #9340, 249.2999999999999829, 0.7853981633974207455 ) ;
#2090=DIRECTION ( 'NONE',  ( 0.000000000000000000, 1.000000000000000000, 0.000000000000000000 ) ) ;
#2091=CIRCLE ( 'NONE', #9537, 231.0000000000000000 ) ;
#2100=LINE ( 'NONE', #50, #5575 ) ;
#2101=DIRECTION ( 'NONE',  ( 0.000000000000000000, 1.000000000000000000, 0.000000000000000000 ) ) ;
#2102=DIRECTION ( 'NONE',  ( 0.000000000000000000, 0.000000000000000000, 1.000000000000000000 ) ) ;
#2111=CARTESIAN_POINT ( 'NONE',  ( -210.0000000000000000, 28.60000000000000142, 0.000000000000000000 ) ) ;
#2114=CARTESIAN_POINT ( 'NONE',  ( -248.3532242370870620, -9.880481159896127963, 6.359788946042714386 ) ) ;
#2115=ORIENTED_EDGE ( 'NONE', *, *, #11514, .T. ) ;
#2119=CARTESIAN_POINT ( 'NONE',  ( -242.9798744230415934, -7.293926269598956402, -9.214525213004751691 ) ) ;
#2126=CIRCLE ( 'NONE', #5099, 245.7999999999999829 ) ;
#2128=B_SPLINE_CURVE_WITH_KNOTS ( 'NONE', 3,
 ( #7950, #1947, #7151, #8153, #7215, #5067, #12148, #11146, #4066, #10272, #5007, #4003, #6217, #9144, #4075, #3129, #1147, #11281, #3943, #10013, #1078, #8084, #6021, #5136, #9212, #8965, #89, #4143, #20, #12219, #3070, #2015, #12021, #10079, #11208, #2072, #2141, #6150, #2999, #6087, #7082, #10204, #8224, #5953, #2867, #951, #6952, #8952, #13013, #3877, #11008, #1881, #882, #4943, #4272, #1411, #5472, #5273, #10541, #9530, #6416, #9347, #152, #2212, #3394, #7347, #12476 ),
 .UNSPECIFIED., .F., .F.,
 ( 4, 2, 2, 1, 1, 1, 1, 2, 2, 2, 2, 2, 1, 1, 1, 1, 1, 2, 2, 2, 2, 2, 1, 1, 1, 2, 2, 2, 2, 1, 1, 1, 1, 2, 2, 2, 2, 1, 1, 1, 2, 2, 4 ),
 ( 0.000000000000000000, 0.1249999999996426747, 0.1874999999994641231, 0.2187499999993749999, 0.2343749999993287592, 0.2421874999993055833, 0.2460937499992956190, 0.2480468749992907895, 0.2499999999992859601, 0.3749999999989899191, 0.4374999999988398169, 0.4687499999987648214, 0.4843749999987274069, 0.4921874999987085886, 0.4960937499986973198, 0.4980468749986917687, 0.4990234374986870503, 0.4995117187486847743, 0.4999999999986824983, 0.5624999999989823696, 0.5937499999991320276, 0.6093749999992053024, 0.6171874999992403854, 0.6210937499992564836, 0.6230468749992645883, 0.6240234374992686961, 0.6249999999992726929, 0.6874999999994171329, 0.7187499999994895195, 0.7343749999995224931, 0.7421874999995388134, 0.7460937499995505817, 0.7480468749995564659, 0.7490234374995594635, 0.7499999999995624611, 0.8124999999996862510, 0.8437499999997453148, 0.8593749999997780664, 0.8671874999997977174, 0.8710937499998041567, 0.8730468749998074873, 0.8749999999998107070, 1.000000000000000000 ),
 .UNSPECIFIED. ) ;
#2129=DIRECTION ( 'NONE',  ( 0.000000000000000000, 0.000000000000000000, 1.000000000000000000 ) ) ;
#2131=VERTEX_POINT ( 'NONE', #6454 ) ;
#2133=DIRECTION ( 'NONE',  ( 0.000000000000000000, 0.000000000000000000, 1.000000000000000000 ) ) ;
#2135=CARTESIAN_POINT ( 'NONE',  ( 239.1818646735635241, -0.9924701939322742028, -3.356351167340032138 ) ) ;
#2137=DIRECTION ( 'NONE',  ( -1.000000000000000000, 0.000000000000000000, 0.000000000000000000 ) ) ;
#2139=CARTESIAN_POINT ( 'NONE',  ( -210.0000000000000000, 28.60000000000000142, -5.100000000000000533 ) ) ;
#2141=CARTESIAN_POINT ( 'NONE',  ( -244.1571280462642619, -8.217568831514851624, 8.398466974160381682 ) ) ;
#2142=EDGE_LOOP ( 'NONE', ( #6103, #9301, #10192, #11179 ) ) ;
#2143=DIRECTION ( 'NONE',  ( 0.000000000000000000, 1.000000000000000000, 0.000000000000000000 ) ) ;
#2144=CARTESIAN_POINT ( 'NONE',  ( -239.1938262336951482, 1.469859129952955312, 11.65770207320726470 ) ) ;
#2145=CARTESIAN_POINT ( 'NONE',  ( 229.9750439289697113, -0.9060155281103843272, 3.388384136948113579 ) ) ;
#2147=ORIENTED_EDGE ( 'NONE', *, *, #7598, .T. ) ;
#2149=CARTESIAN_POINT ( 'NONE',  ( -249.7999999999999829, 22.00000000000000000, 0.000000000000000000 ) ) ;
#2150=ADVANCED_FACE ( 'NONE', ( #10709 ), #10446, .F. ) ;
#2154=AXIS2_PLACEMENT_3D ( 'NONE', #9103, #9171, #4969 ) ;
#2158=CARTESIAN_POINT ( 'NONE',  ( -241.8928034524436441, 6.135811581234290379, 10.02290695385687158 ) ) ;
#2162=ORIENTED_EDGE ( 'NONE', *, *, #6885, .F. ) ;
#2163=LINE ( 'NONE', #11502, #8842 ) ;
#2165=VERTEX_POINT ( 'NONE', #2505 ) ;
#2166=AXIS2_PLACEMENT_3D ( 'NONE', #10042, #6049, #3228 ) ;
#2170=CARTESIAN_POINT ( 'NONE',  ( 239.1158061866188405, 0.8260238041136663822, 3.401362076984711269 ) ) ;
#2177=DIRECTION ( 'NONE',  ( 0.000000000000000000, 1.000000000000000000, 0.000000000000000000 ) ) ;
#2178=CIRCLE ( 'NONE', #700, 6.500000000000000000 ) ;
#2180=CIRCLE ( 'NONE', #3024, 239.8169934640465044 ) ;
#2181=LINE ( 'NONE', #1383, #11686 ) ;
#2182=CYLINDRICAL_SURFACE ( 'NONE', #12147, 5.499999999999998224 ) ;
#2183=CARTESIAN_POINT ( 'NONE',  ( -248.0831933713610056, -9.830508068705269054, 6.436117704883859147 ) ) ;
#2184=VERTEX_POINT ( 'NONE', #2442 ) ;
#2187=LINE ( 'NONE', #10579, #4236 ) ;
#2189=CARTESIAN_POINT ( 'NONE',  ( -246.7009519929982275, -9.473788075376265994, -6.950529151851262633 ) ) ;
#2191=CARTESIAN_POINT ( 'NONE',  ( 239.1299809605872326, -0.8683754750072776307, 3.391597751362151580 ) ) ;
#2193=CARTESIAN_POINT ( 'NONE',  ( 240.5112511684932883, 3.170498835030340690, 1.486196988727406465 ) ) ;
#2196=CIRCLE ( 'NONE', #7959, 6.500000000000005329 ) ;
#2206=CARTESIAN_POINT ( 'NONE',  ( 239.4370728335728700, -1.442813601772337639, -3.188799201155995355 ) ) ;
#2207=CARTESIAN_POINT ( 'NONE',  ( 71.82423009839129691, 19.40000000000000213, 202.4354503650404808 ) ) ;
#2209=CIRCLE ( 'NONE', #4129, 5.500000000000005329 ) ;
#2212=CARTESIAN_POINT ( 'NONE',  ( -246.6693634554316645, -9.463199073330141431, 6.964939579038730955 ) ) ;
#2213=ORIENTED_EDGE ( 'NONE', *, *, #1419, .F. ) ;
#2214=CARTESIAN_POINT ( 'NONE',  ( 71.82423009839129691, 18.00000000000000000, 197.3354503650404865 ) ) ;
#2215=CARTESIAN_POINT ( 'NONE',  ( 229.9884488601945236, -2.638803137220849138, -2.310864750561204772 ) ) ;
#2219=DIRECTION ( 'NONE',  ( 0.000000000000000000, 0.000000000000000000, 1.000000000000000000 ) ) ;
#2222=DIRECTION ( 'NONE',  ( 0.000000000000000000, 1.000000000000000000, 0.000000000000000000 ) ) ;
#2224=CARTESIAN_POINT ( 'NONE',  ( -244.4357566151503534, 8.400224619627458367, 8.216123740249937413 ) ) ;
#2227=CARTESIAN_POINT ( 'NONE',  ( -210.0000000000000000, 18.00000000000000000, -6.500000000000007994 ) ) ;
#2229=ORIENTED_EDGE ( 'NONE', *, *, #2803, .F. ) ;
#2230=EDGE_CURVE ( 'NONE', #6421, #10706, #10641, .T. ) ;
#2231=DIRECTION ( 'NONE',  ( 0.000000000000000000, 1.000000000000000000, 0.000000000000000000 ) ) ;
#2233=VERTEX_POINT ( 'NONE', #8458 ) ;
#2235=DIRECTION ( 'NONE',  ( 0.000000000000000000, 0.000000000000000000, 1.000000000000000000 ) ) ;
#2239=CARTESIAN_POINT ( 'NONE',  ( 239.4793126112416246, 1.500292816075383895, -3.162144597818810077 ) ) ;
#2243=ORIENTED_EDGE ( 'NONE', *, *, #4967, .F. ) ;
#2245=EDGE_LOOP ( 'NONE', ( #10390, #7652, #3647, #709 ) ) ;
#2247=AXIS2_PLACEMENT_3D ( 'NONE', #8902, #7107, #4825 ) ;
#2255=DIRECTION ( 'NONE',  ( 0.000000000000000000, 0.000000000000000000, 1.000000000000000000 ) ) ;
#2256=CARTESIAN_POINT ( 'NONE',  ( -242.2247058965992608, -6.524571383558081195, -9.772025480106055539 ) ) ;
#2262=CYLINDRICAL_SURFACE ( 'NONE', #10521, 230.0000000000000000 ) ;
#2264=CARTESIAN_POINT ( 'NONE',  ( -248.7900388717503404, 10.10208648674501219, 6.000868149965899789 ) ) ;
#2266=LINE ( 'NONE', #5202, #5199 ) ;
#2268=DIRECTION ( 'NONE',  ( 0.000000000000000000, 1.000000000000000000, 0.000000000000000000 ) ) ;
#2272=FACE_OUTER_BOUND ( 'NONE', #6185, .T. ) ;
#2273=EDGE_CURVE ( 'NONE', #12270, #12220, #5318, .T. ) ;
#2274=CARTESIAN_POINT ( 'NONE',  ( 229.9996516955224877, -3.477323162167160753, -0.4589134507980298650 ) ) ;
#2278=DIRECTION ( 'NONE',  ( 0.000000000000000000, 0.000000000000000000, -1.000000000000000000 ) ) ;
#2285=CARTESIAN_POINT ( 'NONE',  ( 0.000000000000000000, 0.000000000000000000, -11.75000000000000000 ) ) ;
#2286=EDGE_CURVE ( 'NONE', #9966, #4005, #12133, .T. ) ;
#2287=ORIENTED_EDGE ( 'NONE', *, *, #3305, .T. ) ;
#2289=ORIENTED_EDGE ( 'NONE', *, *, #7425, .T. ) ;
#2292=CARTESIAN_POINT ( 'NONE',  ( 122.2593324768346008, 30.00000000000000000, 168.2755348299889988 ) ) ;
#2293=DIRECTION ( 'NONE',  ( 0.000000000000000000, -1.000000000000000000, 0.000000000000000000 ) ) ;
#2295=CARTESIAN_POINT ( 'NONE',  ( 239.4650615381723355, 1.481238645322935588, -3.171113114083459639 ) ) ;
#2296=B_SPLINE_CURVE_WITH_KNOTS ( 'NONE', 3,
 ( #8985, #11943, #10167, #6002, #12117, #3037, #1046, #7120, #7914, #4841, #5037, #6057, #11178, #9985, #4043, #12050, #8920, #1920, #2045, #10984, #1856, #7845, #9917, #11113, #5921, #6985, #5105, #12983, #8119, #2970, #854, #10110 ),
 .UNSPECIFIED., .F., .F.,
 ( 4, 2, 2, 1, 1, 2, 2, 2, 2, 1, 2, 2, 2, 2, 1, 1, 1, 2, 4 ),
 ( 0.000000000000000000, 0.06250953600675514255, 0.09376430401013917393, 0.1093916880118240981, 0.1172053800126664769, 0.1211122260130798878, 0.1250190720134933264, 0.1875286080200248562, 0.2187833760232906488, 0.2344107600249281387, 0.2422244520257468836, 0.2500381440265656563, 0.3750572160396264954, 0.4375667520461548610, 0.4688215200494180168, 0.4844489040510496225, 0.4922625960518653976, 0.4961694420522733129, 0.5000762880526811172 ),
 .UNSPECIFIED. ) ;
#2297=CARTESIAN_POINT ( 'NONE',  ( -239.0839753095793014, 1.310033608828027774, -11.67696114067532775 ) ) ;
#2300=AXIS2_PLACEMENT_3D ( 'NONE', #12226, #4281, #8361 ) ;
#2302=ORIENTED_EDGE ( 'NONE', *, *, #3436, .F. ) ;
#2303=DIRECTION ( 'NONE',  ( 0.000000000000000000, -1.000000000000000000, 0.000000000000000000 ) ) ;
#2309=AXIS2_PLACEMENT_3D ( 'NONE', #10771, #6521, #12769 ) ;
#2310=AXIS2_PLACEMENT_3D ( 'NONE', #9323, #12193, #2980 ) ;
#2313=DIRECTION ( 'NONE',  ( 0.000000000000000000, 1.000000000000000000, 0.000000000000000000 ) ) ;
#2314=CIRCLE ( 'NONE', #11256, 239.8169934640465044 ) ;
#2316=CARTESIAN_POINT ( 'NONE',  ( 71.82423009839129691, 30.00000000000000000, 197.3354503650404865 ) ) ;
#2319=AXIS2_PLACEMENT_3D ( 'NONE', #1799, #8861, #470 ) ;
#2320=CIRCLE ( 'NONE', #2733, 6.500000000000005329 ) ;
#2321=( LENGTH_UNIT ( ) NAMED_UNIT ( * ) SI_UNIT ( .MILLI., .METRE. ) );
#2326=AXIS2_PLACEMENT_3D ( 'NONE', #649, #3571, #4700 ) ;
#2328=DIRECTION ( 'NONE',  ( 0.000000000000000000, 0.000000000000000000, 1.000000000000000000 ) ) ;
#2337=CARTESIAN_POINT ( 'NONE',  ( -210.0000000000000000, 30.00000000000000000, 0.000000000000000000 ) ) ;
#2342=EDGE_LOOP ( 'NONE', ( #8244, #9820 ) ) ;
#2343=CARTESIAN_POINT ( 'NONE',  ( 240.4535390813941831, -3.009067775125233712, 1.828999330899334863 ) ) ;
#2346=CARTESIAN_POINT ( 'NONE',  ( 122.2593324768346008, 30.00000000000000000, 161.7755348299889988 ) ) ;
#2348=ORIENTED_EDGE ( 'NONE', *, *, #12233, .F. ) ;
#2363=ORIENTED_EDGE ( 'NONE', *, *, #5955, .T. ) ;
#2364=ORIENTED_EDGE ( 'NONE', *, *, #10139, .F. ) ;
#2367=CIRCLE ( 'NONE', #11688, 5.500000000000005329 ) ;
#2369=EDGE_CURVE ( 'NONE', #12890, #4958, #2126, .T. ) ;
#2370=EDGE_CURVE ( 'NONE', #3500, #2835, #4666, .T. ) ;
#2375=CARTESIAN_POINT ( 'NONE',  ( 0.000000000000000000, 3.327561323230765034, 0.000000000000000000 ) ) ;
#2379=DIRECTION ( 'NONE',  ( 0.000000000000000000, 0.000000000000000000, 1.000000000000000000 ) ) ;
#2381=ORIENTED_EDGE ( 'NONE', *, *, #4479, .T. ) ;
#2382=DIRECTION ( 'NONE',  ( 0.000000000000000000, -1.000000000000000000, 0.000000000000000000 ) ) ;
#2387=CARTESIAN_POINT ( 'NONE',  ( 239.4650615381681860, -1.481238645317465075, 3.171113114088393026 ) ) ;
#2389=ADVANCED_FACE ( 'NONE', ( #3309 ), #10451, .F. ) ;
#2393=ORIENTED_EDGE ( 'NONE', *, *, #117, .T. ) ;
#2396=DIRECTION ( 'NONE',  ( 0.000000000000000000, 0.000000000000000000, -1.000000000000000000 ) ) ;
#2397=CARTESIAN_POINT ( 'NONE',  ( 197.8197553893915028, 30.00000000000000000, -70.77553482998990830 ) ) ;
#2399=CARTESIAN_POINT ( 'NONE',  ( -197.8197553893909912, 29.00000000000000000, 69.77553482999131518 ) ) ;
#2400=FACE_BOUND ( 'NONE', #7484, .T. ) ;
#2401=DIRECTION ( 'NONE',  ( 0.000000000000000000, 0.000000000000000000, 1.000000000000000000 ) ) ;
#2404=AXIS2_PLACEMENT_3D ( 'NONE', #10878, #9882, #1753 ) ;
#2415=EDGE_CURVE ( 'NONE', #9966, #3848, #8124, .T. ) ;
#2418=FACE_OUTER_BOUND ( 'NONE', #3802, .T. ) ;
#2420=CARTESIAN_POINT ( 'NONE',  ( -240.6986105847286694, 4.249529545457076729, 10.95469206492581371 ) ) ;
#2424=VECTOR ( 'NONE', #209, 1000.000000000000114 ) ;
#2425=VERTEX_POINT ( 'NONE', #7452 ) ;
#2427=VERTEX_POINT ( 'NONE', #6588 ) ;
#2429=CIRCLE ( 'NONE', #2002, 249.7999999999999829 ) ;
#2430=DIRECTION ( 'NONE',  ( 0.000000000000000000, 0.000000000000000000, 1.000000000000000000 ) ) ;
#2432=DIRECTION ( 'NONE',  ( 0.000000000000000000, 1.000000000000000000, 0.000000000000000000 ) ) ;
#2434=CARTESIAN_POINT ( 'NONE',  ( -238.7984600057413616, 0.6745672505613249381, -11.73164896005920710 ) ) ;
#2439=CARTESIAN_POINT ( 'NONE',  ( 197.8197553893920144, 30.00000000000000000, 64.27553482998850143 ) ) ;
#2441=CARTESIAN_POINT ( 'NONE',  ( -244.0876578025649621, 8.170278137860064405, -8.444514117778142648 ) ) ;
#2442=CARTESIAN_POINT ( 'NONE',  ( 71.82423009839129691, 18.00000000000000000, 190.8354503650405150 ) ) ;
#2443=ADVANCED_FACE ( 'NONE', ( #11591 ), #5, .F. ) ;
#2445=CARTESIAN_POINT ( 'NONE',  ( 0.000000000000000000, 0.000000000000000000, 0.000000000000000000 ) ) ;
#2448=CARTESIAN_POINT ( 'NONE',  ( -240.8352866738073601, -4.521734056337656682, -10.84609021955956898 ) ) ;
#2450=CARTESIAN_POINT ( 'NONE',  ( 197.8197553893920144, 18.00000000000000000, 57.77553482998850853 ) ) ;
#2461=FACE_OUTER_BOUND ( 'NONE', #4092, .T. ) ;
#2476=CARTESIAN_POINT ( 'NONE',  ( 197.8197553893915028, 19.00000000000000000, -64.27553482998990830 ) ) ;
#2479=EDGE_CURVE ( 'NONE', #11054, #11150, #8522, .T. ) ;
#2480=CARTESIAN_POINT ( 'NONE',  ( 0.000000000000000000, 0.000000000000000000, 0.000000000000000000 ) ) ;
#2491=ORIENTED_EDGE ( 'NONE', *, *, #3333, .T. ) ;
#2492=VERTEX_POINT ( 'NONE', #6844 ) ;
#2496=CARTESIAN_POINT ( 'NONE',  ( 239.4667603743168058, 1.483520951545550526, -3.170043417372648165 ) ) ;
#2497=FACE_OUTER_BOUND ( 'NONE', #1014, .T. ) ;
#2500=CARTESIAN_POINT ( 'NONE',  ( -238.8666832504503930, -0.8657828299950671713, 11.71814331008092402 ) ) ;
#2502=ORIENTED_EDGE ( 'NONE', *, *, #12791, .F. ) ;
#2504=CARTESIAN_POINT ( 'NONE',  ( -240.1208361041844910, 2.772967769358964940, -11.41810622433052025 ) ) ;
#2505=CARTESIAN_POINT ( 'NONE',  ( -122.2593324768359935, 18.00000000000000000, -161.7755348299880040 ) ) ;
#2506=CARTESIAN_POINT ( 'NONE',  ( 0.000000000000000000, 0.000000000000000000, -250.0000000000000000 ) ) ;
#2507=DIRECTION ( 'NONE',  ( 0.000000000000000000, 0.000000000000000000, 1.000000000000000000 ) ) ;
#2509=CARTESIAN_POINT ( 'NONE',  ( -229.8692747951969579, 8.832110811273086171, 7.759242523040085437 ) ) ;
#2512=EDGE_CURVE ( 'NONE', #4880, #1904, #11920, .T. ) ;
#2518=CIRCLE ( 'NONE', #1455, 6.500000000000005329 ) ;
#2523=ORIENTED_EDGE ( 'NONE', *, *, #5493, .T. ) ;
#2527=CARTESIAN_POINT ( 'NONE',  ( 0.000000000000000000, 30.00000000000000000, 0.000000000000000000 ) ) ;
#2528=FACE_OUTER_BOUND ( 'NONE', #3079, .T. ) ;
#2529=EDGE_CURVE ( 'NONE', #4415, #6490, #465, .T. ) ;
#2532=CYLINDRICAL_SURFACE ( 'NONE', #6653, 245.7999999999999829 ) ;
#2534=CARTESIAN_POINT ( 'NONE',  ( 229.9832014715669004, 2.135344109160686177, -2.782701128735099338 ) ) ;
#2535=VECTOR ( 'NONE', #12221, 1000.000000000000000 ) ;
#2537=DIRECTION ( 'NONE',  ( 0.000000000000000000, 0.000000000000000000, 1.000000000000000000 ) ) ;
#2538=EDGE_LOOP ( 'NONE', ( #5365, #3282, #8439, #7987 ) ) ;
#2540=EDGE_CURVE ( 'NONE', #5028, #9692, #5348, .T. ) ;
#2545=DIRECTION ( 'NONE',  ( 0.000000000000000000, 0.000000000000000000, -1.000000000000000000 ) ) ;
#2547=CARTESIAN_POINT ( 'NONE',  ( -240.9194688703003067, 4.677296208860544979, 10.77948277563700330 ) ) ;
#2548=DIRECTION ( 'NONE',  ( 0.000000000000000000, 0.000000000000000000, -1.000000000000000000 ) ) ;
#2550=ORIENTED_EDGE ( 'NONE', *, *, #956, .F. ) ;
#2551=ORIENTED_EDGE ( 'NONE', *, *, #554, .F. ) ;
#2555=EDGE_CURVE ( 'NONE', #1760, #9966, #4072, .T. ) ;
#2563=CARTESIAN_POINT ( 'NONE',  ( 122.2593324768334071, 19.00000000000000000, -173.7755348299895104 ) ) ;
#2564=EDGE_LOOP ( 'NONE', ( #2822, #4515, #8322, #1744 ) ) ;
#2566=ORIENTED_EDGE ( 'NONE', *, *, #1850, .F. ) ;
#2567=CARTESIAN_POINT ( 'NONE',  ( -244.1927368939279859, 8.241533436879795005, -8.374943116871326865 ) ) ;
#2569=ORIENTED_EDGE ( 'NONE', *, *, #4322, .F. ) ;
#2575=CIRCLE ( 'NONE', #12592, 6.500000000000005329 ) ;
#2578=EDGE_CURVE ( 'NONE', #11921, #2857, #6982, .T. ) ;
#2580=CARTESIAN_POINT ( 'NONE',  ( -122.2593324768321992, 18.00000000000000000, 168.2755348299905052 ) ) ;
#2582=ORIENTED_EDGE ( 'NONE', *, *, #4322, .T. ) ;
#2586=DIRECTION ( 'NONE',  ( 0.000000000000000000, -1.000000000000000000, 0.000000000000000000 ) ) ;
#2588=CIRCLE ( 'NONE', #9201, 6.500000000000005329 ) ;
#2594=AXIS2_PLACEMENT_3D ( 'NONE', #7268, #5261, #10257 ) ;
#2598=TOROIDAL_SURFACE ( 'NONE', #5150, 238.4705882352940307, 2.000000000000000000 ) ;
#2599=EDGE_LOOP ( 'NONE', ( #11147, #11321, #6390, #12753, #2243, #12299 ) ) ;
#2603=DIRECTION ( 'NONE',  ( 0.000000000000000000, 0.7071067811865480168, 0.7071067811865470176 ) ) ;
#2604=DIRECTION ( 'NONE',  ( 8.659560562354572940E-17, -0.7071067811865771047, 0.7071067811865180408 ) ) ;
#2608=CIRCLE ( 'NONE', #3036, 2.000000000000001776 ) ;
#2611=ORIENTED_EDGE ( 'NONE', *, *, #6441, .T. ) ;
#2612=FACE_OUTER_BOUND ( 'NONE', #4380, .T. ) ;
#2616=CONICAL_SURFACE ( 'NONE', #7732, 6.500000000000005329, 0.7853981633974476129 ) ;
#2620=CARTESIAN_POINT ( 'NONE',  ( -240.0943994960963721, 2.684989249075541817, -11.43947242957938037 ) ) ;
#2625=TOROIDAL_SURFACE ( 'NONE', #513, 247.7999999999999829, 2.000000000000000000 ) ;
#2626=EDGE_CURVE ( 'NONE', #8550, #11184, #2575, .T. ) ;
#2631=CARTESIAN_POINT ( 'NONE',  ( -242.6830939082452403, 7.008887184829689865, -9.430537149009394327 ) ) ;
#2639=DIRECTION ( 'NONE',  ( 0.000000000000000000, 0.000000000000000000, 1.000000000000000000 ) ) ;
#2641=DIRECTION ( 'NONE',  ( 0.000000000000000000, 0.000000000000000000, 1.000000000000000000 ) ) ;
#2642=AXIS2_PLACEMENT_3D ( 'NONE', #10598, #9474, #10475 ) ;
#2644=ADVANCED_FACE ( 'NONE', ( #5849 ), #9397, .F. ) ;
#2645=ORIENTED_EDGE ( 'NONE', *, *, #8234, .T. ) ;
#2646=CARTESIAN_POINT ( 'NONE',  ( 3.010181832304193602E-14, 25.00000000000000000, 245.7999999999999829 ) ) ;
#2647=ORIENTED_EDGE ( 'NONE', *, *, #9123, .F. ) ;
#2654=DIRECTION ( 'NONE',  ( -1.000000000000000000, 0.000000000000000000, 0.000000000000000000 ) ) ;
#2656=CARTESIAN_POINT ( 'NONE',  ( 229.9760364581192960, 1.127696253648076574, -3.321182350956919827 ) ) ;
#2657=CARTESIAN_POINT ( 'NONE',  ( -249.6793054725033585, 11.18791971373266669, -3.590677820213459714 ) ) ;
#2662=EDGE_LOOP ( 'NONE', ( #2824, #6264, #2674, #3519 ) ) ;
#2665=CARTESIAN_POINT ( 'NONE',  ( 3.059167704270088292E-14, 29.00000000000000000, 249.7999999999999829 ) ) ;
#2667=CARTESIAN_POINT ( 'NONE',  ( -197.8197553893924976, 30.00000000000000000, -64.27553482998719403 ) ) ;
#2670=DIRECTION ( 'NONE',  ( 0.000000000000000000, -1.000000000000000000, 0.000000000000000000 ) ) ;
#2672=VERTEX_POINT ( 'NONE', #1036 ) ;
#2674=ORIENTED_EDGE ( 'NONE', *, *, #2074, .T. ) ;
#2677=ORIENTED_EDGE ( 'NONE', *, *, #12177, .F. ) ;
#2679=CARTESIAN_POINT ( 'NONE',  ( 0.000000000000000000, 0.000000000000000000, 0.000000000000000000 ) ) ;
#2685=ORIENTED_EDGE ( 'NONE', *, *, #1829, .T. ) ;
#2686=CARTESIAN_POINT ( 'NONE',  ( -238.7109915768028827, -0.1647346007394138723, 11.75000001785272907 ) ) ;
#2687=ORIENTED_EDGE ( 'NONE', *, *, #9342, .T. ) ;
#2689=CARTESIAN_POINT ( 'NONE',  ( -241.2291919109576668, 5.202024195572752419, -10.53597307948211537 ) ) ;
#2692=DIRECTION ( 'NONE',  ( 0.000000000000000000, 1.000000000000000000, 0.000000000000000000 ) ) ;
#2693=CARTESIAN_POINT ( 'NONE',  ( 0.000000000000000000, 25.00000000000000000, 249.2999999999999829 ) ) ;
#2703=CARTESIAN_POINT ( 'NONE',  ( -248.8121438751099959, -10.11580272835092842, -5.977715408740924552 ) ) ;
#2704=ORIENTED_EDGE ( 'NONE', *, *, #3333, .F. ) ;
#2709=DIRECTION ( 'NONE',  ( 0.000000000000000000, -1.000000000000000000, 0.000000000000000000 ) ) ;
#2715=CARTESIAN_POINT ( 'NONE',  ( 229.9948767726982908, 3.146592572275391131, 1.549747132302859320 ) ) ;
#2716=AXIS2_PLACEMENT_3D ( 'NONE', #10132, #9589, #1069 ) ;
#2718=CARTESIAN_POINT ( 'NONE',  ( -249.7718704160319589, 11.53079703974196946, 2.260598010248053402 ) ) ;
#2721=ORIENTED_EDGE ( 'NONE', *, *, #1750, .F. ) ;
#2722=ORIENTED_EDGE ( 'NONE', *, *, #10125, .F. ) ;
#2723=CARTESIAN_POINT ( 'NONE',  ( 197.8197553893920144, 19.00000000000000000, 64.27553482998850143 ) ) ;
#2725=DIRECTION ( 'NONE',  ( 0.000000000000000000, 1.000000000000000000, 0.000000000000000000 ) ) ;
#2728=CONICAL_SURFACE ( 'NONE', #1682, 249.2999999999999829, 0.7853981633974207455 ) ;
#2731=DIRECTION ( 'NONE',  ( 0.000000000000000000, 0.000000000000000000, 1.000000000000000000 ) ) ;
#2733=AXIS2_PLACEMENT_3D ( 'NONE', #11603, #1332, #6472 ) ;
#2734=ORIENTED_EDGE ( 'NONE', *, *, #10750, .T. ) ;
#2735=CIRCLE ( 'NONE', #4653, 249.7999999999999829 ) ;
#2737=ORIENTED_EDGE ( 'NONE', *, *, #6959, .T. ) ;
#2739=CARTESIAN_POINT ( 'NONE',  ( 71.82423009839129691, 30.00000000000000000, 197.3354503650404865 ) ) ;
#2740=EDGE_LOOP ( 'NONE', ( #1694, #5351, #12010, #499 ) ) ;
#2741=CARTESIAN_POINT ( 'NONE',  ( 0.000000000000000000, 29.00000000000000000, -208.0000000000000000 ) ) ;
#2744=LINE ( 'NONE', #6834, #6280 ) ;
#2745=DIRECTION ( 'NONE',  ( 0.000000000000000000, 1.000000000000000000, 0.000000000000000000 ) ) ;
#2746=AXIS2_PLACEMENT_3D ( 'NONE', #717, #6781, #5909 ) ;
#2747=ORIENTED_EDGE ( 'NONE', *, *, #624, .T. ) ;
#2749=ORIENTED_EDGE ( 'NONE', *, *, #9962, .T. ) ;
#2750=CARTESIAN_POINT ( 'NONE',  ( -239.1925639823984397, 1.468143814834786953, 11.65791906053731708 ) ) ;
#2757=CARTESIAN_POINT ( 'NONE',  ( 240.2635760546321819, 2.467011616145750708, 2.483268943481589996 ) ) ;
#2758=CARTESIAN_POINT ( 'NONE',  ( 0.000000000000000000, 19.00000000000000000, -208.0000000000000000 ) ) ;
#2759=CARTESIAN_POINT ( 'NONE',  ( -247.3797639061697851, 9.674571922615484709, 6.668012154210222420 ) ) ;
#2762=AXIS2_PLACEMENT_3D ( 'NONE', #9316, #186, #2379 ) ;
#2770=ORIENTED_EDGE ( 'NONE', *, *, #2059, .T. ) ;
#2772=CARTESIAN_POINT ( 'NONE',  ( -249.6681481789321708, -11.15796663577227932, -3.682817568939428909 ) ) ;
#2775=LINE ( 'NONE', #4785, #1261 ) ;
#2778=CIRCLE ( 'NONE', #1732, 5.099999999999993427 ) ;
#2783=EDGE_CURVE ( 'NONE', #10052, #7690, #6636, .T. ) ;
#2784=CARTESIAN_POINT ( 'NONE',  ( 229.9737082357617624, 0.4553564789625448861, -3.477861664728034263 ) ) ;
#2787=CARTESIAN_POINT ( 'NONE',  ( -249.6893775634945598, 11.21617121202809564, -3.501676137307497605 ) ) ;
#2791=ORIENTED_EDGE ( 'NONE', *, *, #7366, .F. ) ;
#2793=LINE ( 'NONE', #11137, #9264 ) ;
#2794=DIRECTION ( 'NONE',  ( 0.000000000000000000, 0.000000000000000000, 1.000000000000000000 ) ) ;
#2795=B_SPLINE_CURVE_WITH_KNOTS ( 'NONE', 3,
 ( #11105, #10232, #10041, #2894, #5031, #6976, #6178, #8247, #2963, #12305, #2170, #977, #3905, #12969, #9241, #116, #6639, #5162, #4170, #1038, #11231, #6247, #10299, #8043, #1178, #3968, #4102, #1976 ),
 .UNSPECIFIED., .F., .F.,
 ( 4, 2, 1, 2, 2, 2, 1, 1, 2, 2, 2, 1, 1, 1, 2, 2, 4 ),
 ( 0.5011901855632154845, 0.5635414123677892073, 0.5947170257700761242, 0.6103048324712180284, 0.6258926391723599325, 0.6882438659769362088, 0.7194194793792243470, 0.7350072860803684716, 0.7428011894309405339, 0.7505950927815124851, 0.8129463195861132974, 0.8441219329884137590, 0.8597097396895591048, 0.8675036430401318333, 0.8714005947154180864, 0.8752975463907042286, 1.000000000000000000 ),
 .UNSPECIFIED. ) ;
#2800=FACE_OUTER_BOUND ( 'NONE', #1117, .T. ) ;
#2802=CARTESIAN_POINT ( 'NONE',  ( 122.2593324768334071, 19.00000000000000000, -168.2755348299895104 ) ) ;
#2803=EDGE_CURVE ( 'NONE', #5993, #5992, #6177, .T. ) ;
#2806=DIRECTION ( 'NONE',  ( 0.000000000000000000, 0.000000000000000000, 1.000000000000000000 ) ) ;
#2811=ORIENTED_EDGE ( 'NONE', *, *, #12656, .F. ) ;
#2813=CARTESIAN_POINT ( 'NONE',  ( 197.8197553893920144, 30.00000000000000000, 64.27553482998850143 ) ) ;
#2814=FACE_OUTER_BOUND ( 'NONE', #288, .T. ) ;
#2818=VERTEX_POINT ( 'NONE', #11305 ) ;
#2819=CARTESIAN_POINT ( 'NONE',  ( -239.0854549270513871, -1.310333253960263455, 11.67674951774069392 ) ) ;
#2820=CONICAL_SURFACE ( 'NONE', #8377, 6.500000000000005329, 0.7853981633974476129 ) ;
#2822=ORIENTED_EDGE ( 'NONE', *, *, #10221, .F. ) ;
#2823=CARTESIAN_POINT ( 'NONE',  ( -245.3311829406554807, 8.905423747920915289, -7.665289359137143599 ) ) ;
#2824=ORIENTED_EDGE ( 'NONE', *, *, #9863, .F. ) ;
#2825=VECTOR ( 'NONE', #3740, 1000.000000000000000 ) ;
#2826=CARTESIAN_POINT ( 'NONE',  ( -197.8197553893909912, 18.00000000000000000, 64.27553482999130097 ) ) ;
#2827=CARTESIAN_POINT ( 'NONE',  ( 239.7985776503625175, 1.848645179571945185, 2.971954070985139751 ) ) ;
#2829=CARTESIAN_POINT ( 'NONE',  ( 122.2593324768334071, 19.00000000000000000, -168.2755348299895104 ) ) ;
#2831=FACE_BOUND ( 'NONE', #12509, .T. ) ;
#2835=VERTEX_POINT ( 'NONE', #4232 ) ;
#2836=CARTESIAN_POINT ( 'NONE',  ( 122.2593324768346008, 19.00000000000000000, 168.2755348299889988 ) ) ;
#2840=ORIENTED_EDGE ( 'NONE', *, *, #7148, .T. ) ;
#2841=CARTESIAN_POINT ( 'NONE',  ( -249.7048772686739255, -11.25744417650646234, -3.375279419700558670 ) ) ;
#2847=B_SPLINE_CURVE_WITH_KNOTS ( 'NONE', 3,
 ( #9460, #3441, #3511, #11595, #6526, #8653, #6659, #10580, #1450, #9577, #7583, #457, #11656, #2509, #10647, #1587, #5648, #4384, #259, #4317, #8398, #4906, #12044, #10842, #650, #10907, #10978, #11038, #9840, #3768, #3712, #8979, #1714, #6724, #721, #3638, #4771, #8847, #1912, #9975, #9700, #5780, #1784, #12908, #847, #9909 ),
 .UNSPECIFIED., .F., .F.,
 ( 4, 2, 2, 1, 2, 2, 2, 2, 2, 2, 2, 2, 2, 2, 2, 2, 2, 2, 2, 2, 1, 2, 2, 4 ),
 ( 0.03674184081479667241, 0.03903768231472214134, 0.04018560306468487581, 0.04133352381464761027, 0.04248144456461034474, 0.04362936531457307920, 0.04592520681449854814, 0.04707312756446127566, 0.04822104831442401013, 0.05051688981434948600, 0.05166481056431222046, 0.05281273131427495493, 0.05510857281420043774, 0.05740441431412590667, 0.05855233506408864808, 0.05970025581405138948, 0.06199609731397685841, 0.06429193881390234122, 0.06658778031382781015, 0.06773570106379055156, 0.06888362181375329296, 0.07003154256371602049, 0.07117946331367874802, 0.07347530481360423082 ),
 .UNSPECIFIED. ) ;
#2849=CARTESIAN_POINT ( 'NONE',  ( -240.0622992133938851, -2.599441824298837300, 11.45917237866061456 ) ) ;
#2850=CONICAL_SURFACE ( 'NONE', #9211, 6.500000000000005329, 0.7853981633974518317 ) ;
#2857=VERTEX_POINT ( 'NONE', #9304 ) ;
#2860=CARTESIAN_POINT ( 'NONE',  ( 0.000000000000000000, 30.00000000000000000, 214.5000000000000000 ) ) ;
#2861=CARTESIAN_POINT ( 'NONE',  ( 197.8197553893920144, 30.00000000000000000, 64.27553482998850143 ) ) ;
#2862=ADVANCED_FACE ( 'NONE', ( #6312 ), #7487, .F. ) ;
#2867=CARTESIAN_POINT ( 'NONE',  ( -245.0626974418777309, -8.766422715046710223, 7.824416521862886498 ) ) ;
#2878=EDGE_CURVE ( 'NONE', #12286, #2427, #8571, .T. ) ;
#2887=DIRECTION ( 'NONE',  ( 0.000000000000000000, 0.000000000000000000, 1.000000000000000000 ) ) ;
#2889=CARTESIAN_POINT ( 'NONE',  ( -239.1331745411521013, 1.386667391244157832, 11.66814598104677181 ) ) ;
#2890=EDGE_LOOP ( 'NONE', ( #10477, #5720, #8784, #9481 ) ) ;
#2892=EDGE_CURVE ( 'NONE', #3737, #12029, #11579, .T. ) ;
#2893=CARTESIAN_POINT ( 'NONE',  ( 240.2344515802825242, 2.410164965994779696, 2.538069655595715624 ) ) ;
#2894=CARTESIAN_POINT ( 'NONE',  ( 238.9937144808838241, 0.3120165756308810878, 3.486321029130972082 ) ) ;
#2896=CYLINDRICAL_SURFACE ( 'NONE', #10301, 5.500000000000005329 ) ;
#2900=ORIENTED_EDGE ( 'NONE', *, *, #4675, .F. ) ;
#2904=CARTESIAN_POINT ( 'NONE',  ( -248.0831933713610056, -9.830508068705260172, -6.436117704883899115 ) ) ;
#2905=ORIENTED_EDGE ( 'NONE', *, *, #7767, .F. ) ;
#2909=DIRECTION ( 'NONE',  ( 0.000000000000000000, 1.000000000000000000, 0.000000000000000000 ) ) ;
#2910=AXIS2_PLACEMENT_3D ( 'NONE', #2316, #8465, #3373 ) ;
#2912=FACE_OUTER_BOUND ( 'NONE', #12450, .T. ) ;
#2914=CARTESIAN_POINT ( 'NONE',  ( -229.6996680450365318, -0.3834651091013355773, 11.74999999999999645 ) ) ;
#2921=DIRECTION ( 'NONE',  ( 0.000000000000000000, 0.7071067811865470176, 0.7071067811865480168 ) ) ;
#2922=DIRECTION ( 'NONE',  ( 0.000000000000000000, 0.000000000000000000, -1.000000000000000000 ) ) ;
#2933=ORIENTED_EDGE ( 'NONE', *, *, #8894, .T. ) ;
#2935=DIRECTION ( 'NONE',  ( 8.659560562354913137E-17, -0.7071067811865489050, 0.7071067811865460184 ) ) ;
#2946=CARTESIAN_POINT ( 'NONE',  ( -249.2136238158385027, 10.44210856395644882, 5.387711592781305292 ) ) ;
#2948=CONICAL_SURFACE ( 'NONE', #10409, 5.500000000000005329, 0.7853981633974461696 ) ;
#2951=CARTESIAN_POINT ( 'NONE',  ( -245.6111173893534385, 9.040876189779853078, 7.505250421144309847 ) ) ;
#2955=EDGE_CURVE ( 'NONE', #11853, #3329, #4119, .T. ) ;
#2957=EDGE_CURVE ( 'NONE', #3502, #8550, #7502, .T. ) ;
#2958=CARTESIAN_POINT ( 'NONE',  ( -239.3015192883510736, 1.606994359549798856, 11.63956803321399391 ) ) ;
#2959=ORIENTED_EDGE ( 'NONE', *, *, #9709, .T. ) ;
#2963=CARTESIAN_POINT ( 'NONE',  ( 239.0510843050448671, 0.6173067666911031814, 3.446156762514750671 ) ) ;
#2965=AXIS2_PLACEMENT_3D ( 'NONE', #5574, #9633, #9384 ) ;
#2970=CARTESIAN_POINT ( 'NONE',  ( -238.7110077732466777, -0.01032322003152743271, -11.74999631638433861 ) ) ;
#2971=AXIS2_PLACEMENT_3D ( 'NONE', #11469, #7659, #7536 ) ;
#2976=CARTESIAN_POINT ( 'NONE',  ( -249.5826926913502177, -10.95569487808942810, 4.257357224404557883 ) ) ;
#2977=ORIENTED_EDGE ( 'NONE', *, *, #4837, .T. ) ;
#2980=DIRECTION ( 'NONE',  ( 0.000000000000000000, 0.000000000000000000, 1.000000000000000000 ) ) ;
#2982=CARTESIAN_POINT ( 'NONE',  ( -244.3371393051882876, -8.336835367652042805, -8.280174501370149542 ) ) ;
#2986=DIRECTION ( 'NONE',  ( 0.000000000000000000, 0.000000000000000000, -1.000000000000000000 ) ) ;
#2988=FACE_OUTER_BOUND ( 'NONE', #2564, .T. ) ;
#2989=ORIENTED_EDGE ( 'NONE', *, *, #8399, .T. ) ;
#2994=CARTESIAN_POINT ( 'NONE',  ( 238.9743710159888224, -9.335707311080796797E-14, -3.499999942258349428 ) ) ;
#2995=CARTESIAN_POINT ( 'NONE',  ( -239.5361044668159991, -1.848645179572815156, 11.60366368868215758 ) ) ;
#2996=AXIS2_PLACEMENT_3D ( 'NONE', #8904, #4902, #12905 ) ;
#2999=CARTESIAN_POINT ( 'NONE',  ( -244.2081860497233379, -8.251870589963452574, 8.364754208130431579 ) ) ;
#3002=APPLICATION_CONTEXT ( 'automotive_design' ) ;
#3004=EDGE_CURVE ( 'NONE', #1017, #12496, #4323, .T. ) ;
#3007=ORIENTED_EDGE ( 'NONE', *, *, #11779, .T. ) ;
#3008=ORIENTED_EDGE ( 'NONE', *, *, #371, .T. ) ;
#3011=CARTESIAN_POINT ( 'NONE',  ( -248.0831933713610056, 9.830508068705238856, 6.436117704883899115 ) ) ;
#3015=CARTESIAN_POINT ( 'NONE',  ( -245.4623802678685820, 8.970018888584359473, 7.589566415410549993 ) ) ;
#3017=LINE ( 'NONE', #5025, #10037 ) ;
#3019=EDGE_CURVE ( 'NONE', #889, #4307, #84, .T. ) ;
#3020=VERTEX_POINT ( 'NONE', #6510 ) ;
#3021=CARTESIAN_POINT ( 'NONE',  ( -245.0626974371188567, 8.766422712495943514, -7.824416524692094477 ) ) ;
#3022=ORIENTED_EDGE ( 'NONE', *, *, #1006, .F. ) ;
#3024=AXIS2_PLACEMENT_3D ( 'NONE', #10367, #4173, #2102 ) ;
#3026=CARTESIAN_POINT ( 'NONE',  ( 240.2035656452411558, 2.353769564626267297, 2.590352657692704508 ) ) ;
#3027=CARTESIAN_POINT ( 'NONE',  ( 0.000000000000000000, 30.00000000000000000, -248.7999999999999829 ) ) ;
#3029=DIRECTION ( 'NONE',  ( 0.000000000000000000, 1.000000000000000000, 0.000000000000000000 ) ) ;
#3030=ADVANCED_FACE ( 'NONE', ( #312 ), #3043, .F. ) ;
#3033=CARTESIAN_POINT ( 'NONE',  ( 71.82423009839129691, 30.00000000000000000, 197.3354503650404865 ) ) ;
#3036=AXIS2_PLACEMENT_3D ( 'NONE', #10028, #4619, #10825 ) ;
#3037=CARTESIAN_POINT ( 'NONE',  ( -239.2405902162603581, -1.531671746713636484, -11.64972311028024876 ) ) ;
#3039=CARTESIAN_POINT ( 'NONE',  ( -249.4806725022636442, 10.78221059153409733, -4.672140297476751414 ) ) ;
#3040=DIRECTION ( 'NONE',  ( 0.000000000000000000, -1.000000000000000000, 0.000000000000000000 ) ) ;
#3043=CONICAL_SURFACE ( 'NONE', #4746, 6.499999999999999112, 0.7853981633974476129 ) ;
#3047=FACE_OUTER_BOUND ( 'NONE', #8727, .T. ) ;
#3048=CARTESIAN_POINT ( 'NONE',  ( -247.3964713744789208, -9.678883351081529085, -6.661754107319017848 ) ) ;
#3055=ADVANCED_FACE ( 'NONE', ( #4683 ), #1356, .F. ) ;
#3057=AXIS2_PLACEMENT_3D ( 'NONE', #8472, #9403, #2396 ) ;
#3059=ORIENTED_EDGE ( 'NONE', *, *, #7901, .F. ) ;
#3060=EDGE_LOOP ( 'NONE', ( #1479, #7378, #3521, #2162, #1084, #11086, #8086, #10345 ) ) ;
#3064=AXIS2_PLACEMENT_3D ( 'NONE', #4907, #849, #3908 ) ;
#3065=DIRECTION ( 'NONE',  ( 0.000000000000000000, 1.000000000000000000, 0.000000000000000000 ) ) ;
#3070=CARTESIAN_POINT ( 'NONE',  ( -243.5599937326495592, -7.782121668009089888, 8.802892756717024980 ) ) ;
#3073=CARTESIAN_POINT ( 'NONE',  ( 7.960204194457795477E-16, 30.00000000000000000, -214.5000000000000000 ) ) ;
#3077=EDGE_LOOP ( 'NONE', ( #11633, #12821 ) ) ;
#3079=EDGE_LOOP ( 'NONE', ( #5767, #532 ) ) ;
#3086=CARTESIAN_POINT ( 'NONE',  ( -242.2664987710823823, 6.571392928988297299, 9.740637196669826636 ) ) ;
#3095=DIRECTION ( 'NONE',  ( 0.000000000000000000, 0.000000000000000000, -1.000000000000000000 ) ) ;
#3098=CYLINDRICAL_SURFACE ( 'NONE', #12182, 5.099999999999993427 ) ;
#3102=ORIENTED_EDGE ( 'NONE', *, *, #4505, .T. ) ;
#3103=CARTESIAN_POINT ( 'NONE',  ( 0.000000000000000000, 18.00000000000000000, 0.000000000000000000 ) ) ;
#3105=DIRECTION ( 'NONE',  ( 0.000000000000000000, 1.000000000000000000, 0.000000000000000000 ) ) ;
#3107=EDGE_CURVE ( 'NONE', #9249, #10068, #12423, .T. ) ;
#3108=CARTESIAN_POINT ( 'NONE',  ( -249.2798997179352796, -10.51457946798325160, 5.244637040187173582 ) ) ;
#3113=CARTESIAN_POINT ( 'NONE',  ( -246.4924783784645399, -9.403937934938156218, -7.045599359059536937 ) ) ;
#3115=CARTESIAN_POINT ( 'NONE',  ( -229.7074030909443252, -1.922301621807196881, 11.59804378764300736 ) ) ;
#3118=EDGE_CURVE ( 'NONE', #2857, #10498, #6706, .T. ) ;
#3121=VERTEX_POINT ( 'NONE', #12957 ) ;
#3124=DIRECTION ( 'NONE',  ( 0.000000000000000000, 1.000000000000000000, 0.000000000000000000 ) ) ;
#3129=CARTESIAN_POINT ( 'NONE',  ( -242.2606306403273209, -6.568547302997950865, 9.743049588217003176 ) ) ;
#3131=CIRCLE ( 'NONE', #3984, 249.2999999999999829 ) ;
#3132=EDGE_LOOP ( 'NONE', ( #9283, #13005, #12904, #9099 ) ) ;
#3137=EDGE_LOOP ( 'NONE', ( #10622, #369, #3399, #4261 ) ) ;
#3140=DIRECTION ( 'NONE',  ( 0.000000000000000000, 0.000000000000000000, 1.000000000000000000 ) ) ;
#3146=CARTESIAN_POINT ( 'NONE',  ( -247.2571636853384405, 9.642662941262603482, 6.714255740641853265 ) ) ;
#3147=EDGE_LOOP ( 'NONE', ( #11267, #7302, #267, #2721 ) ) ;
#3148=VECTOR ( 'NONE', #9156, 1000.000000000000000 ) ;
#3150=DIRECTION ( 'NONE',  ( 0.000000000000000000, 0.000000000000000000, 1.000000000000000000 ) ) ;
#3151=CIRCLE ( 'NONE', #10610, 5.500000000000005329 ) ;
#3155=VERTEX_POINT ( 'NONE', #8828 ) ;
#3156=ORIENTED_EDGE ( 'NONE', *, *, #6606, .F. ) ;
#3158=DIRECTION ( 'NONE',  ( 0.000000000000000000, -1.000000000000000000, 0.000000000000000000 ) ) ;
#3163=DIRECTION ( 'NONE',  ( 0.000000000000000000, 1.000000000000000000, 0.000000000000000000 ) ) ;
#3167=DIRECTION ( 'NONE',  ( 0.000000000000000000, -0.7071067811865480168, -0.7071067811865470176 ) ) ;
#3168=ORIENTED_EDGE ( 'NONE', *, *, #2783, .T. ) ;
#3169=CARTESIAN_POINT ( 'NONE',  ( -239.5361044668155159, 1.848645179572584896, -11.60366368868220022 ) ) ;
#3171=EDGE_CURVE ( 'NONE', #1172, #4030, #7103, .T. ) ;
#3174=CARTESIAN_POINT ( 'NONE',  ( -248.9847817896189213, -10.23580904445972450, 5.770128483534315400 ) ) ;
#3179=CARTESIAN_POINT ( 'NONE',  ( -241.8928034536404255, -6.135811582726104163, -10.02290695296160017 ) ) ;
#3181=AXIS2_PLACEMENT_3D ( 'NONE', #4331, #7203, #6082 ) ;
#3182=CARTESIAN_POINT ( 'NONE',  ( 239.4975972757000591, -1.524294659598023793, 3.150668454000119745 ) ) ;
#3191=CARTESIAN_POINT ( 'NONE',  ( 239.7985776503645354, -1.848645179573700004, -2.971954070984049956 ) ) ;
#3193=CARTESIAN_POINT ( 'NONE',  ( -249.6387411364665923, 11.08439570754534387, 3.900217602256478067 ) ) ;
#3194=LINE ( 'NONE', #2207, #2424 ) ;
#3195=EDGE_CURVE ( 'NONE', #2427, #6421, #10073, .T. ) ;
#3200=AXIS2_PLACEMENT_3D ( 'NONE', #5739, #4593, #9870 ) ;
#3201=CARTESIAN_POINT ( 'NONE',  ( -210.0000000000000000, 30.00000000000000000, 0.000000000000000000 ) ) ;
#3205=CARTESIAN_POINT ( 'NONE',  ( 229.9733680233431130, 4.286263893147487610E-16, -3.499999999999964917 ) ) ;
#3206=ORIENTED_EDGE ( 'NONE', *, *, #7931, .T. ) ;
#3208=DIRECTION ( 'NONE',  ( 0.000000000000000000, -1.000000000000000000, 0.000000000000000000 ) ) ;
#3209=ORIENTED_EDGE ( 'NONE', *, *, #10916, .F. ) ;
#3214=CYLINDRICAL_SURFACE ( 'NONE', #4942, 249.7999999999999829 ) ;
#3216=CARTESIAN_POINT ( 'NONE',  ( -244.6792151888649016, 8.549823287007102479, 8.060814821815563747 ) ) ;
#3217=ORIENTED_EDGE ( 'NONE', *, *, #11291, .F. ) ;
#3218=CARTESIAN_POINT ( 'NONE',  ( 229.9733680233429993, 8.492964294626340574E-17, 3.499999999999964917 ) ) ;
#3219=ADVANCED_FACE ( 'NONE', ( #10693 ), #6998, .F. ) ;
#3220=ORIENTED_EDGE ( 'NONE', *, *, #12961, .F. ) ;
#3223=EDGE_LOOP ( 'NONE', ( #4759, #11420, #5962, #11334 ) ) ;
#3225=CARTESIAN_POINT ( 'NONE',  ( 0.000000000000000000, -19.00000000000000000, 0.000000000000000000 ) ) ;
#3228=DIRECTION ( 'NONE',  ( 0.000000000000000000, 0.000000000000000000, 1.000000000000000000 ) ) ;
#3229=CARTESIAN_POINT ( 'NONE',  ( -238.9324529062528484, 1.023324755385371265, -11.70535849071079859 ) ) ;
#3233=EDGE_LOOP ( 'NONE', ( #5443, #4225, #11604, #11504 ) ) ;
#3234=DIRECTION ( 'NONE',  ( 0.000000000000000000, 0.000000000000000000, 1.000000000000000000 ) ) ;
#3235=AXIS2_PLACEMENT_3D ( 'NONE', #4353, #3277, #7360 ) ;
#3238=CARTESIAN_POINT ( 'NONE',  ( 0.000000000000000000, 25.50000000000000000, 0.000000000000000000 ) ) ;
#3240=CARTESIAN_POINT ( 'NONE',  ( -249.7849245721288867, -11.61140107739196559, 1.799432318634510919 ) ) ;
#3246=CARTESIAN_POINT ( 'NONE',  ( -245.8608051775114234, -9.153297364587587026, -7.368056644624257245 ) ) ;
#3249=CARTESIAN_POINT ( 'NONE',  ( 239.5749691952057674, -1.619550703834554017, 3.102778355627506368 ) ) ;
#3251=CARTESIAN_POINT ( 'NONE',  ( 0.000000000000000000, -2.957522019940860139E-14, -241.5000000000000000 ) ) ;
#3252=CIRCLE ( 'NONE', #1357, 5.099999999999993427 ) ;
#3253=FACE_OUTER_BOUND ( 'NONE', #12448, .T. ) ;
#3257=CARTESIAN_POINT ( 'NONE',  ( 197.8197553893915028, 19.00000000000000000, -64.27553482998990830 ) ) ;
#3258=CARTESIAN_POINT ( 'NONE',  ( -249.2423535134873873, 10.47282816799440752, 5.327573254783502854 ) ) ;
#3261=CARTESIAN_POINT ( 'NONE',  ( -210.0000000000000000, 30.00000000000000000, 6.500000000000000000 ) ) ;
#3262=ADVANCED_FACE ( 'NONE', ( #13023 ), #2089, .T. ) ;
#3269=DIRECTION ( 'NONE',  ( 0.000000000000000000, 1.000000000000000000, 0.000000000000000000 ) ) ;
#3270=CARTESIAN_POINT ( 'NONE',  ( 229.9849516113886807, -2.313877045632423357, 2.635927966202019412 ) ) ;
#3271=ORIENTED_EDGE ( 'NONE', *, *, #12233, .T. ) ;
#3277=DIRECTION ( 'NONE',  ( 0.000000000000000000, 1.000000000000000000, 0.000000000000000000 ) ) ;
#3282=ORIENTED_EDGE ( 'NONE', *, *, #1270, .F. ) ;
#3285=EDGE_LOOP ( 'NONE', ( #3585, #7282, #7364, #8630 ) ) ;
#3289=DIRECTION ( 'NONE',  ( 0.000000000000000000, 1.000000000000000000, 0.000000000000000000 ) ) ;
#3290=FACE_BOUND ( 'NONE', #4731, .T. ) ;
#3294=ADVANCED_FACE ( 'NONE', ( #7093 ), #7423, .F. ) ;
#3295=DIRECTION ( 'NONE',  ( 0.000000000000000000, 0.000000000000000000, 1.000000000000000000 ) ) ;
#3299=DIRECTION ( 'NONE',  ( 0.000000000000000000, 1.000000000000000000, 0.000000000000000000 ) ) ;
#3302=TOROIDAL_SURFACE ( 'NONE', #3947, 241.5000000000000000, 2.500000000000000000 ) ;
#3303=CARTESIAN_POINT ( 'NONE',  ( 122.2593324768346008, 18.00000000000000000, 168.2755348299889988 ) ) ;
#3305=EDGE_CURVE ( 'NONE', #58, #11184, #6341, .T. ) ;
#3309=FACE_OUTER_BOUND ( 'NONE', #1497, .T. ) ;
#3313=PRESENTATION_STYLE_ASSIGNMENT (( #9461 ) ) ;
#3317=B_SPLINE_CURVE_WITH_KNOTS ( 'NONE', 3,
 ( #9284, #11283, #4208, #7220, #9531, #10408, #351, #6487, #3330, #5415, #1151, #155, #412, #4342, #1349, #11482, #2343, #8291 ),
 .UNSPECIFIED., .F., .F.,
 ( 4, 2, 2, 2, 2, 2, 2, 2, 4 ),
 ( 0.000000000000000000, 0.1249999999999946709, 0.1874999999999935607, 0.2499999999999924505, 0.4999999999999944489, 0.6249999999999954481, 0.6874999999999965583, 0.7499999999999976685, 1.000000000000000000 ),
 .UNSPECIFIED. ) ;
#3318=DIRECTION ( 'NONE',  ( 0.000000000000000000, 1.000000000000000000, 0.000000000000000000 ) ) ;
#3326=DIRECTION ( 'NONE',  ( 0.000000000000000000, 1.000000000000000000, 0.000000000000000000 ) ) ;
#3328=CARTESIAN_POINT ( 'NONE',  ( 2.816687638038912194E-14, 0.000000000000000000, 230.0000000000000000 ) ) ;
#3329=VERTEX_POINT ( 'NONE', #8345 ) ;
#3330=CARTESIAN_POINT ( 'NONE',  ( 240.6324715325870045, -3.499918297958790170, -0.3875926898298525658 ) ) ;
#3333=EDGE_CURVE ( 'NONE', #4800, #5845, #12200, .T. ) ;
#3335=EDGE_CURVE ( 'NONE', #3781, #11051, #11249, .T. ) ;
#3341=DIRECTION ( 'NONE',  ( 0.000000000000000000, -0.7071067811865489050, -0.7071067811865460184 ) ) ;
#3352=CARTESIAN_POINT ( 'NONE',  ( 239.5143764669230677, 1.545628038502534718, -3.140199926907355721 ) ) ;
#3355=DIRECTION ( 'NONE',  ( 0.000000000000000000, -1.000000000000000000, 0.000000000000000000 ) ) ;
#3356=EDGE_CURVE ( 'NONE', #368, #6293, #8518, .T. ) ;
#3361=CARTESIAN_POINT ( 'NONE',  ( 2.400307726328812375E-14, 30.00000000000000000, -196.0000000000000000 ) ) ;
#3367=B_SPLINE_CURVE_WITH_KNOTS ( 'NONE', 3,
 ( #7814, #1762, #11890, #10889, #12954, #3819, #7885, #10959, #1354, #8297, #1220, #9289, #10346 ),
 .UNSPECIFIED., .F., .F.,
 ( 4, 2, 2, 1, 2, 2, 4 ),
 ( 0.000000000000000000, 0.2500000000000313083, 0.3750000000000306422, 0.4375000000000306422, 0.4687500000000305866, 0.5000000000000305311, 1.000000000000000000 ),
 .UNSPECIFIED. ) ;
#3372=VECTOR ( 'NONE', #6154, 1000.000000000000000 ) ;
#3373=DIRECTION ( 'NONE',  ( 0.000000000000000000, 0.000000000000000000, 1.000000000000000000 ) ) ;
#3377=( NAMED_UNIT ( * ) SI_UNIT ( $, .STERADIAN. ) SOLID_ANGLE_UNIT ( ) );
#3379=CARTESIAN_POINT ( 'NONE',  ( 240.6325187087303163, 3.500040777394010760, -0.1929172346387737214 ) ) ;
#3381=VECTOR ( 'NONE', #5912, 1000.000000000000000 ) ;
#3382=EDGE_CURVE ( 'NONE', #1401, #1635, #6386, .T. ) ;
#3384=VERTEX_POINT ( 'NONE', #11520 ) ;
#3386=CARTESIAN_POINT ( 'NONE',  ( 0.000000000000000000, 0.000000000000000000, 0.000000000000000000 ) ) ;
#3394=CARTESIAN_POINT ( 'NONE',  ( -247.1684828225455135, -9.630976094945838284, 6.736800401210575551 ) ) ;
#3396=B_SPLINE_CURVE_WITH_KNOTS ( 'NONE', 3,
 ( #9593, #11866, #2784, #9719, #2656, #10735, #11812, #2534, #1607, #546, #4591, #3532, #478, #4792, #3597, #6612, #9867, #744, #6680, #11741, #5669, #2715, #7864, #8867, #4527, #6871, #11933, #6807, #12928, #5735, #1738, #8667 ),
 .UNSPECIFIED., .F., .F.,
 ( 4, 2, 2, 2, 2, 2, 2, 2, 2, 2, 2, 2, 2, 2, 2, 4 ),
 ( 0.01094275811428774454, 0.01162652601767144404, 0.01231029392105514354, 0.01299406182443884304, 0.01367782972782254428, 0.01436159763120624204, 0.01504536553458994327, 0.01572913343797364277, 0.01641290134135733880, 0.01709666924474104177, 0.01778043714812473780, 0.01846420505150844077, 0.01914797295489213680, 0.01983174085827583630, 0.02051550876165953580, 0.02188304456842693480 ),
 .UNSPECIFIED. ) ;
#3398=CARTESIAN_POINT ( 'NONE',  ( -197.8197553893909912, 30.00000000000000000, 57.77553482999130807 ) ) ;
#3399=ORIENTED_EDGE ( 'NONE', *, *, #5644, .T. ) ;
#3400=ORIENTED_EDGE ( 'NONE', *, *, #9220, .F. ) ;
#3402=DIRECTION ( 'NONE',  ( 0.000000000000000000, 1.000000000000000000, 0.000000000000000000 ) ) ;
#3406=DIRECTION ( 'NONE',  ( 0.000000000000000000, 1.000000000000000000, 0.000000000000000000 ) ) ;
#3408=CARTESIAN_POINT ( 'NONE',  ( 197.8197553893920144, 19.00000000000000000, 64.27553482998850143 ) ) ;
#3412=VERTEX_POINT ( 'NONE', #3169 ) ;
#3413=CYLINDRICAL_SURFACE ( 'NONE', #5614, 195.0000000000000000 ) ;
#3417=ORIENTED_EDGE ( 'NONE', *, *, #6841, .T. ) ;
#3420=DIRECTION ( 'NONE',  ( 0.000000000000000000, 0.000000000000000000, 1.000000000000000000 ) ) ;
#3423=CARTESIAN_POINT ( 'NONE',  ( 239.2930894857298370, 1.216635601427789704, -3.281912597133258114 ) ) ;
#3424=CARTESIAN_POINT ( 'NONE',  ( -239.1925857173410748, 1.468173494105658117, -11.65791534653013350 ) ) ;
#3426=EDGE_CURVE ( 'NONE', #982, #4563, #5289, .T. ) ;
#3429=DIRECTION ( 'NONE',  ( -1.000000000000000000, 0.000000000000000000, 0.000000000000000000 ) ) ;
#3436=EDGE_CURVE ( 'NONE', #12239, #7634, #8908, .T. ) ;
#3438=EDGE_CURVE ( 'NONE', #8275, #12029, #2181, .T. ) ;
#3441=CARTESIAN_POINT ( 'NONE',  ( -229.6996680450366455, 0.7667553648700247138, 11.75000000000000355 ) ) ;
#3445=VECTOR ( 'NONE', #7711, 1000.000000000000000 ) ;
#3454=EDGE_CURVE ( 'NONE', #5992, #9288, #4859, .T. ) ;
#3455=DIRECTION ( 'NONE',  ( 0.000000000000000000, 0.000000000000000000, 1.000000000000000000 ) ) ;
#3456=LINE ( 'NONE', #1336, #1787 ) ;
#3457=AXIS2_PLACEMENT_3D ( 'NONE', #7765, #2745, #11024 ) ;
#3458=FACE_OUTER_BOUND ( 'NONE', #3899, .T. ) ;
#3463=VECTOR ( 'NONE', #6018, 1000.000000000000000 ) ;
#3465=CIRCLE ( 'NONE', #10075, 5.099999999999993427 ) ;
#3467=CONICAL_SURFACE ( 'NONE', #6473, 6.499999999999999112, 0.7853981633974476129 ) ;
#3473=ORIENTED_EDGE ( 'NONE', *, *, #3454, .F. ) ;
#3474=DIRECTION ( 'NONE',  ( 0.000000000000000000, 0.000000000000000000, 1.000000000000000000 ) ) ;
#3479=CARTESIAN_POINT ( 'NONE',  ( 197.8197553893920144, 30.00000000000000000, 57.77553482998850143 ) ) ;
#3481=CARTESIAN_POINT ( 'NONE',  ( 2.828934106030385709E-14, -20.00000000000000000, 231.0000000000000000 ) ) ;
#3487=CARTESIAN_POINT ( 'NONE',  ( 3.059167704270088292E-14, 21.50000000000000000, 249.7999999999999829 ) ) ;
#3488=VERTEX_POINT ( 'NONE', #6323 ) ;
#3494=DIRECTION ( 'NONE',  ( 0.000000000000000000, 1.000000000000000000, 0.000000000000000000 ) ) ;
#3495=AXIS2_PLACEMENT_3D ( 'NONE', #8764, #7764, #3826 ) ;
#3497=CARTESIAN_POINT ( 'NONE',  ( -238.7452622531599502, 0.4192131502268354182, -11.74262611718073579 ) ) ;
#3500=VERTEX_POINT ( 'NONE', #12451 ) ;
#3501=CARTESIAN_POINT ( 'NONE',  ( -238.8442808645216076, -0.8022036787917719014, 11.72256788271878492 ) ) ;
#3502=VERTEX_POINT ( 'NONE', #4434 ) ;
#3503=DIRECTION ( 'NONE',  ( 0.000000000000000000, 0.000000000000000000, 1.000000000000000000 ) ) ;
#3506=EDGE_CURVE ( 'NONE', #11184, #8550, #822, .T. ) ;
#3511=CARTESIAN_POINT ( 'NONE',  ( -229.7035075530963582, 1.528882821208700893, 11.67566906642231395 ) ) ;
#3512=CONICAL_SURFACE ( 'NONE', #7574, 5.500000000000005329, 0.7853981633974461696 ) ;
#3519=ORIENTED_EDGE ( 'NONE', *, *, #3708, .F. ) ;
#3520=DIRECTION ( 'NONE',  ( 0.000000000000000000, -1.000000000000000000, 0.000000000000000000 ) ) ;
#3521=ORIENTED_EDGE ( 'NONE', *, *, #6457, .T. ) ;
#3522=AXIS2_PLACEMENT_3D ( 'NONE', #9517, #11794, #2639 ) ;
#3531=EDGE_CURVE ( 'NONE', #6775, #10688, #9315, .T. ) ;
#3532=CARTESIAN_POINT ( 'NONE',  ( 229.9933834991255139, 3.036879765700447820, -1.754926613119420331 ) ) ;
#3533=EDGE_CURVE ( 'NONE', #3502, #58, #8063, .T. ) ;
#3535=DIRECTION ( 'NONE',  ( 0.000000000000000000, 1.000000000000000000, 0.000000000000000000 ) ) ;
#3536=ORIENTED_EDGE ( 'NONE', *, *, #10139, .T. ) ;
#3542=CARTESIAN_POINT ( 'NONE',  ( 0.000000000000000000, 30.00000000000000000, 0.000000000000000000 ) ) ;
#3545=DIRECTION ( 'NONE',  ( 0.000000000000000000, 0.000000000000000000, 1.000000000000000000 ) ) ;
#3547=ORIENTED_EDGE ( 'NONE', *, *, #10231, .T. ) ;
#3556=CARTESIAN_POINT ( 'NONE',  ( 239.0232640335058250, -0.4900023589501671384, -3.465599286982509408 ) ) ;
#3563=LINE ( 'NONE', #5507, #1990 ) ;
#3568=DIRECTION ( 'NONE',  ( 0.000000000000000000, 0.000000000000000000, 1.000000000000000000 ) ) ;
#3571=DIRECTION ( 'NONE',  ( -1.000000000000000000, -0.000000000000000000, -0.000000000000000000 ) ) ;
#3585=ORIENTED_EDGE ( 'NONE', *, *, #12911, .F. ) ;
#3586=CIRCLE ( 'NONE', #5079, 6.500000000000005329 ) ;
#3588=CARTESIAN_POINT ( 'NONE',  ( -122.2593324768321992, 19.00000000000000000, 168.2755348299905052 ) ) ;
#3589=DIRECTION ( 'NONE',  ( 0.000000000000000000, -1.000000000000000000, 0.000000000000000000 ) ) ;
#3592=FACE_BOUND ( 'NONE', #9008, .T. ) ;
#3593=CARTESIAN_POINT ( 'NONE',  ( -239.9440496357932204, -2.353898415756147777, 11.51208791644677731 ) ) ;
#3597=CARTESIAN_POINT ( 'NONE',  ( 229.9983154552353142, 3.387787197656995097, -0.9082533462923773060 ) ) ;
#3599=CARTESIAN_POINT ( 'NONE',  ( 2.388061258337338860E-14, 19.00000000000000000, 195.0000000000000000 ) ) ;
#3600=LINE ( 'NONE', #12730, #902 ) ;
#3602=ORIENTED_EDGE ( 'NONE', *, *, #8838, .T. ) ;
#3606=EDGE_CURVE ( 'NONE', #1432, #8308, #5642, .T. ) ;
#3607=EDGE_CURVE ( 'NONE', #9651, #11942, #6513, .T. ) ;
#3611=FACE_OUTER_BOUND ( 'NONE', #3137, .T. ) ;
#3612=CARTESIAN_POINT ( 'NONE',  ( -122.2593324768321992, 30.00000000000000000, 168.2755348299905052 ) ) ;
#3614=ORIENTED_EDGE ( 'NONE', *, *, #11354, .T. ) ;
#3618=ORIENTED_EDGE ( 'NONE', *, *, #12187, .F. ) ;
#3621=EDGE_CURVE ( 'NONE', #9495, #5845, #3735, .T. ) ;
#3623=DIRECTION ( 'NONE',  ( 0.000000000000000000, 1.000000000000000000, 0.000000000000000000 ) ) ;
#3625=LINE ( 'NONE', #1631, #9255 ) ;
#3627=EDGE_CURVE ( 'NONE', #8308, #6775, #4575, .T. ) ;
#3629=ORIENTED_EDGE ( 'NONE', *, *, #10718, .F. ) ;
#3630=DIRECTION ( 'NONE',  ( 0.000000000000000000, 0.7071067811865480168, 0.7071067811865470176 ) ) ;
#3636=DIRECTION ( 'NONE',  ( 0.000000000000000000, 0.7071067811865670016, 0.7071067811865280328 ) ) ;
#3638=CARTESIAN_POINT ( 'NONE',  ( -229.8110182538512447, 7.181715867726937041, -9.331701923201524806 ) ) ;
#3640=CARTESIAN_POINT ( 'NONE',  ( 197.8197553893920144, 30.00000000000000000, 69.77553482998851564 ) ) ;
#3646=EDGE_LOOP ( 'NONE', ( #2034, #9667 ) ) ;
#3647=ORIENTED_EDGE ( 'NONE', *, *, #11244, .T. ) ;
#3648=CARTESIAN_POINT ( 'NONE',  ( -249.2423535136895794, -10.47282816813556394, -5.327573254505493239 ) ) ;
#3654=VECTOR ( 'NONE', #912, 1000.000000000000000 ) ;
#3655=EDGE_CURVE ( 'NONE', #8497, #6601, #8355, .T. ) ;
#3658=DIRECTION ( 'NONE',  ( 0.000000000000000000, 1.000000000000000000, 0.000000000000000000 ) ) ;
#3660=CARTESIAN_POINT ( 'NONE',  ( -229.7576761218622892, -5.211361453271662114, -10.55923603912193798 ) ) ;
#3661=CIRCLE ( 'NONE', #4649, 6.500000000000005329 ) ;
#3664=CARTESIAN_POINT ( 'NONE',  ( -248.8927262318754856, 10.16869272944746427, -5.887412069865806785 ) ) ;
#3665=LINE ( 'NONE', #3599, #12574 ) ;
#3672=ADVANCED_FACE ( 'NONE', ( #1906 ), #3302, .F. ) ;
#3675=DIRECTION ( 'NONE',  ( 0.000000000000000000, 0.000000000000000000, 1.000000000000000000 ) ) ;
#3679=CARTESIAN_POINT ( 'NONE',  ( -197.8197553893909912, 19.00000000000000000, 64.27553482999130097 ) ) ;
#3681=EDGE_CURVE ( 'NONE', #789, #12455, #11618, .T. ) ;
#3683=ORIENTED_EDGE ( 'NONE', *, *, #1492, .T. ) ;
#3684=ORIENTED_EDGE ( 'NONE', *, *, #6699, .F. ) ;
#3689=VECTOR ( 'NONE', #4475, 1000.000000000000114 ) ;
#3691=CARTESIAN_POINT ( 'NONE',  ( -240.0622992133934872, 2.599441824297004544, -11.45917237866102845 ) ) ;
#3693=DIRECTION ( 'NONE',  ( 0.000000000000000000, -0.7071067811865489050, -0.7071067811865460184 ) ) ;
#3696=CARTESIAN_POINT ( 'NONE',  ( 0.000000000000000000, -19.00000000000000000, 249.7999999999999545 ) ) ;
#3697=PRODUCT_DEFINITION_SHAPE ( 'NONE', 'NONE',  #7672 ) ;
#3699=ORIENTED_EDGE ( 'NONE', *, *, #9789, .T. ) ;
#3702=ADVANCED_FACE ( 'NONE', ( #4029 ), #8108, .T. ) ;
#3708=EDGE_CURVE ( 'NONE', #1614, #10046, #2163, .T. ) ;
#3712=CARTESIAN_POINT ( 'NONE',  ( -229.9422451730981436, 10.56339097491623491, -5.203035948314511216 ) ) ;
#3714=DIRECTION ( 'NONE',  ( 0.000000000000000000, 0.000000000000000000, -1.000000000000000000 ) ) ;
#3717=CIRCLE ( 'NONE', #10535, 2.500000000000002220 ) ;
#3718=ORIENTED_EDGE ( 'NONE', *, *, #11421, .F. ) ;
#3721=CARTESIAN_POINT ( 'NONE',  ( -248.7900388717992257, -10.10208648675346055, -6.000868149951671171 ) ) ;
#3722=ORIENTED_EDGE ( 'NONE', *, *, #9547, .F. ) ;
#3724=DIRECTION ( 'NONE',  ( 0.000000000000000000, 0.000000000000000000, 1.000000000000000000 ) ) ;
#3725=CARTESIAN_POINT ( 'NONE',  ( -247.7878302976576776, -9.772649828929147020, -6.523883475188711145 ) ) ;
#3728=FACE_OUTER_BOUND ( 'NONE', #12986, .T. ) ;
#3730=CARTESIAN_POINT ( 'NONE',  ( -229.9848033347263652, -11.44892737729956345, -2.670968136663461667 ) ) ;
#3732=CARTESIAN_POINT ( 'NONE',  ( -249.7885090783126429, 11.63841215214888791, -1.617571259253988369 ) ) ;
#3733=DIRECTION ( 'NONE',  ( 0.000000000000000000, 0.000000000000000000, 1.000000000000000000 ) ) ;
#3734=CIRCLE ( 'NONE', #12891, 5.500000000000005329 ) ;
#3735=B_SPLINE_CURVE_WITH_KNOTS ( 'NONE', 3,
 ( #2504, #7576, #7701, #10640, #12703, #8647, #11842, #2689, #5703, #11586, #5772, #1637, #4695, #9695, #10832, #1511, #9761, #2631, #7638, #6651, #643, #11649, #8772, #12836, #7771, #6779, #5573, #1706, #9832, #714, #517, #4763, #4566, #7515, #12578, #2441, #11716, #2567, #10708, #1580, #576, #4624, #8705, #7039, #3021, #6970, #3964, #2823, #1969, #1778, #1034, #7271, #9100, #904, #7972, #5975, #6912, #2033, #7829, #12903, #12099, #4899, #8036, #8971, #5906, #11903, #9901 ),
 .UNSPECIFIED., .F., .F.,
 ( 4, 2, 2, 1, 1, 1, 1, 2, 2, 2, 2, 2, 1, 1, 1, 1, 1, 2, 2, 2, 2, 2, 1, 1, 1, 2, 2, 2, 2, 1, 1, 1, 1, 2, 2, 2, 2, 1, 1, 1, 2, 2, 4 ),
 ( 0.000000000000000000, 0.1250000000007419343, 0.1875000000011130541, 0.2187500000012986556, 0.2343750000013898882, 0.2421875000014337698, 0.2460937500014541701, 0.2480468750014659107, 0.2500000000014776513, 0.3750000000022004065, 0.4375000000025618396, 0.4687500000027445268, 0.4843750000028378966, 0.4921875000028826386, 0.4960937500029050651, 0.4980468750029143910, 0.4990234375029189429, 0.4995117187529211078, 0.5000000000029232172, 0.5625000000027089442, 0.5937500000026018077, 0.6093750000025481839, 0.6171875000025213165, 0.6210937500025078828, 0.6230468750024996671, 0.6240234375024956703, 0.6250000000024915625, 0.6875000000021134205, 0.7187500000019271251, 0.7343750000018338664, 0.7421875000017872370, 0.7460937500017674751, 0.7480468750017541524, 0.7490234375017439383, 0.7500000000017337243, 0.8125000000012649881, 0.8437500000010332846, 0.8593750000009204859, 0.8671875000008643086, 0.8710937500008359979, 0.8730468750008220091, 0.8750000000008079093, 1.000000000000000000 ),
 .UNSPECIFIED. ) ;
#3736=CARTESIAN_POINT ( 'NONE',  ( 0.000000000000000000, 30.00000000000000000, 208.0000000000000000 ) ) ;
#3737=VERTEX_POINT ( 'NONE', #10357 ) ;
#3740=DIRECTION ( 'NONE',  ( 0.000000000000000000, -1.000000000000000000, 0.000000000000000000 ) ) ;
#3742=DIRECTION ( 'NONE',  ( 0.000000000000000000, -0.7071067811865489050, -0.7071067811865460184 ) ) ;
#3744=CARTESIAN_POINT ( 'NONE',  ( -197.8197553893924976, 30.00000000000000000, -64.27553482998719403 ) ) ;
#3745=CARTESIAN_POINT ( 'NONE',  ( 197.8197553893915028, 30.00000000000000000, -70.77553482998990830 ) ) ;
#3746=ORIENTED_EDGE ( 'NONE', *, *, #5038, .F. ) ;
#3747=EDGE_CURVE ( 'NONE', #3753, #678, #1395, .T. ) ;
#3749=CARTESIAN_POINT ( 'NONE',  ( 0.000000000000000000, -2.772967769359314882, 240.3921568627447982 ) ) ;
#3751=ORIENTED_EDGE ( 'NONE', *, *, #7660, .T. ) ;
#3753=VERTEX_POINT ( 'NONE', #6173 ) ;
#3754=DIRECTION ( 'NONE',  ( 0.000000000000000000, 0.000000000000000000, 1.000000000000000000 ) ) ;
#3756=DIRECTION ( 'NONE',  ( 0.000000000000000000, 0.000000000000000000, -1.000000000000000000 ) ) ;
#3757=CARTESIAN_POINT ( 'NONE',  ( -247.7878302962004113, 9.772649828613312550, 6.523883475601624404 ) ) ;
#3761=EDGE_LOOP ( 'NONE', ( #10112, #3614, #10883, #8788 ) ) ;
#3762=CARTESIAN_POINT ( 'NONE',  ( -239.2239471044186416, 1.510219371731709170, 11.65254212361304198 ) ) ;
#3765=FACE_OUTER_BOUND ( 'NONE', #4962, .T. ) ;
#3767=EDGE_CURVE ( 'NONE', #10938, #2233, #127, .T. ) ;
#3768=CARTESIAN_POINT ( 'NONE',  ( -229.9631128808514973, 11.00533685364415248, -4.134445395687372127 ) ) ;
#3775=ORIENTED_EDGE ( 'NONE', *, *, #7056, .F. ) ;
#3778=ORIENTED_EDGE ( 'NONE', *, *, #1708, .T. ) ;
#3780=CARTESIAN_POINT ( 'NONE',  ( -249.6727234477500588, -11.17009475776062821, -3.645778574373556680 ) ) ;
#3781=VERTEX_POINT ( 'NONE', #4163 ) ;
#3785=DIRECTION ( 'NONE',  ( 0.000000000000000000, 0.000000000000000000, 1.000000000000000000 ) ) ;
#3797=AXIS2_PLACEMENT_3D ( 'NONE', #287, #5277, #8159 ) ;
#3798=CARTESIAN_POINT ( 'NONE',  ( -249.7845350863069029, 11.60862138571708968, -1.817256861374815458 ) ) ;
#3801=ORIENTED_EDGE ( 'NONE', *, *, #6936, .F. ) ;
#3802=EDGE_LOOP ( 'NONE', ( #3618, #8370, #5090, #5144, #5344, #6956 ) ) ;
#3803=DIRECTION ( 'NONE',  ( 0.000000000000000000, -1.000000000000000000, 0.000000000000000000 ) ) ;
#3804=DIRECTION ( 'NONE',  ( 0.000000000000000000, 1.000000000000000000, 0.000000000000000000 ) ) ;
#3806=VECTOR ( 'NONE', #6477, 1000.000000000000000 ) ;
#3811=DIRECTION ( 'NONE',  ( 0.000000000000000000, 0.000000000000000000, 1.000000000000000000 ) ) ;
#3812=DIRECTION ( 'NONE',  ( 0.000000000000000000, -1.000000000000000000, 0.000000000000000000 ) ) ;
#3813=AXIS2_PLACEMENT_3D ( 'NONE', #338, #400, #466 ) ;
#3818=ORIENTED_EDGE ( 'NONE', *, *, #8894, .F. ) ;
#3819=CARTESIAN_POINT ( 'NONE',  ( 240.1157413331997361, -2.212437690467188744, 2.712157915437692246 ) ) ;
#3821=DIRECTION ( 'NONE',  ( 0.000000000000000000, 0.000000000000000000, 1.000000000000000000 ) ) ;
#3826=DIRECTION ( 'NONE',  ( 0.000000000000000000, 0.000000000000000000, 1.000000000000000000 ) ) ;
#3831=CARTESIAN_POINT ( 'NONE',  ( 0.000000000000000000, -2.957522019940860139E-14, 0.000000000000000000 ) ) ;
#3833=CARTESIAN_POINT ( 'NONE',  ( 240.2193860685933942, -2.381856054525893551, -2.564741263598352639 ) ) ;
#3835=CARTESIAN_POINT ( 'NONE',  ( 197.8197553893915028, 18.00000000000000000, -57.77553482998991541 ) ) ;
#3838=LINE ( 'NONE', #8779, #5694 ) ;
#3843=ORIENTED_EDGE ( 'NONE', *, *, #5661, .T. ) ;
#3847=ADVANCED_FACE ( 'NONE', ( #10294 ), #10122, .T. ) ;
#3848=VERTEX_POINT ( 'NONE', #1232 ) ;
#3850=CARTESIAN_POINT ( 'NONE',  ( -249.7825649082131747, -11.59499477627102415, -1.902498381831638108 ) ) ;
#3851=VERTEX_POINT ( 'NONE', #7429 ) ;
#3856=AXIS2_PLACEMENT_3D ( 'NONE', #8112, #4034, #909 ) ;
#3857=ORIENTED_EDGE ( 'NONE', *, *, #4405, .T. ) ;
#3858=CARTESIAN_POINT ( 'NONE',  ( 0.000000000000000000, 9.830508068699479907, 0.000000000000000000 ) ) ;
#3863=EDGE_CURVE ( 'NONE', #1648, #4880, #5091, .T. ) ;
#3876=CIRCLE ( 'NONE', #9426, 248.1666666666679930 ) ;
#3877=CARTESIAN_POINT ( 'NONE',  ( -245.3834146150771574, -8.931379171322292976, 7.634986101120779800 ) ) ;
#3879=ORIENTED_EDGE ( 'NONE', *, *, #1750, .T. ) ;
#3880=CIRCLE ( 'NONE', #4512, 6.500000000000005329 ) ;
#3882=DIRECTION ( 'NONE',  ( 8.659560562354926695E-17, 0.7071067811865480168, -0.7071067811865470176 ) ) ;
#3884=ORIENTED_EDGE ( 'NONE', *, *, #8821, .T. ) ;
#3885=DIRECTION ( 'NONE',  ( 0.000000000000000000, 1.000000000000000000, 0.000000000000000000 ) ) ;
#3886=ORIENTED_EDGE ( 'NONE', *, *, #755, .F. ) ;
#3888=CONICAL_SURFACE ( 'NONE', #281, 6.500000000000005329, 0.7853981633974476129 ) ;
#3889=DIRECTION ( 'NONE',  ( 0.000000000000000000, 0.000000000000000000, 1.000000000000000000 ) ) ;
#3890=CONICAL_SURFACE ( 'NONE', #3457, 6.500000000000005329, 0.7853981633974476129 ) ;
#3894=ORIENTED_EDGE ( 'NONE', *, *, #3533, .F. ) ;
#3895=DIRECTION ( 'NONE',  ( 0.000000000000000000, 1.000000000000000000, 0.000000000000000000 ) ) ;
#3896=AXIS2_PLACEMENT_3D ( 'NONE', #5802, #11675, #6543 ) ;
#3898=AXIS2_PLACEMENT_3D ( 'NONE', #7379, #2177, #3234 ) ;
#3899=EDGE_LOOP ( 'NONE', ( #1066, #4148, #7825, #2905, #3775, #3602, #2502, #5828, #1215, #10412 ) ) ;
#3901=CARTESIAN_POINT ( 'NONE',  ( -239.3871160943602661, 1.704640309878053150, 11.62580261321480535 ) ) ;
#3902=EDGE_LOOP ( 'NONE', ( #10603, #5641, #12180, #12915 ) ) ;
#3904=DIRECTION ( 'NONE',  ( 0.000000000000000000, 0.000000000000000000, 1.000000000000000000 ) ) ;
#3905=CARTESIAN_POINT ( 'NONE',  ( 239.1683641398503255, 0.9613626713097240817, 3.365491595542490444 ) ) ;
#3906=CARTESIAN_POINT ( 'NONE',  ( 0.000000000000000000, -20.00000000000000000, 0.000000000000000000 ) ) ;
#3908=DIRECTION ( 'NONE',  ( 0.000000000000000000, 0.000000000000000000, -1.000000000000000000 ) ) ;
#3913=CARTESIAN_POINT ( 'NONE',  ( 197.8197553893920144, 19.00000000000000000, 58.77553482998850853 ) ) ;
#3919=CARTESIAN_POINT ( 'NONE',  ( -249.6587182942291179, -11.13358978280005118, -3.756204109176177752 ) ) ;
#3920=ORIENTED_EDGE ( 'NONE', *, *, #8649, .T. ) ;
#3924=DIRECTION ( 'NONE',  ( 0.000000000000000000, -1.000000000000000000, 0.000000000000000000 ) ) ;
#3927=AXIS2_PLACEMENT_3D ( 'NONE', #4398, #8289, #5412 ) ;
#3930=CARTESIAN_POINT ( 'NONE',  ( -229.9952077895577247, -11.65587983266546424, 1.533898002187394916 ) ) ;
#3934=AXIS2_PLACEMENT_3D ( 'NONE', #7862, #10182, #6130 ) ;
#3936=DIRECTION ( 'NONE',  ( 0.000000000000000000, 0.000000000000000000, -1.000000000000000000 ) ) ;
#3938=EDGE_CURVE ( 'NONE', #5812, #9614, #5869, .T. ) ;
#3941=FACE_OUTER_BOUND ( 'NONE', #9072, .T. ) ;
#3943=CARTESIAN_POINT ( 'NONE',  ( -242.7734209792739364, -7.097132674162740962, 9.364576600943349760 ) ) ;
#3946=ORIENTED_EDGE ( 'NONE', *, *, #846, .F. ) ;
#3947=AXIS2_PLACEMENT_3D ( 'NONE', #3831, #4964, #5027 ) ;
#3948=DIRECTION ( 'NONE',  ( 1.000000000000000000, 0.000000000000000000, 0.000000000000000000 ) ) ;
#3951=ORIENTED_EDGE ( 'NONE', *, *, #3767, .T. ) ;
#3957=EDGE_CURVE ( 'NONE', #468, #12455, #7562, .T. ) ;
#3959=CARTESIAN_POINT ( 'NONE',  ( -246.8900737811224815, 9.535158802951487544, 6.866190026894644305 ) ) ;
#3963=ORIENTED_EDGE ( 'NONE', *, *, #5644, .F. ) ;
#3964=CARTESIAN_POINT ( 'NONE',  ( -245.2595250062178707, 8.869312995476704486, -7.707186825661166196 ) ) ;
#3968=CARTESIAN_POINT ( 'NONE',  ( 239.5387464294004474, 1.581210111871798940, 3.124650851984021038 ) ) ;
#3969=DIRECTION ( 'NONE',  ( 0.000000000000000000, 0.000000000000000000, 1.000000000000000000 ) ) ;
#3970=LINE ( 'NONE', #9045, #4137 ) ;
#3977=ORIENTED_EDGE ( 'NONE', *, *, #8203, .T. ) ;
#3978=CARTESIAN_POINT ( 'NONE',  ( -249.2754563888361758, -10.50954084450015991, 5.254718384043918000 ) ) ;
#3979=ORIENTED_EDGE ( 'NONE', *, *, #7505, .T. ) ;
#3982=DIRECTION ( 'NONE',  ( 0.000000000000000000, -0.7071067811865489050, -0.7071067811865460184 ) ) ;
#3983=CARTESIAN_POINT ( 'NONE',  ( -246.7886136447417300, -9.502664450157794818, -6.911022174141807639 ) ) ;
#3984=AXIS2_PLACEMENT_3D ( 'NONE', #12800, #12775, #7837 ) ;
#3988=FACE_OUTER_BOUND ( 'NONE', #3761, .T. ) ;
#3992=DIRECTION ( 'NONE',  ( 0.000000000000000000, 0.000000000000000000, 1.000000000000000000 ) ) ;
#3993=ORIENTED_EDGE ( 'NONE', *, *, #3531, .T. ) ;
#3997=CYLINDRICAL_SURFACE ( 'NONE', #10007, 5.500000000000005329 ) ;
#3998=CIRCLE ( 'NONE', #5940, 6.499999999999999112 ) ;
#4003=CARTESIAN_POINT ( 'NONE',  ( -241.3417439075396373, -5.375691555202312344, 10.44818116087240512 ) ) ;
#4005=VERTEX_POINT ( 'NONE', #1368 ) ;
#4009=VECTOR ( 'NONE', #7382, 1000.000000000000000 ) ;
#4013=EDGE_CURVE ( 'NONE', #12433, #8176, #11476, .T. ) ;
#4014=CARTESIAN_POINT ( 'NONE',  ( 0.000000000000000000, 25.00000000000000000, 0.000000000000000000 ) ) ;
#4016=CIRCLE ( 'NONE', #8916, 5.500000000000005329 ) ;
#4023=CARTESIAN_POINT ( 'NONE',  ( -246.2885828769054228, 9.329251171726635761, 7.144935789750891608 ) ) ;
#4027=EDGE_LOOP ( 'NONE', ( #768, #1048 ) ) ;
#4029=FACE_OUTER_BOUND ( 'NONE', #1380, .T. ) ;
#4030=VERTEX_POINT ( 'NONE', #9681 ) ;
#4034=DIRECTION ( 'NONE',  ( 0.000000000000000000, 1.000000000000000000, 0.000000000000000000 ) ) ;
#4035=FACE_OUTER_BOUND ( 'NONE', #7495, .T. ) ;
#4040=CARTESIAN_POINT ( 'NONE',  ( 0.000000000000000000, 30.00000000000000000, 208.0000000000000000 ) ) ;
#4043=CARTESIAN_POINT ( 'NONE',  ( -238.9989076695733559, -1.159495732441587768, -11.69268798842454160 ) ) ;
#4044=AXIS2_PLACEMENT_3D ( 'NONE', #6478, #11673, #9715 ) ;
#4045=ORIENTED_EDGE ( 'NONE', *, *, #2051, .T. ) ;
#4046=CARTESIAN_POINT ( 'NONE',  ( -249.7994671776788209, 11.75014634418644377, -0.3782187742944450037 ) ) ;
#4047=CARTESIAN_POINT ( 'NONE',  ( 0.000000000000000000, 1.848645179567965036, 0.000000000000000000 ) ) ;
#4049=CARTESIAN_POINT ( 'NONE',  ( -249.7095932324938872, -11.27773618749138684, 3.298468584332664655 ) ) ;
#4050=ORIENTED_EDGE ( 'NONE', *, *, #1006, .T. ) ;
#4053=CARTESIAN_POINT ( 'NONE',  ( -239.8125244181988762, 2.098251439821959607, 11.56389750601951327 ) ) ;
#4054=CONICAL_SURFACE ( 'NONE', #8737, 249.7999999999999829, 0.7853981633974066456 ) ;
#4055=CARTESIAN_POINT ( 'NONE',  ( -247.1459274944737103, -9.611803614974679277, -6.758488902612981519 ) ) ;
#4057=CIRCLE ( 'NONE', #9521, 231.0000000000000000 ) ;
#4058=DIRECTION ( 'NONE',  ( 0.000000000000000000, 0.000000000000000000, -1.000000000000000000 ) ) ;
#4060=CARTESIAN_POINT ( 'NONE',  ( 0.000000000000000000, 19.00000000000000000, 0.000000000000000000 ) ) ;
#4061=CYLINDRICAL_SURFACE ( 'NONE', #265, 5.500000000000005329 ) ;
#4066=CARTESIAN_POINT ( 'NONE',  ( -241.2893272559581135, -5.295647553031770371, 10.48903809276563059 ) ) ;
#4069=VECTOR ( 'NONE', #5314, 1000.000000000000000 ) ;
#4070=CARTESIAN_POINT ( 'NONE',  ( 6.735557395310442023E-16, 30.00000000000000000, 202.4999999999999716 ) ) ;
#4072=CIRCLE ( 'NONE', #2996, 2.000000000000001776 ) ;
#4073=LINE ( 'NONE', #11075, #7721 ) ;
#4075=CARTESIAN_POINT ( 'NONE',  ( -241.8128863209092856, -6.047237972655528537, 10.08137159841291997 ) ) ;
#4078=FACE_BOUND ( 'NONE', #2342, .T. ) ;
#4079=CARTESIAN_POINT ( 'NONE',  ( 229.9933841504430063, -3.036907577538628278, -1.754770297504167464 ) ) ;
#4090=CARTESIAN_POINT ( 'NONE',  ( -242.8048495207236215, 7.129644030681907552, 9.341687345561288325 ) ) ;
#4092=EDGE_LOOP ( 'NONE', ( #5591, #9744, #1426, #11032 ) ) ;
#4094=CIRCLE ( 'NONE', #7291, 245.7999999999999829 ) ;
#4095=ORIENTED_EDGE ( 'NONE', *, *, #9465, .F. ) ;
#4097=ORIENTED_EDGE ( 'NONE', *, *, #846, .T. ) ;
#4100=DIRECTION ( 'NONE',  ( 0.000000000000000000, 1.000000000000000000, 0.000000000000000000 ) ) ;
#4101=CARTESIAN_POINT ( 'NONE',  ( 240.3826708216974737, 2.772967769358989809, 2.135567781667440102 ) ) ;
#4102=CARTESIAN_POINT ( 'NONE',  ( 239.6467530165474784, 1.711397835215433760, 3.057326063786706793 ) ) ;
#4103=CARTESIAN_POINT ( 'NONE',  ( 239.7985776503645354, -1.848645179573700004, -2.971954070984049956 ) ) ;
#4108=ADVANCED_FACE ( 'NONE', ( #2612 ), #5077, .F. ) ;
#4109=LINE ( 'NONE', #8190, #12039 ) ;
#4113=ORIENTED_EDGE ( 'NONE', *, *, #5991, .F. ) ;
#4114=CARTESIAN_POINT ( 'NONE',  ( -249.2798997179278615, 10.51457946798599608, -5.244637040181677534 ) ) ;
#4116=ADVANCED_FACE ( 'NONE', ( #1430 ), #7498, .F. ) ;
#4118=ORIENTED_EDGE ( 'NONE', *, *, #2230, .F. ) ;
#4119=CIRCLE ( 'NONE', #6040, 248.7999999999999829 ) ;
#4123=CARTESIAN_POINT ( 'NONE',  ( -244.5179878651543675, -8.451416882004156861, -8.163389688603578165 ) ) ;
#4125=EDGE_CURVE ( 'NONE', #7101, #12848, #2314, .T. ) ;
#4128=CARTESIAN_POINT ( 'NONE',  ( -229.7297352805116759, -3.784240722071517293, 11.15059988720178374 ) ) ;
#4129=AXIS2_PLACEMENT_3D ( 'NONE', #7365, #2090, #5224 ) ;
#4137=VECTOR ( 'NONE', #8045, 1000.000000000000114 ) ;
#4141=CARTESIAN_POINT ( 'NONE',  ( -210.0000000000000000, 28.60000000000000142, 0.000000000000000000 ) ) ;
#4143=CARTESIAN_POINT ( 'NONE',  ( -243.1580368189675028, -7.448595192430751410, 9.087405006325091961 ) ) ;
#4146=AXIS2_PLACEMENT_3D ( 'NONE', #11600, #6790, #1720 ) ;
#4148=ORIENTED_EDGE ( 'NONE', *, *, #4249, .T. ) ;
#4149=ORIENTED_EDGE ( 'NONE', *, *, #9689, .T. ) ;
#4157=CARTESIAN_POINT ( 'NONE',  ( -244.2871807289265575, 8.304201005827847482, 8.312831357947803923 ) ) ;
#4159=EDGE_CURVE ( 'NONE', #12455, #1965, #692, .T. ) ;
#4163=CARTESIAN_POINT ( 'NONE',  ( -197.8197553893924976, 18.00000000000000000, -57.77553482998720824 ) ) ;
#4170=CARTESIAN_POINT ( 'NONE',  ( 239.3359268382297387, 1.289900281958762385, 3.253812819694583691 ) ) ;
#4171=DIRECTION ( 'NONE',  ( 0.000000000000000000, 0.000000000000000000, 1.000000000000000000 ) ) ;
#4173=DIRECTION ( 'NONE',  ( 0.000000000000000000, 1.000000000000000000, 0.000000000000000000 ) ) ;
#4177=CARTESIAN_POINT ( 'NONE',  ( 0.000000000000000000, 18.00000000000000000, 0.000000000000000000 ) ) ;
#4183=EDGE_CURVE ( 'NONE', #167, #9614, #12947, .T. ) ;
#4185=CARTESIAN_POINT ( 'NONE',  ( -197.8197553893909912, 19.00000000000000000, 58.77553482999130807 ) ) ;
#4186=CARTESIAN_POINT ( 'NONE',  ( -242.3262939453856006, -6.637532586610901397, -9.695808798832128872 ) ) ;
#4187=CARTESIAN_POINT ( 'NONE',  ( 239.5143764665039043, -1.545628037973273861, 3.140199927189666340 ) ) ;
#4189=CARTESIAN_POINT ( 'NONE',  ( 240.5163796273739933, 3.187645493190168544, -1.494965077647770535 ) ) ;
#4191=AXIS2_PLACEMENT_3D ( 'NONE', #9357, #12483, #4537 ) ;
#4193=VERTEX_POINT ( 'NONE', #3749 ) ;
#4198=CARTESIAN_POINT ( 'NONE',  ( 239.3703217811417119, -1.345486616489417031, -3.231439195715531287 ) ) ;
#4199=FACE_OUTER_BOUND ( 'NONE', #6439, .T. ) ;
#4202=CARTESIAN_POINT ( 'NONE',  ( 0.000000000000000000, -2.926905849962176352E-14, 0.000000000000000000 ) ) ;
#4204=CYLINDRICAL_SURFACE ( 'NONE', #3927, 5.500000000000005329 ) ;
#4208=CARTESIAN_POINT ( 'NONE',  ( 240.4516407507180134, -2.994726891292637028, -1.822055168134961489 ) ) ;
#4209=CARTESIAN_POINT ( 'NONE',  ( 229.9831997411649525, -2.134968791774042529, -2.782786951242176787 ) ) ;
#4211=ORIENTED_EDGE ( 'NONE', *, *, #10605, .F. ) ;
#4213=CARTESIAN_POINT ( 'NONE',  ( -122.2593324768321992, 29.00000000000000000, 162.7755348299905052 ) ) ;
#4218=CARTESIAN_POINT ( 'NONE',  ( -243.4706526635933983, 7.711678326568429220, 8.866250685001064724 ) ) ;
#4220=AXIS2_PLACEMENT_3D ( 'NONE', #1088, #160, #7227 ) ;
#4221=AXIS2_PLACEMENT_3D ( 'NONE', #4177, #7182, #185 ) ;
#4223=CIRCLE ( 'NONE', #9974, 5.500000000000005329 ) ;
#4225=ORIENTED_EDGE ( 'NONE', *, *, #519, .F. ) ;
#4226=AXIS2_PLACEMENT_3D ( 'NONE', #25, #1082, #7156 ) ;
#4232=CARTESIAN_POINT ( 'NONE',  ( 240.3826708216974737, 2.772967769358989809, 2.135567781667440102 ) ) ;
#4233=DIRECTION ( 'NONE',  ( 0.000000000000000000, 0.000000000000000000, -1.000000000000000000 ) ) ;
#4235=CARTESIAN_POINT ( 'NONE',  ( -122.2593324768359935, 18.00000000000000000, -168.2755348299880040 ) ) ;
#4236=VECTOR ( 'NONE', #12584, 1000.000000000000114 ) ;
#4239=VECTOR ( 'NONE', #2019, 1000.000000000000000 ) ;
#4241=ORIENTED_EDGE ( 'NONE', *, *, #10221, .T. ) ;
#4242=DIRECTION ( 'NONE',  ( 0.000000000000000000, 1.000000000000000000, 0.000000000000000000 ) ) ;
#4244=CARTESIAN_POINT ( 'NONE',  ( 2.816687638038912194E-14, -19.00000000000000000, 230.0000000000000000 ) ) ;
#4246=CIRCLE ( 'NONE', #5087, 5.500000000000005329 ) ;
#4247=CARTESIAN_POINT ( 'NONE',  ( -249.7885090780623614, -11.63841214936962309, 1.617571278916385191 ) ) ;
#4248=EDGE_LOOP ( 'NONE', ( #787, #12563, #12783, #11818 ) ) ;
#4249=EDGE_CURVE ( 'NONE', #6601, #4565, #11285, .T. ) ;
#4253=CARTESIAN_POINT ( 'NONE',  ( -245.6948533279551157, -9.079155725198473803, -7.458842555897192028 ) ) ;
#4254=AXIS2_PLACEMENT_3D ( 'NONE', #11544, #540, #4394 ) ;
#4255=CARTESIAN_POINT ( 'NONE',  ( 239.7229759534581888, -1.780302303530038266, 3.014465403709621683 ) ) ;
#4257=EDGE_CURVE ( 'NONE', #7755, #158, #9943, .T. ) ;
#4259=EDGE_CURVE ( 'NONE', #1020, #4577, #4016, .T. ) ;
#4261=ORIENTED_EDGE ( 'NONE', *, *, #5542, .T. ) ;
#4263=CARTESIAN_POINT ( 'NONE',  ( 0.000000000000000000, -19.00000000000000000, 0.000000000000000000 ) ) ;
#4265=CARTESIAN_POINT ( 'NONE',  ( -122.2593324768359935, 18.00000000000000000, -168.2755348299880040 ) ) ;
#4267=DIRECTION ( 'NONE',  ( 0.000000000000000000, 1.000000000000000000, 0.000000000000000000 ) ) ;
#4269=CARTESIAN_POINT ( 'NONE',  ( 0.000000000000000000, -2.957522019940860139E-14, 0.000000000000000000 ) ) ;
#4271=EDGE_CURVE ( 'NONE', #12676, #468, #10829, .T. ) ;
#4272=CARTESIAN_POINT ( 'NONE',  ( -245.8522126016038101, -9.151584521558959295, 7.371153476891942447 ) ) ;
#4273=EDGE_CURVE ( 'NONE', #11841, #1954, #5292, .T. ) ;
#4275=DIRECTION ( 'NONE',  ( 0.000000000000000000, 1.000000000000000000, 0.000000000000000000 ) ) ;
#4279=EDGE_LOOP ( 'NONE', ( #6552, #3884, #4097, #5555 ) ) ;
#4281=DIRECTION ( 'NONE',  ( 0.000000000000000000, 1.000000000000000000, 0.000000000000000000 ) ) ;
#4284=AXIS2_PLACEMENT_3D ( 'NONE', #844, #6917, #1975 ) ;
#4287=CARTESIAN_POINT ( 'NONE',  ( -240.6618454235808997, 4.173161342497821558, 10.98396364135080461 ) ) ;
#4288=EDGE_CURVE ( 'NONE', #5643, #8360, #2078, .T. ) ;
#4290=DIRECTION ( 'NONE',  ( 0.000000000000000000, 0.000000000000000000, -1.000000000000000000 ) ) ;
#4291=ORIENTED_EDGE ( 'NONE', *, *, #5991, .T. ) ;
#4296=DIRECTION ( 'NONE',  ( 0.000000000000000000, 0.000000000000000000, 1.000000000000000000 ) ) ;
#4304=ORIENTED_EDGE ( 'NONE', *, *, #11690, .T. ) ;
#4307=VERTEX_POINT ( 'NONE', #2346 ) ;
#4308=AXIS2_PLACEMENT_3D ( 'NONE', #9013, #10074, #9140 ) ;
#4311=CARTESIAN_POINT ( 'NONE',  ( 197.8197553893915028, 29.00000000000000000, -64.27553482998990830 ) ) ;
#4312=EDGE_LOOP ( 'NONE', ( #6192, #2582, #13020, #5363 ) ) ;
#4313=DIRECTION ( 'NONE',  ( 0.000000000000000000, 0.000000000000000000, -1.000000000000000000 ) ) ;
#4314=DIRECTION ( 'NONE',  ( 0.000000000000000000, 0.000000000000000000, 1.000000000000000000 ) ) ;
#4317=CARTESIAN_POINT ( 'NONE',  ( -229.9691448513986529, 11.13025846491926885, 3.785357242864812122 ) ) ;
#4318=CARTESIAN_POINT ( 'NONE',  ( 239.0530249120693327, -0.6193663072279376181, 3.444815813525719861 ) ) ;
#4322=EDGE_CURVE ( 'NONE', #1020, #4307, #3600, .T. ) ;
#4323=CIRCLE ( 'NONE', #9639, 5.500000000000005329 ) ;
#4325=DIRECTION ( 'NONE',  ( 0.000000000000000000, 1.000000000000000000, 0.000000000000000000 ) ) ;
#4328=DIRECTION ( 'NONE',  ( 0.000000000000000000, 1.000000000000000000, 0.000000000000000000 ) ) ;
#4330=CARTESIAN_POINT ( 'NONE',  ( -249.2664547940201203, 10.49941023132624807, 5.274932156596537247 ) ) ;
#4331=CARTESIAN_POINT ( 'NONE',  ( 0.000000000000000000, 0.000000000000000000, 0.000000000000000000 ) ) ;
#4334=AXIS2_PLACEMENT_3D ( 'NONE', #1491, #10685, #9494 ) ;
#4335=CARTESIAN_POINT ( 'NONE',  ( 197.8197553893915028, 30.00000000000000000, -64.27553482998990830 ) ) ;
#4338=DIRECTION ( 'NONE',  ( 0.000000000000000000, 0.000000000000000000, 1.000000000000000000 ) ) ;
#4341=ORIENTED_EDGE ( 'NONE', *, *, #8399, .F. ) ;
#4342=CARTESIAN_POINT ( 'NONE',  ( 240.5832516929892222, -3.370511182595831379, 0.9484507947687070839 ) ) ;
#4347=DIRECTION ( 'NONE',  ( 0.000000000000000000, 0.000000000000000000, 1.000000000000000000 ) ) ;
#4349=EDGE_CURVE ( 'NONE', #3851, #4889, #479, .T. ) ;
#4350=B_SPLINE_CURVE_WITH_KNOTS ( 'NONE', 3,
 ( #11534, #139, #5326, #4386, #2193, #6272, #12523, #199, #11331, #3379, #10323, #7194, #1202, #5259, #336, #4189, #6334, #8467 ),
 .UNSPECIFIED., .F., .F.,
 ( 4, 2, 2, 2, 2, 2, 2, 2, 4 ),
 ( 0.000000000000000000, 0.1250000000000028588, 0.1875000000000042744, 0.2500000000000057176, 0.5000000000000069944, 0.6250000000000076605, 0.6875000000000074385, 0.7500000000000071054, 1.000000000000000000 ),
 .UNSPECIFIED. ) ;
#4353=CARTESIAN_POINT ( 'NONE',  ( 122.2593324768334071, 30.00000000000000000, -168.2755348299895104 ) ) ;
#4355=CARTESIAN_POINT ( 'NONE',  ( 71.82423009839129691, 19.40000000000000213, 192.2354503650404922 ) ) ;
#4358=ORIENTED_EDGE ( 'NONE', *, *, #6319, .T. ) ;
#4364=CARTESIAN_POINT ( 'NONE',  ( 197.8197553893915028, 30.00000000000000000, -64.27553482998990830 ) ) ;
#4365=EDGE_CURVE ( 'NONE', #8176, #6169, #11680, .T. ) ;
#4366=CARTESIAN_POINT ( 'NONE',  ( 0.000000000000000000, 19.00000000000000000, -208.0000000000000000 ) ) ;
#4368=CARTESIAN_POINT ( 'NONE',  ( 239.1625895582377552, 0.9513411440000743013, -3.369326940753043953 ) ) ;
#4369=DIRECTION ( 'NONE',  ( -1.000000000000000000, 0.000000000000000000, 0.000000000000000000 ) ) ;
#4371=EDGE_CURVE ( 'NONE', #6121, #1707, #6658, .T. ) ;
#4377=DIRECTION ( 'NONE',  ( 0.000000000000000000, -1.000000000000000000, 0.000000000000000000 ) ) ;
#4380=EDGE_LOOP ( 'NONE', ( #5976, #6224, #4981, #10289 ) ) ;
#4381=DIRECTION ( 'NONE',  ( 0.000000000000000000, 0.000000000000000000, -1.000000000000000000 ) ) ;
#4383=CARTESIAN_POINT ( 'NONE',  ( 238.9743710159888224, -9.335707311080796797E-14, -3.499999942258349428 ) ) ;
#4384=CARTESIAN_POINT ( 'NONE',  ( -229.9419135018622171, 10.55618113774804101, 5.217406956883983149 ) ) ;
#4386=CARTESIAN_POINT ( 'NONE',  ( 240.4969650423413725, 3.129188642588045077, 1.571450734147935790 ) ) ;
#4394=DIRECTION ( 'NONE',  ( 0.000000000000000000, 0.000000000000000000, -1.000000000000000000 ) ) ;
#4398=CARTESIAN_POINT ( 'NONE',  ( 197.8197553893920144, 30.00000000000000000, 64.27553482998850143 ) ) ;
#4405=EDGE_CURVE ( 'NONE', #6551, #2184, #11118, .T. ) ;
#4407=CIRCLE ( 'NONE', #381, 249.7999999999999829 ) ;
#4408=CARTESIAN_POINT ( 'NONE',  ( 122.2593324768346008, 30.00000000000000000, 168.2755348299889988 ) ) ;
#4410=DIRECTION ( 'NONE',  ( 0.000000000000000000, 1.000000000000000000, 0.000000000000000000 ) ) ;
#4415=VERTEX_POINT ( 'NONE', #10739 ) ;
#4421=DIRECTION ( 'NONE',  ( 0.000000000000000000, 0.000000000000000000, -1.000000000000000000 ) ) ;
#4423=CARTESIAN_POINT ( 'NONE',  ( 197.8197553893915028, 19.00000000000000000, -58.77553482998990830 ) ) ;
#4424=CARTESIAN_POINT ( 'NONE',  ( -239.5361044668155159, 1.848645179572584896, -11.60366368868220022 ) ) ;
#4428=AXIS2_PLACEMENT_3D ( 'NONE', #6278, #9469, #1335 ) ;
#4433=EDGE_CURVE ( 'NONE', #4958, #12890, #4094, .T. ) ;
#4434=CARTESIAN_POINT ( 'NONE',  ( 122.2593324768346008, 19.00000000000000000, 162.7755348299889988 ) ) ;
#4439=CARTESIAN_POINT ( 'NONE',  ( 0.000000000000000000, 2.772967769359004908, 0.000000000000000000 ) ) ;
#4450=CARTESIAN_POINT ( 'NONE',  ( 0.000000000000000000, 29.00000000000000000, -249.7999999999999829 ) ) ;
#4454=DIRECTION ( 'NONE',  ( 8.659560562354816994E-17, 0.7071067811865570096, -0.7071067811865380248 ) ) ;
#4455=DIRECTION ( 'NONE',  ( 0.000000000000000000, 0.000000000000000000, 1.000000000000000000 ) ) ;
#4459=DIRECTION ( 'NONE',  ( 0.000000000000000000, 0.000000000000000000, 1.000000000000000000 ) ) ;
#4461=CARTESIAN_POINT ( 'NONE',  ( 71.82423009839129691, 18.00000000000000000, 203.8354503650404581 ) ) ;
#4467=ORIENTED_EDGE ( 'NONE', *, *, #9054, .T. ) ;
#4475=DIRECTION ( 'NONE',  ( 0.000000000000000000, -0.7071067811865460184, -0.7071067811865489050 ) ) ;
#4477=DIRECTION ( 'NONE',  ( 1.000000000000000000, 0.000000000000000000, -1.224646799147353207E-16 ) ) ;
#4479=EDGE_CURVE ( 'NONE', #8155, #8360, #6016, .T. ) ;
#4490=CARTESIAN_POINT ( 'NONE',  ( 239.2050160255438414, 1.043887935153559487, -3.340720568028653137 ) ) ;
#4491=FACE_OUTER_BOUND ( 'NONE', #12271, .T. ) ;
#4495=ORIENTED_EDGE ( 'NONE', *, *, #7170, .F. ) ;
#4496=CARTESIAN_POINT ( 'NONE',  ( -238.7109915808064500, 2.244475480116206709E-14, 11.74999999995203126 ) ) ;
#4505=EDGE_CURVE ( 'NONE', #58, #4577, #6944, .T. ) ;
#4507=CARTESIAN_POINT ( 'NONE',  ( -241.0949697665562041, -4.988078590052489325, -10.64105268538957283 ) ) ;
#4510=FACE_OUTER_BOUND ( 'NONE', #1623, .T. ) ;
#4512=AXIS2_PLACEMENT_3D ( 'NONE', #4040, #1111, #9378 ) ;
#4514=CARTESIAN_POINT ( 'NONE',  ( -122.2593324768359935, 30.00000000000000000, -174.7755348299880040 ) ) ;
#4515=ORIENTED_EDGE ( 'NONE', *, *, #4918, .T. ) ;
#4520=DIRECTION ( 'NONE',  ( 0.000000000000000000, 1.000000000000000000, 0.000000000000000000 ) ) ;
#4521=ADVANCED_FACE ( 'NONE', ( #9871 ), #5375, .F. ) ;
#4523=CARTESIAN_POINT ( 'NONE',  ( 0.000000000000000000, -19.00000000000000000, 0.000000000000000000 ) ) ;
#4526=VECTOR ( 'NONE', #8635, 1000.000000000000114 ) ;
#4527=CARTESIAN_POINT ( 'NONE',  ( 229.9884417198156257, 2.638064155344324924, 2.311452626510129615 ) ) ;
#4528=CIRCLE ( 'NONE', #3898, 6.499999999999999112 ) ;
#4532=CONICAL_SURFACE ( 'NONE', #10668, 5.099999999999993427, 0.7853981633974461696 ) ;
#4535=EDGE_LOOP ( 'NONE', ( #7071, #1299 ) ) ;
#4537=DIRECTION ( 'NONE',  ( -1.224646799147349509E-16, 0.000000000000000000, -1.000000000000000000 ) ) ;
#4538=CONICAL_SURFACE ( 'NONE', #5407, 5.500000000000005329, 0.7853981633974461696 ) ;
#4543=CARTESIAN_POINT ( 'NONE',  ( 0.000000000000000000, 21.50000000000000000, -249.7999999999999829 ) ) ;
#4545=ORIENTED_EDGE ( 'NONE', *, *, #9622, .F. ) ;
#4547=AXIS2_PLACEMENT_3D ( 'NONE', #6412, #7401, #8280 ) ;
#4549=CARTESIAN_POINT ( 'NONE',  ( -197.8197553893909912, 29.00000000000000000, 64.27553482999130097 ) ) ;
#4553=CARTESIAN_POINT ( 'NONE',  ( 3.061616997868383121E-14, 0.000000000000000000, 250.0000000000000000 ) ) ;
#4556=CARTESIAN_POINT ( 'NONE',  ( 239.5494890110568065, 1.589230970485129735, -3.118420702611433892 ) ) ;
#4557=AXIS2_PLACEMENT_3D ( 'NONE', #9691, #1837, #8694 ) ;
#4561=DIRECTION ( 'NONE',  ( 0.000000000000000000, 0.000000000000000000, 1.000000000000000000 ) ) ;
#4563=VERTEX_POINT ( 'NONE', #8069 ) ;
#4565=VERTEX_POINT ( 'NONE', #12206 ) ;
#4566=CARTESIAN_POINT ( 'NONE',  ( -243.8540711624768846, 8.004651165874994589, -8.601279203521002614 ) ) ;
#4568=DIRECTION ( 'NONE',  ( 0.000000000000000000, 0.000000000000000000, -1.000000000000000000 ) ) ;
#4570=CYLINDRICAL_SURFACE ( 'NONE', #2910, 5.099999999999993427 ) ;
#4575=CIRCLE ( 'NONE', #6729, 230.0000000000000000 ) ;
#4577=VERTEX_POINT ( 'NONE', #10128 ) ;
#4579=ORIENTED_EDGE ( 'NONE', *, *, #9910, .F. ) ;
#4588=CARTESIAN_POINT ( 'NONE',  ( -240.0943994960961447, -2.684989249076883855, 11.43947242957905353 ) ) ;
#4589=LINE ( 'NONE', #9661, #9637 ) ;
#4591=CARTESIAN_POINT ( 'NONE',  ( 229.9901642561758592, 2.782416201478342455, -2.135548222472730462 ) ) ;
#4593=DIRECTION ( 'NONE',  ( 0.000000000000000000, 1.000000000000000000, 0.000000000000000000 ) ) ;
#4594=EDGE_CURVE ( 'NONE', #11853, #4811, #9198, .T. ) ;
#4595=DIRECTION ( 'NONE',  ( 0.000000000000000000, -1.000000000000000000, 0.000000000000000000 ) ) ;
#4598=CARTESIAN_POINT ( 'NONE',  ( 197.8197553893915028, 30.00000000000000000, -57.77553482998990830 ) ) ;
#4600=EDGE_CURVE ( 'NONE', #6169, #12610, #4938, .T. ) ;
#4605=DIRECTION ( 'NONE',  ( 0.000000000000000000, 1.000000000000000000, 0.000000000000000000 ) ) ;
#4606=FACE_OUTER_BOUND ( 'NONE', #11737, .T. ) ;
#4609=ORIENTED_EDGE ( 'NONE', *, *, #9485, .F. ) ;
#4611=ORIENTED_EDGE ( 'NONE', *, *, #3382, .F. ) ;
#4614=DIRECTION ( 'NONE',  ( 0.000000000000000000, 1.000000000000000000, 0.000000000000000000 ) ) ;
#4617=DIRECTION ( 'NONE',  ( 0.000000000000000000, -1.000000000000000000, 0.000000000000000000 ) ) ;
#4619=DIRECTION ( 'NONE',  ( -1.000000000000000000, 0.000000000000000000, 0.000000000000000000 ) ) ;
#4621=ORIENTED_EDGE ( 'NONE', *, *, #3533, .T. ) ;
#4624=CARTESIAN_POINT ( 'NONE',  ( -244.4597039919655117, 8.419215816066659031, -8.199143449616464352 ) ) ;
#4625=ORIENTED_EDGE ( 'NONE', *, *, #4600, .T. ) ;
#4628=CARTESIAN_POINT ( 'NONE',  ( 71.82423009839129691, 19.40000000000000213, 197.3354503650404865 ) ) ;
#4630=VECTOR ( 'NONE', #2603, 1000.000000000000000 ) ;
#4638=AXIS2_PLACEMENT_3D ( 'NONE', #2111, #7446, #10242 ) ;
#4639=ADVANCED_FACE ( 'NONE', ( #3253 ), #4061, .F. ) ;
#4641=CARTESIAN_POINT ( 'NONE',  ( -249.6767732310697454, -11.18100465982222502, -3.612153022818042736 ) ) ;
#4643=ORIENTED_EDGE ( 'NONE', *, *, #7170, .T. ) ;
#4644=CIRCLE ( 'NONE', #618, 5.499999999999998224 ) ;
#4649=AXIS2_PLACEMENT_3D ( 'NONE', #6203, #11266, #2129 ) ;
#4653=AXIS2_PLACEMENT_3D ( 'NONE', #456, #2313, #2255 ) ;
#4656=LINE ( 'NONE', #10863, #5859 ) ;
#4657=CONICAL_SURFACE ( 'NONE', #839, 5.500000000000005329, 0.7853981633974461696 ) ;
#4658=CARTESIAN_POINT ( 'NONE',  ( -249.7806011016498928, 11.58204051030000947, 1.980500725882820445 ) ) ;
#4665=CARTESIAN_POINT ( 'NONE',  ( 0.000000000000000000, -1.848645179579245124, 0.000000000000000000 ) ) ;
#4666=CIRCLE ( 'NONE', #5747, 240.3921568627449687 ) ;
#4670=DIRECTION ( 'NONE',  ( 0.000000000000000000, -1.000000000000000000, 0.000000000000000000 ) ) ;
#4675=EDGE_CURVE ( 'NONE', #7886, #534, #3661, .T. ) ;
#4677=DIRECTION ( 'NONE',  ( 0.000000000000000000, 0.000000000000000000, 1.000000000000000000 ) ) ;
#4682=AXIS2_PLACEMENT_3D ( 'NONE', #5473, #3269, #11552 ) ;
#4683=FACE_OUTER_BOUND ( 'NONE', #4885, .T. ) ;
#4684=CARTESIAN_POINT ( 'NONE',  ( -197.8197553893924976, 18.00000000000000000, -64.27553482998719403 ) ) ;
#4685=B_SPLINE_CURVE_WITH_KNOTS ( 'NONE', 3,
 ( #2994, #7076, #1697, #5765, #12694, #4753, #3556, #8829, #12893, #12072, #1942, #11273, #10332, #2135, #12275, #5062, #6210, #8346, #5336, #4198, #7275, #2206, #9407, #10266, #10198, #147, #6342, #3191 ),
 .UNSPECIFIED., .F., .F.,
 ( 4, 2, 1, 2, 2, 2, 1, 1, 2, 2, 2, 1, 1, 1, 2, 2, 4 ),
 ( 0.5011901855463575250, 0.5635414123530773089, 0.5947170257564382556, 0.6103048324581187289, 0.6258926391597992023, 0.6882438659665208736, 0.7194194793698815982, 0.7350072860715587408, 0.7428011894223938150, 0.7505950927732287781, 0.8129463195799428998, 0.8441219329832998497, 0.8597097396849784356, 0.8675036430358130657, 0.8714005947112304362, 0.8752975463866476957, 1.000000000000000000 ),
 .UNSPECIFIED. ) ;
#4686=CARTESIAN_POINT ( 'NONE',  ( 0.000000000000000000, 3.327561323230765034, 0.000000000000000000 ) ) ;
#4694=ORIENTED_EDGE ( 'NONE', *, *, #3356, .T. ) ;
#4695=CARTESIAN_POINT ( 'NONE',  ( -241.3472527820971152, 5.384021912553072831, -10.44389002222748886 ) ) ;
#4698=DIRECTION ( 'NONE',  ( 0.000000000000000000, 1.000000000000000000, 0.000000000000000000 ) ) ;
#4700=DIRECTION ( 'NONE',  ( 0.000000000000000000, 0.000000000000000000, 1.000000000000000000 ) ) ;
#4710=CARTESIAN_POINT ( 'NONE',  ( -249.2664547940505884, -10.49941023134739915, -5.274932156554418938 ) ) ;
#4711=EDGE_LOOP ( 'NONE', ( #6056, #793, #12913, #4781 ) ) ;
#4716=CARTESIAN_POINT ( 'NONE',  ( 0.000000000000000000, 22.00000000000000000, -249.2999999999999829 ) ) ;
#4718=ADVANCED_FACE ( 'NONE', ( #8274 ), #659, .F. ) ;
#4719=CARTESIAN_POINT ( 'NONE',  ( -239.7946578092521577, -2.116498006235906892, 11.55893420607609912 ) ) ;
#4720=ADVANCED_FACE ( 'NONE', ( #2988 ), #11483, .F. ) ;
#4723=CARTESIAN_POINT ( 'NONE',  ( -229.9691690360902498, -11.13075325490934020, -3.783731615047171370 ) ) ;
#4724=AXIS2_PLACEMENT_3D ( 'NONE', #13003, #872, #677 ) ;
#4727=CARTESIAN_POINT ( 'NONE',  ( -248.3532242375468684, 9.880481159981247430, -6.359788945912696612 ) ) ;
#4731=EDGE_LOOP ( 'NONE', ( #8673, #6174 ) ) ;
#4734=LINE ( 'NONE', #8810, #2825 ) ;
#4737=DIRECTION ( 'NONE',  ( 0.000000000000000000, 1.000000000000000000, 0.000000000000000000 ) ) ;
#4741=ORIENTED_EDGE ( 'NONE', *, *, #119, .F. ) ;
#4744=VERTEX_POINT ( 'NONE', #533 ) ;
#4745=ADVANCED_FACE ( 'NONE', ( #8468 ), #1687, .F. ) ;
#4746=AXIS2_PLACEMENT_3D ( 'NONE', #4364, #11506, #2235 ) ;
#4748=ADVANCED_FACE ( 'NONE', ( #7653 ), #7008, .F. ) ;
#4751=CONICAL_SURFACE ( 'NONE', #6042, 5.499999999999998224, 0.7853981633974461696 ) ;
#4753=CARTESIAN_POINT ( 'NONE',  ( 239.0147185140185115, -0.4456008732492039437, -3.471580854532841709 ) ) ;
#4759=ORIENTED_EDGE ( 'NONE', *, *, #7196, .F. ) ;
#4762=ORIENTED_EDGE ( 'NONE', *, *, #464, .F. ) ;
#4763=CARTESIAN_POINT ( 'NONE',  ( -243.6657758070387843, 7.864920305444456972, -8.729522397915381760 ) ) ;
#4767=DIRECTION ( 'NONE',  ( 0.000000000000000000, 1.000000000000000000, 0.000000000000000000 ) ) ;
#4771=CARTESIAN_POINT ( 'NONE',  ( -229.7836540530505829, 6.220351915703449919, -9.975897099602894613 ) ) ;
#4773=PLANE ( 'NONE',  #3064 ) ;
#4781=ORIENTED_EDGE ( 'NONE', *, *, #5385, .T. ) ;
#4782=CARTESIAN_POINT ( 'NONE',  ( -249.6197023358011222, -11.04161720068388952, -4.018949317641925312 ) ) ;
#4785=CARTESIAN_POINT ( 'NONE',  ( 197.8197553893915028, 30.00000000000000000, -58.77553482998990830 ) ) ;
#4789=VECTOR ( 'NONE', #6717, 1000.000000000000000 ) ;
#4792=CARTESIAN_POINT ( 'NONE',  ( 229.9973173948202430, 3.320200122780408325, -1.130823014037518170 ) ) ;
#4794=CARTESIAN_POINT ( 'NONE',  ( -249.7944461413453894, 11.69162236983806835, -1.179780665110756521 ) ) ;
#4796=AXIS2_PLACEMENT_3D ( 'NONE', #3679, #2670, #11951 ) ;
#4799=ORIENTED_EDGE ( 'NONE', *, *, #7048, .T. ) ;
#4800=VERTEX_POINT ( 'NONE', #10726 ) ;
#4801=EDGE_CURVE ( 'NONE', #167, #3488, #1475, .T. ) ;
#4808=CARTESIAN_POINT ( 'NONE',  ( 0.000000000000000000, 29.00000000000000000, -202.4999999999999716 ) ) ;
#4811=VERTEX_POINT ( 'NONE', #4450 ) ;
#4818=CARTESIAN_POINT ( 'NONE',  ( 7.960204194457795477E-16, 30.00000000000000000, 201.4999999999999716 ) ) ;
#4820=ADVANCED_FACE ( 'NONE', ( #12463 ), #5081, .F. ) ;
#4825=DIRECTION ( 'NONE',  ( 0.000000000000000000, 0.000000000000000000, -1.000000000000000000 ) ) ;
#4828=CARTESIAN_POINT ( 'NONE',  ( 240.1881190901118259, -2.326983775948836985, -2.614448608526312334 ) ) ;
#4830=DIRECTION ( 'NONE',  ( 0.000000000000000000, 0.000000000000000000, 1.000000000000000000 ) ) ;
#4837=EDGE_CURVE ( 'NONE', #12496, #1017, #7859, .T. ) ;
#4840=ORIENTED_EDGE ( 'NONE', *, *, #11342, .F. ) ;
#4841=CARTESIAN_POINT ( 'NONE',  ( -239.1938262371573103, -1.469859134671393397, -11.65770207259568281 ) ) ;
#4844=B_SPLINE_CURVE_WITH_KNOTS ( 'NONE', 3,
 ( #4101, #7978, #12042, #9907, #2757, #2893, #5096, #3026, #1910, #11169, #7904, #12103, #2827 ),
 .UNSPECIFIED., .F., .F.,
 ( 4, 2, 2, 1, 2, 2, 4 ),
 ( 0.000000000000000000, 0.2500000000000368594, 0.3750000000000559552, 0.4375000000000651701, 0.4687500000000694445, 0.5000000000000737188, 1.000000000000000000 ),
 .UNSPECIFIED. ) ;
#4847=CARTESIAN_POINT ( 'NONE',  ( -249.7718704162269319, -11.53079704007455142, -2.260598008543511561 ) ) ;
#4852=CARTESIAN_POINT ( 'NONE',  ( 197.8197553893920144, 30.00000000000000000, 58.77553482998850853 ) ) ;
#4854=B_SPLINE_CURVE_WITH_KNOTS ( 'NONE', 3,
 ( #5182, #4053, #10119, #10317 ),
 .UNSPECIFIED., .F., .F.,
 ( 4, 4 ),
 ( 0.000000000000000000, 1.000000000000000000 ),
 .UNSPECIFIED. ) ;
#4855=CARTESIAN_POINT ( 'NONE',  ( -239.6752751780977064, -1.974315850609194012, 11.58364238450984018 ) ) ;
#4859=CIRCLE ( 'NONE', #4638, 5.100000000000000533 ) ;
#4866=CARTESIAN_POINT ( 'NONE',  ( -249.7900429581053743, 11.65124970777654667, -1.521630442913122216 ) ) ;
#4875=CIRCLE ( 'NONE', #1473, 6.500000000000005329 ) ;
#4880=VERTEX_POINT ( 'NONE', #11537 ) ;
#4883=AXIS2_PLACEMENT_3D ( 'NONE', #9908, #781, #4830 ) ;
#4885=EDGE_LOOP ( 'NONE', ( #9916, #11045, #7637, #13004 ) ) ;
#4889=VERTEX_POINT ( 'NONE', #6667 ) ;
#4895=EDGE_CURVE ( 'NONE', #1370, #10870, #2320, .T. ) ;
#4899=CARTESIAN_POINT ( 'NONE',  ( -246.6527294682080367, 9.457576189755920737, -6.972573804798820163 ) ) ;
#4901=EDGE_CURVE ( 'NONE', #4811, #13033, #12540, .T. ) ;
#4902=DIRECTION ( 'NONE',  ( 1.000000000000000000, -0.000000000000000000, 1.224646799147353207E-16 ) ) ;
#4903=CARTESIAN_POINT ( 'NONE',  ( -122.2593324768321992, 18.00000000000000000, 168.2755348299905052 ) ) ;
#4906=CARTESIAN_POINT ( 'NONE',  ( -229.9847620420411261, 11.44809447175227035, 2.673990570740190975 ) ) ;
#4907=CARTESIAN_POINT ( 'NONE',  ( -195.0000000000000000, 30.00000000000000000, 0.000000000000000000 ) ) ;
#4916=CARTESIAN_POINT ( 'NONE',  ( -249.7841416270006789, -11.60584252727432109, -1.834925605625155498 ) ) ;
#4918=EDGE_CURVE ( 'NONE', #9610, #10870, #9583, .T. ) ;
#4920=EDGE_CURVE ( 'NONE', #789, #5629, #12658, .T. ) ;
#4921=CARTESIAN_POINT ( 'NONE',  ( -197.8197553893924976, 30.00000000000000000, -70.77553482998720824 ) ) ;
#4923=CARTESIAN_POINT ( 'NONE',  ( -248.0831933713610056, -9.830508068705260172, -6.436117704883899115 ) ) ;
#4925=CARTESIAN_POINT ( 'NONE',  ( -210.0000000000000000, 30.00000000000000000, -6.500000000000000000 ) ) ;
#4927=DIRECTION ( 'NONE',  ( 0.000000000000000000, -1.000000000000000000, 0.000000000000000000 ) ) ;
#4929=CARTESIAN_POINT ( 'NONE',  ( -229.7506357186298089, -4.852194303783566198, 10.70827597515549989 ) ) ;
#4932=ORIENTED_EDGE ( 'NONE', *, *, #375, .T. ) ;
#4934=CONICAL_SURFACE ( 'NONE', #2166, 6.500000000000005329, 0.7853981633974476129 ) ;
#4938=CIRCLE ( 'NONE', #2594, 6.500000000000005329 ) ;
#4940=CARTESIAN_POINT ( 'NONE',  ( 122.2593324768346008, 30.00000000000000000, 174.7755348299889988 ) ) ;
#4942=AXIS2_PLACEMENT_3D ( 'NONE', #2480, #9489, #1422 ) ;
#4943=CARTESIAN_POINT ( 'NONE',  ( -245.6300371773186839, -9.052739546058479192, 7.492707602925837485 ) ) ;
#4946=LINE ( 'NONE', #8228, #1056 ) ;
#4949=EDGE_LOOP ( 'NONE', ( #12527, #2687, #12338, #5350, #12115, #12543 ) ) ;
#4953=CARTESIAN_POINT ( 'NONE',  ( -249.1360723386881943, 10.36505329179906632, 5.534757212115697378 ) ) ;
#4957=CARTESIAN_POINT ( 'NONE',  ( -242.2371604624929944, 6.538578786594999137, 9.762666687128254139 ) ) ;
#4958=VERTEX_POINT ( 'NONE', #2646 ) ;
#4959=CARTESIAN_POINT ( 'NONE',  ( -239.1752428789251326, -1.444203915845354125, 11.66090825388631202 ) ) ;
#4960=AXIS2_PLACEMENT_3D ( 'NONE', #12824, #11835, #569 ) ;
#4962=EDGE_LOOP ( 'NONE', ( #3022, #12153, #5146, #1821 ) ) ;
#4964=DIRECTION ( 'NONE',  ( 0.000000000000000000, -1.000000000000000000, 0.000000000000000000 ) ) ;
#4965=ORIENTED_EDGE ( 'NONE', *, *, #3426, .F. ) ;
#4967=EDGE_CURVE ( 'NONE', #4005, #11054, #11651, .T. ) ;
#4969=DIRECTION ( 'NONE',  ( 0.000000000000000000, 0.000000000000000000, 1.000000000000000000 ) ) ;
#4971=DIRECTION ( 'NONE',  ( 0.000000000000000000, 1.000000000000000000, 0.000000000000000000 ) ) ;
#4978=DIRECTION ( 'NONE',  ( 0.000000000000000000, -1.000000000000000000, 0.000000000000000000 ) ) ;
#4980=TOROIDAL_SURFACE ( 'NONE', #5419, 247.7999999999999829, 2.000000000000000000 ) ;
#4981=ORIENTED_EDGE ( 'NONE', *, *, #7529, .T. ) ;
#4982=CARTESIAN_POINT ( 'NONE',  ( -248.8555022323135120, -10.14371006989313706, 5.930260236134023977 ) ) ;
#4986=CARTESIAN_POINT ( 'NONE',  ( 3.059167704270088292E-14, 0.000000000000000000, 249.7999999999999829 ) ) ;
#4990=CIRCLE ( 'NONE', #10742, 249.7999999999999829 ) ;
#4993=ADVANCED_FACE ( 'NONE', ( #6191 ), #2948, .F. ) ;
#4999=ORIENTED_EDGE ( 'NONE', *, *, #10537, .F. ) ;
#5004=DIRECTION ( 'NONE',  ( 0.000000000000000000, 1.000000000000000000, 0.000000000000000000 ) ) ;
#5007=CARTESIAN_POINT ( 'NONE',  ( -241.3329571118493959, -5.362363067942219175, 10.45502706639050672 ) ) ;
#5010=ORIENTED_EDGE ( 'NONE', *, *, #6579, .F. ) ;
#5012=DIRECTION ( 'NONE',  ( -0.000000000000000000, 1.000000000000000000, 0.000000000000000000 ) ) ;
#5015=ORIENTED_EDGE ( 'NONE', *, *, #1557, .T. ) ;
#5018=DIRECTION ( 'NONE',  ( 0.000000000000000000, -1.000000000000000000, 0.000000000000000000 ) ) ;
#5019=CARTESIAN_POINT ( 'NONE',  ( -249.5485775754664814, 10.89766932136149613, 4.396091617827336151 ) ) ;
#5023=CARTESIAN_POINT ( 'NONE',  ( -241.4114469334947444, 5.479936497169059173, 10.39393372328349585 ) ) ;
#5024=ORIENTED_EDGE ( 'NONE', *, *, #7704, .T. ) ;
#5025=CARTESIAN_POINT ( 'NONE',  ( -197.8197553893924976, 19.00000000000000000, -58.77553482998720114 ) ) ;
#5027=DIRECTION ( 'NONE',  ( 0.000000000000000000, 0.000000000000000000, -1.000000000000000000 ) ) ;
#5028=VERTEX_POINT ( 'NONE', #11391 ) ;
#5031=CARTESIAN_POINT ( 'NONE',  ( 239.0028278883971780, 0.3789072388907981925, 3.479912193141485144 ) ) ;
#5034=DIRECTION ( 'NONE',  ( 0.000000000000000000, 1.000000000000000000, 0.000000000000000000 ) ) ;
#5037=CARTESIAN_POINT ( 'NONE',  ( -239.1925639862890591, -1.468143820144465650, -11.65791905985560284 ) ) ;
#5038=EDGE_CURVE ( 'NONE', #12564, #2818, #1091, .T. ) ;
#5041=CARTESIAN_POINT ( 'NONE',  ( -249.3819455667575369, -10.64000139045997351, 4.985720160815903412 ) ) ;
#5042=ORIENTED_EDGE ( 'NONE', *, *, #3747, .F. ) ;
#5045=CARTESIAN_POINT ( 'NONE',  ( -245.4195491721955875, -8.949151682342847636, -7.614144253697441300 ) ) ;
#5051=CARTESIAN_POINT ( 'NONE',  ( -229.9990560493756107, -11.73156903894478376, 0.7633253822087937568 ) ) ;
#5052=EDGE_CURVE ( 'NONE', #6599, #1185, #4644, .T. ) ;
#5062=CARTESIAN_POINT ( 'NONE',  ( 239.1963018252558584, -1.024882057282255898, -3.346595946699232549 ) ) ;
#5067=CARTESIAN_POINT ( 'NONE',  ( -241.0175249738750551, -4.851820797546724684, 10.70187039113691085 ) ) ;
#5071=CARTESIAN_POINT ( 'NONE',  ( 229.9999987649675859, -3.499918840721679025, 0.2295273192198076240 ) ) ;
#5072=ORIENTED_EDGE ( 'NONE', *, *, #3621, .T. ) ;
#5073=ORIENTED_EDGE ( 'NONE', *, *, #10116, .F. ) ;
#5074=AXIS2_PLACEMENT_3D ( 'NONE', #1864, #1600, #9714 ) ;
#5076=CARTESIAN_POINT ( 'NONE',  ( 122.2593324768346008, 19.00000000000000000, 173.7755348299889988 ) ) ;
#5077=CONICAL_SURFACE ( 'NONE', #7213, 6.500000000000005329, 0.7853981633974476129 ) ;
#5078=ADVANCED_FACE ( 'NONE', ( #826 ), #11265, .T. ) ;
#5079=AXIS2_PLACEMENT_3D ( 'NONE', #159, #1158, #4347 ) ;
#5080=ADVANCED_FACE ( 'NONE', ( #6960 ), #2728, .T. ) ;
#5081=CONICAL_SURFACE ( 'NONE', #8708, 6.500000000000000000, 0.7853981633974518317 ) ;
#5085=CARTESIAN_POINT ( 'NONE',  ( -245.4148443365517949, 8.946846751025407940, 7.616852152958314193 ) ) ;
#5087=AXIS2_PLACEMENT_3D ( 'NONE', #7643, #7834, #11909 ) ;
#5088=EDGE_LOOP ( 'NONE', ( #1938, #5743, #5688, #6764 ) ) ;
#5089=DIRECTION ( 'NONE',  ( 0.000000000000000000, -1.000000000000000000, 0.000000000000000000 ) ) ;
#5090=ORIENTED_EDGE ( 'NONE', *, *, #6885, .T. ) ;
#5091=LINE ( 'NONE', #43, #9063 ) ;
#5093=TOROIDAL_SURFACE ( 'NONE', #3181, 250.0000000000000000, 10.00000000000000000 ) ;
#5096=CARTESIAN_POINT ( 'NONE',  ( 240.2193860686244022, 2.381856054652649934, 2.564741263481397304 ) ) ;
#5097=DIRECTION ( 'NONE',  ( 8.659560562354951347E-17, -0.7071067811865460184, 0.7071067811865489050 ) ) ;
#5099=AXIS2_PLACEMENT_3D ( 'NONE', #6655, #387, #1583 ) ;
#5101=CARTESIAN_POINT ( 'NONE',  ( 122.2593324768334071, 30.00000000000000000, -168.2755348299895104 ) ) ;
#5105=CARTESIAN_POINT ( 'NONE',  ( -238.7118990657748157, -0.07233802403633284028, -11.74979657428336211 ) ) ;
#5107=CARTESIAN_POINT ( 'NONE',  ( -249.2714863791366611, 10.50505558484134738, -5.263680432602310333 ) ) ;
#5111=CARTESIAN_POINT ( 'NONE',  ( -249.0239419977331750, -10.26696504969905277, 5.714577089209429417 ) ) ;
#5115=DIRECTION ( 'NONE',  ( 0.000000000000000000, 0.000000000000000000, 1.000000000000000000 ) ) ;
#5116=AXIS2_PLACEMENT_3D ( 'NONE', #2214, #6289, #10341 ) ;
#5117=CARTESIAN_POINT ( 'NONE',  ( -244.2656328536486967, -8.290010951899001057, -8.326962424612901259 ) ) ;
#5120=CARTESIAN_POINT ( 'NONE',  ( -229.7045047833707940, -1.539767244506014432, 11.65512487062059677 ) ) ;
#5122=ORIENTED_EDGE ( 'NONE', *, *, #4273, .F. ) ;
#5123=ORIENTED_EDGE ( 'NONE', *, *, #4433, .F. ) ;
#5125=DIRECTION ( 'NONE',  ( 0.000000000000000000, 0.000000000000000000, -1.000000000000000000 ) ) ;
#5130=DIRECTION ( 'NONE',  ( 0.000000000000000000, 1.000000000000000000, 0.000000000000000000 ) ) ;
#5131=DIRECTION ( 'NONE',  ( 0.000000000000000000, 0.000000000000000000, 1.000000000000000000 ) ) ;
#5136=CARTESIAN_POINT ( 'NONE',  ( -243.1363860133195089, -7.429686608487776844, 9.102873391554766158 ) ) ;
#5141=CARTESIAN_POINT ( 'NONE',  ( 0.000000000000000000, 19.00000000000000000, 213.5000000000000000 ) ) ;
#5142=CARTESIAN_POINT ( 'NONE',  ( 229.9884266870191709, -2.636753545538539800, 2.312936221645658819 ) ) ;
#5144=ORIENTED_EDGE ( 'NONE', *, *, #4273, .T. ) ;
#5146=ORIENTED_EDGE ( 'NONE', *, *, #10265, .T. ) ;
#5150=AXIS2_PLACEMENT_3D ( 'NONE', #4686, #10763, #10964 ) ;
#5151=CARTESIAN_POINT ( 'NONE',  ( -241.3664650619784311, 5.412961098280363537, 10.42892899847316102 ) ) ;
#5154=EDGE_CURVE ( 'NONE', #7072, #6121, #1891, .T. ) ;
#5157=DIRECTION ( 'NONE',  ( 0.000000000000000000, -1.000000000000000000, 0.000000000000000000 ) ) ;
#5162=CARTESIAN_POINT ( 'NONE',  ( 239.2711857406566764, 1.179132569667092456, 3.296284915102607904 ) ) ;
#5167=AXIS2_PLACEMENT_3D ( 'NONE', #4335, #2268, #1278 ) ;
#5170=CIRCLE ( 'NONE', #10716, 6.500000000000005329 ) ;
#5171=DIRECTION ( 'NONE',  ( 0.000000000000000000, 0.000000000000000000, 1.000000000000000000 ) ) ;
#5174=CARTESIAN_POINT ( 'NONE',  ( 122.2593324768334071, 30.00000000000000000, -173.7755348299895104 ) ) ;
#5176=CARTESIAN_POINT ( 'NONE',  ( -249.7266004377088393, -11.33448610411373991, 3.100135290851260272 ) ) ;
#5178=AXIS2_PLACEMENT_3D ( 'NONE', #5844, #3895, #1840 ) ;
#5182=CARTESIAN_POINT ( 'NONE',  ( -239.5361044668155159, 1.848645179572584896, 11.60366368868220022 ) ) ;
#5183=CARTESIAN_POINT ( 'NONE',  ( -245.4623802705897333, -8.970018889905636783, -7.589566413994238481 ) ) ;
#5185=CARTESIAN_POINT ( 'NONE',  ( 239.4068548683480628, -1.402387639798359231, 3.207804078318175378 ) ) ;
#5193=ORIENTED_EDGE ( 'NONE', *, *, #956, .T. ) ;
#5194=CIRCLE ( 'NONE', #6914, 6.500000000000005329 ) ;
#5199=VECTOR ( 'NONE', #6343, 1000.000000000000000 ) ;
#5202=CARTESIAN_POINT ( 'NONE',  ( 0.000000000000000000, 0.000000000000000000, -249.7999999999999829 ) ) ;
#5203=CARTESIAN_POINT ( 'NONE',  ( 71.82423009839129691, 18.00000000000000000, -190.8354503650405150 ) ) ;
#5204=DIRECTION ( 'NONE',  ( 0.000000000000000000, -1.000000000000000000, 0.000000000000000000 ) ) ;
#5207=VERTEX_POINT ( 'NONE', #8135 ) ;
#5208=CARTESIAN_POINT ( 'NONE',  ( 197.8197553893920144, 18.00000000000000000, 64.27553482998850143 ) ) ;
#5212=CARTESIAN_POINT ( 'NONE',  ( 229.9948716278398706, -3.146202118422226413, 1.550284843520935762 ) ) ;
#5213=ORIENTED_EDGE ( 'NONE', *, *, #10627, .T. ) ;
#5218=CONICAL_SURFACE ( 'NONE', #9282, 5.100000000000000533, 0.7853981633974503884 ) ;
#5222=CARTESIAN_POINT ( 'NONE',  ( -246.9758887651909163, 9.561393940552608939, 6.829510940766356342 ) ) ;
#5224=DIRECTION ( 'NONE',  ( 0.000000000000000000, 0.000000000000000000, 1.000000000000000000 ) ) ;
#5232=CIRCLE ( 'NONE', #9918, 5.500000000000005329 ) ;
#5234=DIRECTION ( 'NONE',  ( 0.000000000000000000, 1.000000000000000000, 0.000000000000000000 ) ) ;
#5236=EDGE_CURVE ( 'NONE', #12366, #12887, #9554, .T. ) ;
#5242=ORIENTED_EDGE ( 'NONE', *, *, #135, .F. ) ;
#5246=DIRECTION ( 'NONE',  ( 0.000000000000000000, 0.000000000000000000, 1.000000000000000000 ) ) ;
#5248=CARTESIAN_POINT ( 'NONE',  ( -249.7845036514944468, -11.60839712336035845, 1.818694302480377889 ) ) ;
#5249=EDGE_LOOP ( 'NONE', ( #10152, #4694, #2749, #4611 ) ) ;
#5252=DIRECTION ( 'NONE',  ( 0.000000000000000000, 0.000000000000000000, -1.000000000000000000 ) ) ;
#5254=EDGE_CURVE ( 'NONE', #7121, #10886, #3367, .T. ) ;
#5255=CARTESIAN_POINT ( 'NONE',  ( -242.2371604626287649, -6.538578786747162752, -9.762666687019821765 ) ) ;
#5257=CARTESIAN_POINT ( 'NONE',  ( 238.9743709119342441, -0.1785824616379369512, 3.500006748982332994 ) ) ;
#5259=CARTESIAN_POINT ( 'NONE',  ( 240.5832516929813494, 3.370511182575330000, -0.9484507949093432533 ) ) ;
#5261=DIRECTION ( 'NONE',  ( 0.000000000000000000, 1.000000000000000000, 0.000000000000000000 ) ) ;
#5263=AXIS2_PLACEMENT_3D ( 'NONE', #7726, #3924, #7998 ) ;
#5266=CARTESIAN_POINT ( 'NONE',  ( -249.6767732310727865, 11.18100465983052949, 3.612153022792313095 ) ) ;
#5267=LINE ( 'NONE', #9338, #6176 ) ;
#5273=CARTESIAN_POINT ( 'NONE',  ( -246.4294064422139741, -9.379184893293130543, 7.077828147970874006 ) ) ;
#5276=CARTESIAN_POINT ( 'NONE',  ( 71.82423009839129691, 19.40000000000000213, -197.3354503650404865 ) ) ;
#5277=DIRECTION ( 'NONE',  ( 0.000000000000000000, 1.000000000000000000, 0.000000000000000000 ) ) ;
#5278=ORIENTED_EDGE ( 'NONE', *, *, #12634, .F. ) ;
#5280=FACE_OUTER_BOUND ( 'NONE', #10273, .T. ) ;
#5288=AXIS2_PLACEMENT_3D ( 'NONE', #10485, #421, #224 ) ;
#5289=CIRCLE ( 'NONE', #6577, 249.7999999999999829 ) ;
#5292=CIRCLE ( 'NONE', #3797, 240.3921568627449687 ) ;
#5294=ORIENTED_EDGE ( 'NONE', *, *, #12898, .F. ) ;
#5297=VECTOR ( 'NONE', #5795, 1000.000000000000000 ) ;
#5301=ADVANCED_FACE ( 'NONE', ( #5280 ), #5724, .F. ) ;
#5302=EDGE_CURVE ( 'NONE', #5843, #11287, #3586, .T. ) ;
#5305=CARTESIAN_POINT ( 'NONE',  ( -197.8197553893909912, 30.00000000000000000, 64.27553482999130097 ) ) ;
#5311=DIRECTION ( 'NONE',  ( 0.000000000000000000, 1.000000000000000000, 0.000000000000000000 ) ) ;
#5313=CARTESIAN_POINT ( 'NONE',  ( -248.0831933713610056, 9.830508068705238856, -6.436117704883929314 ) ) ;
#5314=DIRECTION ( 'NONE',  ( 0.000000000000000000, 0.7071067811865470176, 0.7071067811865480168 ) ) ;
#5316=DIRECTION ( 'NONE',  ( 0.000000000000000000, 1.000000000000000000, 0.000000000000000000 ) ) ;
#5318=CIRCLE ( 'NONE', #433, 6.500000000000005329 ) ;
#5322=CARTESIAN_POINT ( 'NONE',  ( -243.2136795283335857, -7.496740008778170150, -9.047741638628279404 ) ) ;
#5323=CIRCLE ( 'NONE', #9787, 5.500000000000005329 ) ;
#5324=CARTESIAN_POINT ( 'NONE',  ( 239.3580835733109495, -1.327753754010405851, 3.239279126423496802 ) ) ;
#5326=CARTESIAN_POINT ( 'NONE',  ( 240.4516407507319400, 2.994726891335696806, 1.822055168078867471 ) ) ;
#5329=AXIS2_PLACEMENT_3D ( 'NONE', #9418, #2143, #216 ) ;
#5331=VERTEX_POINT ( 'NONE', #8232 ) ;
#5336=CARTESIAN_POINT ( 'NONE',  ( 239.3359268379452658, -1.289900281489894995, -3.253812819841678472 ) ) ;
#5344=ORIENTED_EDGE ( 'NONE', *, *, #1742, .T. ) ;
#5345=DIRECTION ( 'NONE',  ( 0.000000000000000000, 1.000000000000000000, 0.000000000000000000 ) ) ;
#5346=DIRECTION ( 'NONE',  ( 0.000000000000000000, -1.000000000000000000, 0.000000000000000000 ) ) ;
#5348=B_SPLINE_CURVE_WITH_KNOTS ( 'NONE', 3,
 ( #10774, #580, #843, #8710, #12839, #10975, #3833, #1846, #11844, #4828, #13039, #12772, #11033 ),
 .UNSPECIFIED., .F., .F.,
 ( 4, 2, 2, 1, 2, 2, 4 ),
 ( 0.000000000000000000, 0.2499999999999983347, 0.3749999999999975020, 0.4374999999999973910, 0.4687499999999859002, 0.4999999999999743538, 1.000000000000000000 ),
 .UNSPECIFIED. ) ;
#5349=CARTESIAN_POINT ( 'NONE',  ( 229.9750547325863010, -0.9088897890003139191, -3.387654320631149130 ) ) ;
#5350=ORIENTED_EDGE ( 'NONE', *, *, #5637, .T. ) ;
#5351=ORIENTED_EDGE ( 'NONE', *, *, #2286, .T. ) ;
#5353=DIRECTION ( 'NONE',  ( 0.000000000000000000, 0.000000000000000000, 1.000000000000000000 ) ) ;
#5355=AXIS2_PLACEMENT_3D ( 'NONE', #8313, #4100, #12372 ) ;
#5357=FACE_OUTER_BOUND ( 'NONE', #7772, .T. ) ;
#5358=FACE_OUTER_BOUND ( 'NONE', #131, .T. ) ;
#5361=ORIENTED_EDGE ( 'NONE', *, *, #6936, .T. ) ;
#5363=ORIENTED_EDGE ( 'NONE', *, *, #9006, .F. ) ;
#5365=ORIENTED_EDGE ( 'NONE', *, *, #9538, .F. ) ;
#5369=CARTESIAN_POINT ( 'NONE',  ( -122.2593324768359935, 30.00000000000000000, -168.2755348299880040 ) ) ;
#5371=CARTESIAN_POINT ( 'NONE',  ( 239.6582758818212540, 1.713542963916843131, -3.052483991371184757 ) ) ;
#5372=CARTESIAN_POINT ( 'NONE',  ( -122.2593324768359935, 19.00000000000000000, -168.2755348299880040 ) ) ;
#5375=CONICAL_SURFACE ( 'NONE', #4724, 5.099999999999993427, 0.7853981633974461696 ) ;
#5377=ORIENTED_EDGE ( 'NONE', *, *, #11829, .F. ) ;
#5379=TOROIDAL_SURFACE ( 'NONE', #7712, 238.4705882352940307, 2.000000000000000000 ) ;
#5385=EDGE_CURVE ( 'NONE', #4744, #9610, #4223, .T. ) ;
#5387=EDGE_LOOP ( 'NONE', ( #7812, #1219, #2213, #1544 ) ) ;
#5392=CARTESIAN_POINT ( 'NONE',  ( 0.000000000000000000, 25.00000000000000000, -245.7999999999999829 ) ) ;
#5396=AXIS2_PLACEMENT_3D ( 'NONE', #6637, #6768, #8962 ) ;
#5398=CARTESIAN_POINT ( 'NONE',  ( 122.2593324768346008, 19.00000000000000000, 168.2755348299889988 ) ) ;
#5399=AXIS2_PLACEMENT_3D ( 'NONE', #3744, #11824, #10681 ) ;
#5407=AXIS2_PLACEMENT_3D ( 'NONE', #11297, #5089, #4290 ) ;
#5408=ADVANCED_FACE ( 'NONE', ( #223 ), #7413, .F. ) ;
#5409=DIRECTION ( 'NONE',  ( 0.000000000000000000, 0.000000000000000000, -1.000000000000000000 ) ) ;
#5412=DIRECTION ( 'NONE',  ( 0.000000000000000000, 0.000000000000000000, 1.000000000000000000 ) ) ;
#5415=CARTESIAN_POINT ( 'NONE',  ( 240.6325187087389565, -3.500040777417273041, 0.1929172344771862835 ) ) ;
#5417=EDGE_LOOP ( 'NONE', ( #10849, #11876, #8191, #1792 ) ) ;
#5419=AXIS2_PLACEMENT_3D ( 'NONE', #10200, #1072, #5131 ) ;
#5421=LINE ( 'NONE', #9484, #5470 ) ;
#5427=DIRECTION ( 'NONE',  ( 0.000000000000000000, -1.000000000000000000, 0.000000000000000000 ) ) ;
#5429=CIRCLE ( 'NONE', #8556, 240.3921568627449687 ) ;
#5430=ORIENTED_EDGE ( 'NONE', *, *, #11663, .T. ) ;
#5433=ORIENTED_EDGE ( 'NONE', *, *, #4371, .F. ) ;
#5434=DIRECTION ( 'NONE',  ( 0.000000000000000000, 1.000000000000000000, 0.000000000000000000 ) ) ;
#5436=ORIENTED_EDGE ( 'NONE', *, *, #3627, .T. ) ;
#5439=CARTESIAN_POINT ( 'NONE',  ( 71.82423009839129691, 28.60000000000000142, 202.4354503650404808 ) ) ;
#5440=DIRECTION ( 'NONE',  ( 0.000000000000000000, 0.000000000000000000, 1.000000000000000000 ) ) ;
#5441=CARTESIAN_POINT ( 'NONE',  ( -238.7109915775760669, 0.006370638632528863136, -11.75000000064824768 ) ) ;
#5443=ORIENTED_EDGE ( 'NONE', *, *, #4183, .F. ) ;
#5445=CIRCLE ( 'NONE', #7999, 5.099999999999993427 ) ;
#5446=VERTEX_POINT ( 'NONE', #10414 ) ;
#5447=DIRECTION ( 'NONE',  ( 0.000000000000000000, 0.000000000000000000, 1.000000000000000000 ) ) ;
#5453=CARTESIAN_POINT ( 'NONE',  ( -241.3664650619595022, -5.412961098251741987, -10.42892899848466115 ) ) ;
#5459=B_SPLINE_CURVE_WITH_KNOTS ( 'NONE', 3,
 ( #6890, #6760, #12746, #9941, #5619, #12943, #7680, #1686, #760, #9809, #8819, #8880, #6823 ),
 .UNSPECIFIED., .F., .F.,
 ( 4, 2, 2, 1, 2, 2, 4 ),
 ( 0.000000000000000000, 0.2499999999999875655, 0.3749999999999813483, 0.4374999999999648614, 0.4687499999999565903, 0.4999999999999483191, 1.000000000000000000 ),
 .UNSPECIFIED. ) ;
#5460=DIRECTION ( 'NONE',  ( 0.000000000000000000, 0.000000000000000000, 1.000000000000000000 ) ) ;
#5467=EDGE_CURVE ( 'NONE', #6909, #6421, #6158, .T. ) ;
#5470=VECTOR ( 'NONE', #5545, 1000.000000000000114 ) ;
#5472=CARTESIAN_POINT ( 'NONE',  ( -246.2764285590020279, -9.322503223484712720, 7.152604638120487301 ) ) ;
#5473=CARTESIAN_POINT ( 'NONE',  ( 197.8197553893915028, 19.00000000000000000, -64.27553482998990830 ) ) ;
#5476=ORIENTED_EDGE ( 'NONE', *, *, #12187, .T. ) ;
#5482=DIRECTION ( 'NONE',  ( 0.000000000000000000, 0.000000000000000000, 1.000000000000000000 ) ) ;
#5485=CARTESIAN_POINT ( 'NONE',  ( -122.2593324768359935, 19.00000000000000000, -168.2755348299880040 ) ) ;
#5487=ORIENTED_EDGE ( 'NONE', *, *, #2369, .F. ) ;
#5490=CARTESIAN_POINT ( 'NONE',  ( -210.0000000000000000, 30.00000000000000000, 0.000000000000000000 ) ) ;
#5493=EDGE_CURVE ( 'NONE', #11582, #158, #1417, .T. ) ;
#5496=DIRECTION ( 'NONE',  ( 0.000000000000000000, -1.000000000000000000, 0.000000000000000000 ) ) ;
#5498=LINE ( 'NONE', #12635, #11553 ) ;
#5500=DIRECTION ( 'NONE',  ( 0.000000000000000000, 0.000000000000000000, 1.000000000000000000 ) ) ;
#5501=CIRCLE ( 'NONE', #7204, 5.500000000000005329 ) ;
#5505=ORIENTED_EDGE ( 'NONE', *, *, #1165, .T. ) ;
#5506=VECTOR ( 'NONE', #483, 1000.000000000000000 ) ;
#5507=CARTESIAN_POINT ( 'NONE',  ( -122.2593324768359935, 30.00000000000000000, -161.7755348299880040 ) ) ;
#5509=CARTESIAN_POINT ( 'NONE',  ( 71.82423009839129691, 28.60000000000000142, 197.3354503650404865 ) ) ;
#5511=B_SPLINE_CURVE_WITH_KNOTS ( 'NONE', 3,
 ( #9751, #1701, #3757, #7822, #638, #11896, #772, #2759, #3146, #2029, #5222, #3959, #1026, #11294, #12162, #7692, #899, #12293, #4023, #7296, #2087, #8101, #2951, #9231, #3015, #9294, #6100, #11094, #5085, #8031, #9160, #36, #3216, #12363, #2224, #7098, #4157, #12093, #10151, #8238, #1962, #1094, #102, #4218, #11364, #8303, #9096, #6037, #11160, #7233, #4090, #6303, #166, #8170, #10092, #3086, #4957, #12231, #7164, #9034, #7033, #2158, #11223, #6166, #966, #5023, #10220, #6236, #5151, #10288, #1163, #2547, #1424, #10617, #2420, #12488, #12430, #4287, #362, #9362, #1226 ),
 .UNSPECIFIED., .F., .F.,
 ( 4, 1, 1, 1, 2, 2, 2, 1, 1, 1, 2, 2, 2, 2, 1, 1, 1, 1, 2, 2, 2, 2, 1, 1, 1, 2, 2, 2, 1, 1, 1, 2, 2, 2, 2, 1, 1, 1, 2, 2, 2, 1, 1, 1, 2, 2, 2, 1, 1, 1, 2, 2, 4 ),
 ( 0.000000000000000000, 0.03124999999994631378, 0.04687499999991946720, 0.05468749999990599880, 0.05859374999989923338, 0.06249999999989246796, 0.09374999999987096433, 0.1093749999998601952, 0.1171874999998548522, 0.1210937499998521738, 0.1230468749998536865, 0.1249999999998551992, 0.1875000000000294764, 0.2187500000001137146, 0.2343750000001531830, 0.2421875000001753597, 0.2460937500001839640, 0.2480468750001859068, 0.2490234375001867950, 0.2500000000001876832, 0.3125000000001743050, 0.3437500000001676437, 0.3593750000001619815, 0.3671875000001592615, 0.3710937500001600386, 0.3730468750001624811, 0.3750000000001648681, 0.4375000000001639244, 0.4687500000001658118, 0.4843750000001668665, 0.4921875000001651457, 0.4960937500001642575, 0.5000000000001634248, 0.5625000000001737499, 0.5937500000001809664, 0.6093750000001847411, 0.6171875000001865175, 0.6210937500001851852, 0.6230468750001870726, 0.6250000000001889600, 0.6875000000001727507, 0.7187500000001628697, 0.7343750000001598721, 0.7421875000001600942, 0.7460937500001600942, 0.7500000000001599831, 0.8125000000001328937, 0.8437500000001192380, 0.8593750000001121325, 0.8671875000001085798, 0.8710937500001052491, 0.8750000000001018075, 1.000000000000000000 ),
 .UNSPECIFIED. ) ;
#5515=LINE ( 'NONE', #2693, #7899 ) ;
#5525=DIRECTION ( 'NONE',  ( 0.000000000000000000, 0.000000000000000000, -1.000000000000000000 ) ) ;
#5528=CARTESIAN_POINT ( 'NONE',  ( 0.000000000000000000, 0.000000000000000000, 0.000000000000000000 ) ) ;
#5531=CIRCLE ( 'NONE', #11061, 239.8169934640564804 ) ;
#5532=FACE_BOUND ( 'NONE', #12490, .T. ) ;
#5535=CARTESIAN_POINT ( 'NONE',  ( -229.7148377869573608, -2.666494325112176433, -11.44984222230669069 ) ) ;
#5537=CARTESIAN_POINT ( 'NONE',  ( 0.000000000000000000, 18.00000000000000000, 0.000000000000000000 ) ) ;
#5539=ORIENTED_EDGE ( 'NONE', *, *, #10116, .T. ) ;
#5541=ORIENTED_EDGE ( 'NONE', *, *, #9993, .T. ) ;
#5542=EDGE_CURVE ( 'NONE', #6354, #6448, #3998, .T. ) ;
#5545=DIRECTION ( 'NONE',  ( 8.659560562354913137E-17, -0.7071067811865489050, 0.7071067811865460184 ) ) ;
#5548=LINE ( 'NONE', #9806, #11571 ) ;
#5550=DIRECTION ( 'NONE',  ( 0.000000000000000000, -1.000000000000000000, 0.000000000000000000 ) ) ;
#5554=FACE_OUTER_BOUND ( 'NONE', #2599, .T. ) ;
#5555=ORIENTED_EDGE ( 'NONE', *, *, #3335, .F. ) ;
#5556=DIRECTION ( 'NONE',  ( 0.000000000000000000, 0.000000000000000000, 1.000000000000000000 ) ) ;
#5559=CARTESIAN_POINT ( 'NONE',  ( 0.000000000000000000, 0.000000000000000000, 0.000000000000000000 ) ) ;
#5563=CARTESIAN_POINT ( 'NONE',  ( 239.0530249120305371, 0.6193663070761113998, -3.444815813553090411 ) ) ;
#5564=CARTESIAN_POINT ( 'NONE',  ( -238.7118983370134799, 0.07231316710876492526, -11.74979690964867807 ) ) ;
#5565=( NAMED_UNIT ( * ) SI_UNIT ( $, .STERADIAN. ) SOLID_ANGLE_UNIT ( ) );
#5566=CARTESIAN_POINT ( 'NONE',  ( 0.000000000000000000, 30.00000000000000000, 0.000000000000000000 ) ) ;
#5568=EDGE_CURVE ( 'NONE', #1635, #6293, #2367, .T. ) ;
#5573=CARTESIAN_POINT ( 'NONE',  ( -243.1551830321994316, 7.446108171819295407, -9.089443071765307636 ) ) ;
#5574=CARTESIAN_POINT ( 'NONE',  ( 0.000000000000000000, -9.830508068699650437, 0.000000000000000000 ) ) ;
#5575=VECTOR ( 'NONE', #11377, 1000.000000000000114 ) ;
#5580=CARTESIAN_POINT ( 'NONE',  ( -240.7431671956743173, -4.340241521192577778, -10.91924886806390838 ) ) ;
#5586=AXIS2_PLACEMENT_3D ( 'NONE', #11575, #2432, #6514 ) ;
#5591=ORIENTED_EDGE ( 'NONE', *, *, #10968, .F. ) ;
#5592=TOROIDAL_SURFACE ( 'NONE', #8791, 241.5000000000000000, 2.500000000000000000 ) ;
#5595=FACE_OUTER_BOUND ( 'NONE', #12154, .T. ) ;
#5596=FACE_OUTER_BOUND ( 'NONE', #7297, .T. ) ;
#5600=CARTESIAN_POINT ( 'NONE',  ( 0.000000000000000000, 0.000000000000000000, 0.000000000000000000 ) ) ;
#5602=CIRCLE ( 'NONE', #10281, 239.0000000000000000 ) ;
#5604=CARTESIAN_POINT ( 'NONE',  ( -229.8108972436801594, -7.155453164010755707, -9.328021014420249557 ) ) ;
#5607=VECTOR ( 'NONE', #8625, 1000.000000000000000 ) ;
#5612=CARTESIAN_POINT ( 'NONE',  ( 122.2593324768334071, 29.00000000000000000, -168.2755348299895104 ) ) ;
#5614=AXIS2_PLACEMENT_3D ( 'NONE', #1209, #1142, #345 ) ;
#5616=CARTESIAN_POINT ( 'NONE',  ( -239.5361044668159991, -1.848645179572815156, -11.60366368868215758 ) ) ;
#5618=CARTESIAN_POINT ( 'NONE',  ( 0.000000000000000000, -1.848645179579245124, 0.000000000000000000 ) ) ;
#5619=CARTESIAN_POINT ( 'NONE',  ( 240.0731061099968429, 2.151402440697789853, -2.761193928003757847 ) ) ;
#5621=ORIENTED_EDGE ( 'NONE', *, *, #4895, .T. ) ;
#5623=VECTOR ( 'NONE', #6710, 1000.000000000000114 ) ;
#5627=ORIENTED_EDGE ( 'NONE', *, *, #3655, .F. ) ;
#5629=VERTEX_POINT ( 'NONE', #6619 ) ;
#5630=DIRECTION ( 'NONE',  ( 0.000000000000000000, 0.000000000000000000, 1.000000000000000000 ) ) ;
#5634=CARTESIAN_POINT ( 'NONE',  ( 0.000000000000000000, 0.000000000000000000, 0.000000000000000000 ) ) ;
#5637=EDGE_CURVE ( 'NONE', #3848, #5028, #8055, .T. ) ;
#5639=ORIENTED_EDGE ( 'NONE', *, *, #4433, .T. ) ;
#5640=CARTESIAN_POINT ( 'NONE',  ( -238.9974237869947444, -1.159187598540258213, 11.69290073402236985 ) ) ;
#5641=ORIENTED_EDGE ( 'NONE', *, *, #306, .T. ) ;
#5642=LINE ( 'NONE', #1445, #4789 ) ;
#5643=VERTEX_POINT ( 'NONE', #553 ) ;
#5644=EDGE_CURVE ( 'NONE', #6599, #6354, #8675, .T. ) ;
#5648=CARTESIAN_POINT ( 'NONE',  ( -229.9254091646820370, 10.19501318499466613, 5.891900222926529374 ) ) ;
#5654=DIRECTION ( 'NONE',  ( 0.000000000000000000, -1.000000000000000000, 0.000000000000000000 ) ) ;
#5656=ORIENTED_EDGE ( 'NONE', *, *, #9595, .F. ) ;
#5657=CARTESIAN_POINT ( 'NONE',  ( -249.7994671773518292, -11.75014634419642512, 0.3782188002307603214 ) ) ;
#5659=ADVANCED_FACE ( 'NONE', ( #10743 ), #7415, .F. ) ;
#5661=EDGE_CURVE ( 'NONE', #10688, #10559, #2091, .T. ) ;
#5667=FACE_OUTER_BOUND ( 'NONE', #6276, .T. ) ;
#5669=CARTESIAN_POINT ( 'NONE',  ( 229.9973455135990719, 3.322144853712378332, 1.125217561599514582 ) ) ;
#5670=CARTESIAN_POINT ( 'NONE',  ( -249.6369960391239431, 11.07262528784599986, -3.948341302959084143 ) ) ;
#5678=CARTESIAN_POINT ( 'NONE',  ( -122.2593324768359935, 30.00000000000000000, -173.7755348299880040 ) ) ;
#5685=DIRECTION ( 'NONE',  ( 0.000000000000000000, 0.000000000000000000, 1.000000000000000000 ) ) ;
#5686=ORIENTED_EDGE ( 'NONE', *, *, #11342, .T. ) ;
#5688=ORIENTED_EDGE ( 'NONE', *, *, #12273, .F. ) ;
#5694=VECTOR ( 'NONE', #12843, 1000.000000000000000 ) ;
#5695=DIRECTION ( 'NONE',  ( 0.000000000000000000, 0.000000000000000000, -1.000000000000000000 ) ) ;
#5697=CYLINDRICAL_SURFACE ( 'NONE', #4557, 5.499999999999998224 ) ;
#5698=SHAPE_REPRESENTATION_RELATIONSHIP ( 'NONE' , 'NONE' ,  #11156, #12065 ) ;
#5699=DIRECTION ( 'NONE',  ( 0.000000000000000000, 0.000000000000000000, 1.000000000000000000 ) ) ;
#5700=ORIENTED_EDGE ( 'NONE', *, *, #11027, .T. ) ;
#5703=CARTESIAN_POINT ( 'NONE',  ( -241.2893272559224158, 5.295647552975790262, -10.48903809278043120 ) ) ;
#5705=EDGE_CURVE ( 'NONE', #7072, #497, #3151, .T. ) ;
#5716=DIRECTION ( 'NONE',  ( 0.000000000000000000, 1.000000000000000000, 0.000000000000000000 ) ) ;
#5720=ORIENTED_EDGE ( 'NONE', *, *, #8795, .T. ) ;
#5721=CARTESIAN_POINT ( 'NONE',  ( -248.2181897918291895, -9.855491095783875721, -6.397958699636017599 ) ) ;
#5724=CONICAL_SURFACE ( 'NONE', #10404, 5.099999999999993427, 0.7853981633974461696 ) ;
#5727=DIRECTION ( 'NONE',  ( 0.000000000000000000, -1.000000000000000000, 0.000000000000000000 ) ) ;
#5728=AXIS2_PLACEMENT_3D ( 'NONE', #12337, #1267, #9070 ) ;
#5731=AXIS2_PLACEMENT_3D ( 'NONE', #2758, #11846, #9699 ) ;
#5732=FACE_OUTER_BOUND ( 'NONE', #10428, .T. ) ;
#5735=CARTESIAN_POINT ( 'NONE',  ( 229.9748299376111333, 0.9217590672928105411, 3.407079461714101143 ) ) ;
#5738=CARTESIAN_POINT ( 'NONE',  ( -248.5980333530941380, 9.980365686252888224, -6.207212897962511633 ) ) ;
#5739=CARTESIAN_POINT ( 'NONE',  ( 0.000000000000000000, 30.00000000000000000, -208.0000000000000000 ) ) ;
#5743=ORIENTED_EDGE ( 'NONE', *, *, #1850, .T. ) ;
#5746=DIRECTION ( 'NONE',  ( 0.000000000000000000, -1.000000000000000000, 0.000000000000000000 ) ) ;
#5747=AXIS2_PLACEMENT_3D ( 'NONE', #4439, #6393, #4313 ) ;
#5749=FACE_OUTER_BOUND ( 'NONE', #1907, .T. ) ;
#5751=CARTESIAN_POINT ( 'NONE',  ( 122.2593324768334071, 19.00000000000000000, -168.2755348299895104 ) ) ;
#5754=EDGE_CURVE ( 'NONE', #171, #8155, #7803, .T. ) ;
#5763=CIRCLE ( 'NONE', #5116, 6.500000000000005329 ) ;
#5764=DIRECTION ( 'NONE',  ( 0.000000000000000000, 0.7071067811865570096, 0.7071067811865380248 ) ) ;
#5765=CARTESIAN_POINT ( 'NONE',  ( 238.9937144808761502, -0.3120165755701557186, -3.486321029136065786 ) ) ;
#5767=ORIENTED_EDGE ( 'NONE', *, *, #2955, .T. ) ;
#5772=CARTESIAN_POINT ( 'NONE',  ( -241.3329571118387946, 5.362363067925850935, -10.45502706639501334 ) ) ;
#5774=CIRCLE ( 'NONE', #6638, 6.500000000000005329 ) ;
#5775=CARTESIAN_POINT ( 'NONE',  ( -249.3500139047620223, -10.59807002899673911, 5.074486595336709094 ) ) ;
#5776=AXIS2_PLACEMENT_3D ( 'NONE', #8395, #2382, #4568 ) ;
#5780=CARTESIAN_POINT ( 'NONE',  ( -229.7197566492325222, 3.060063085356466317, -11.35103441395172119 ) ) ;
#5781=AXIS2_PLACEMENT_3D ( 'NONE', #3225, #8245, #6851 ) ;
#5784=VERTEX_POINT ( 'NONE', #10994 ) ;
#5787=ORIENTED_EDGE ( 'NONE', *, *, #9412, .T. ) ;
#5789=EDGE_CURVE ( 'NONE', #9651, #12366, #2793, .T. ) ;
#5790=VERTEX_POINT ( 'NONE', #11944 ) ;
#5791=ORIENTED_EDGE ( 'NONE', *, *, #8978, .F. ) ;
#5792=CARTESIAN_POINT ( 'NONE',  ( -249.2564709991243603, -10.48830713239226320, -5.296988132951380379 ) ) ;
#5795=DIRECTION ( 'NONE',  ( 0.000000000000000000, 0.7071067811865480168, 0.7071067811865470176 ) ) ;
#5799=DIRECTION ( 'NONE',  ( 0.000000000000000000, -1.000000000000000000, 0.000000000000000000 ) ) ;
#5802=CARTESIAN_POINT ( 'NONE',  ( 0.000000000000000000, 30.00000000000000000, -208.0000000000000000 ) ) ;
#5804=CARTESIAN_POINT ( 'NONE',  ( 0.000000000000000000, 18.00000000000000000, -214.5000000000000000 ) ) ;
#5808=CARTESIAN_POINT ( 'NONE',  ( -249.7843163504555548, 11.60707272978753757, 1.827122155623386091 ) ) ;
#5811=EDGE_LOOP ( 'NONE', ( #9920, #2747, #5072, #2933 ) ) ;
#5812=VERTEX_POINT ( 'NONE', #9801 ) ;
#5822=CARTESIAN_POINT ( 'NONE',  ( -122.2593324768359935, 30.00000000000000000, -174.7755348299880040 ) ) ;
#5823=AXIS2_PLACEMENT_3D ( 'NONE', #8163, #11289, #12227 ) ;
#5827=ORIENTED_EDGE ( 'NONE', *, *, #8326, .F. ) ;
#5828=ORIENTED_EDGE ( 'NONE', *, *, #4967, .T. ) ;
#5831=B_SPLINE_CURVE_WITH_KNOTS ( 'NONE', 3,
 ( #5616, #10746, #1683, #7876 ),
 .UNSPECIFIED., .F., .F.,
 ( 4, 4 ),
 ( 0.000000000000000000, 1.000000000000000000 ),
 .UNSPECIFIED. ) ;
#5838=CARTESIAN_POINT ( 'NONE',  ( 71.82423009839129691, 30.00000000000000000, -197.3354503650404865 ) ) ;
#5839=DIRECTION ( 'NONE',  ( -0.000000000000000000, 1.000000000000000000, 0.000000000000000000 ) ) ;
#5841=CIRCLE ( 'NONE', #5178, 195.0000000000000000 ) ;
#5843=VERTEX_POINT ( 'NONE', #6005 ) ;
#5844=CARTESIAN_POINT ( 'NONE',  ( 0.000000000000000000, 29.00000000000000000, 0.000000000000000000 ) ) ;
#5845=VERTEX_POINT ( 'NONE', #6869 ) ;
#5846=CARTESIAN_POINT ( 'NONE',  ( -238.7779969860605718, 0.6784773152999695744, 11.73519575009920857 ) ) ;
#5847=EDGE_LOOP ( 'NONE', ( #6076, #8953, #8968, #4579 ) ) ;
#5848=AXIS2_PLACEMENT_3D ( 'NONE', #2337, #10267, #12410 ) ;
#5849=FACE_OUTER_BOUND ( 'NONE', #12506, .T. ) ;
#5859=VECTOR ( 'NONE', #12727, 1000.000000000000114 ) ;
#5860=EDGE_LOOP ( 'NONE', ( #3751, #2734, #7671, #22 ) ) ;
#5865=DIRECTION ( 'NONE',  ( 0.000000000000000000, 0.000000000000000000, -1.000000000000000000 ) ) ;
#5869=CIRCLE ( 'NONE', #7002, 6.500000000000005329 ) ;
#5870=CARTESIAN_POINT ( 'NONE',  ( -239.5361044668159991, -1.848645179572815156, 11.60366368868215758 ) ) ;
#5875=CARTESIAN_POINT ( 'NONE',  ( -249.7982158291746941, 11.73176039496360445, -0.7224695577198212426 ) ) ;
#5881=CARTESIAN_POINT ( 'NONE',  ( 0.000000000000000000, -2.957522019940860139E-14, 0.000000000000000000 ) ) ;
#5883=ADVANCED_FACE ( 'NONE', ( #2912 ), #9678, .F. ) ;
#5884=ADVANCED_FACE ( 'NONE', ( #8937 ), #1174, .F. ) ;
#5890=EDGE_CURVE ( 'NONE', #10191, #552, #11397, .T. ) ;
#5894=ORIENTED_EDGE ( 'NONE', *, *, #5890, .F. ) ;
#5898=CARTESIAN_POINT ( 'NONE',  ( 71.82423009839129691, 30.00000000000000000, 203.8354503650404865 ) ) ;
#5899=CARTESIAN_POINT ( 'NONE',  ( 0.000000000000000000, -20.00000000000000000, -231.0000000000000000 ) ) ;
#5900=AXIS2_PLACEMENT_3D ( 'NONE', #1355, #6356, #5353 ) ;
#5901=ORIENTED_EDGE ( 'NONE', *, *, #11244, .F. ) ;
#5903=ADVANCED_FACE ( 'NONE', ( #3988 ), #11062, .T. ) ;
#5905=ADVANCED_FACE ( 'NONE', ( #8001 ), #9903, .T. ) ;
#5906=CARTESIAN_POINT ( 'NONE',  ( -247.1684828253810906, 9.630976095903571732, -6.736800400388656129 ) ) ;
#5908=AXIS2_PLACEMENT_3D ( 'NONE', #1642, #7906, #11848 ) ;
#5909=DIRECTION ( 'NONE',  ( 0.000000000000000000, 0.000000000000000000, 1.000000000000000000 ) ) ;
#5912=DIRECTION ( 'NONE',  ( 0.000000000000000000, -0.7071067811865480168, -0.7071067811865470176 ) ) ;
#5914=FACE_BOUND ( 'NONE', #8022, .T. ) ;
#5917=AXIS2_PLACEMENT_3D ( 'NONE', #6575, #1438, #5500 ) ;
#5921=CARTESIAN_POINT ( 'NONE',  ( -238.7194017472469341, -0.2080061402095525758, -11.74814821798330478 ) ) ;
#5925=CARTESIAN_POINT ( 'NONE',  ( -249.2624683436029898, -10.49496574118427716, -5.283769350921994068 ) ) ;
#5930=LINE ( 'NONE', #4852, #1469 ) ;
#5937=AXIS2_PLACEMENT_3D ( 'NONE', #2476, #10347, #2278 ) ;
#5940=AXIS2_PLACEMENT_3D ( 'NONE', #6493, #1481, #9535 ) ;
#5944=ORIENTED_EDGE ( 'NONE', *, *, #6818, .T. ) ;
#5945=AXIS2_PLACEMENT_3D ( 'NONE', #8603, #12662, #6864 ) ;
#5949=CARTESIAN_POINT ( 'NONE',  ( -197.8197553893909912, 30.00000000000000000, 64.27553482999130097 ) ) ;
#5953=CARTESIAN_POINT ( 'NONE',  ( -244.9693137076198752, -8.715706976269279593, 7.881056910973075702 ) ) ;
#5955=EDGE_CURVE ( 'NONE', #7121, #8160, #6083, .T. ) ;
#5956=CARTESIAN_POINT ( 'NONE',  ( 197.8197553893920144, 18.00000000000000000, 70.77553482998851564 ) ) ;
#5958=CIRCLE ( 'NONE', #4883, 5.500000000000005329 ) ;
#5959=MANIFOLD_SOLID_BREP ( 'NONE', #6257 ) ;
#5961=ORIENTED_EDGE ( 'NONE', *, *, #10627, .F. ) ;
#5962=ORIENTED_EDGE ( 'NONE', *, *, #9547, .T. ) ;
#5964=DIRECTION ( 'NONE',  ( 0.000000000000000000, -0.7071067811865489050, -0.7071067811865460184 ) ) ;
#5966=CARTESIAN_POINT ( 'NONE',  ( -249.0998459876556979, 10.33180199737826577, 5.596503889598144710 ) ) ;
#5973=CARTESIAN_POINT ( 'NONE',  ( 71.82423009839129691, 30.00000000000000000, -197.3354503650404865 ) ) ;
#5974=ORIENTED_EDGE ( 'NONE', *, *, #3004, .F. ) ;
#5975=CARTESIAN_POINT ( 'NONE',  ( -246.1720478471803517, 9.282004956765195658, -7.205195109033324385 ) ) ;
#5976=ORIENTED_EDGE ( 'NONE', *, *, #4801, .F. ) ;
#5980=CARTESIAN_POINT ( 'NONE',  ( 240.3826708216974737, 2.772967769358989809, -2.135567781667440102 ) ) ;
#5982=CARTESIAN_POINT ( 'NONE',  ( 0.000000000000000000, 0.000000000000000000, -249.7999999999999829 ) ) ;
#5991=EDGE_CURVE ( 'NONE', #8275, #7222, #12792, .T. ) ;
#5992=VERTEX_POINT ( 'NONE', #1128 ) ;
#5993=VERTEX_POINT ( 'NONE', #1646 ) ;
#5994=CARTESIAN_POINT ( 'NONE',  ( -248.8285144558357445, -10.12619208585344133, 5.960099103772717122 ) ) ;
#5995=ORIENTED_EDGE ( 'NONE', *, *, #5705, .T. ) ;
#5999=CARTESIAN_POINT ( 'NONE',  ( 0.000000000000000000, 0.000000000000000000, 0.000000000000000000 ) ) ;
#6002=CARTESIAN_POINT ( 'NONE',  ( -239.3015193013782209, -1.606994374921540736, -11.63956803099216586 ) ) ;
#6005=CARTESIAN_POINT ( 'NONE',  ( 122.2593324768334071, 18.00000000000000000, -161.7755348299894820 ) ) ;
#6010=ORIENTED_EDGE ( 'NONE', *, *, #11781, .T. ) ;
#6014=CARTESIAN_POINT ( 'NONE',  ( 0.000000000000000000, 9.830508068699479907, 248.1666666666505137 ) ) ;
#6015=DIRECTION ( 'NONE',  ( 0.000000000000000000, -0.7071067811865489050, -0.7071067811865460184 ) ) ;
#6016=CIRCLE ( 'NONE', #11558, 6.500000000000005329 ) ;
#6017=CARTESIAN_POINT ( 'NONE',  ( -197.8197553893924976, 29.00000000000000000, -58.77553482998720114 ) ) ;
#6018=DIRECTION ( 'NONE',  ( 0.000000000000000000, 1.000000000000000000, 0.000000000000000000 ) ) ;
#6021=CARTESIAN_POINT ( 'NONE',  ( -243.1145437064502062, -7.410518230721312882, 9.118492839119728188 ) ) ;
#6023=AXIS2_PLACEMENT_3D ( 'NONE', #8149, #12214, #11205 ) ;
#6024=FACE_OUTER_BOUND ( 'NONE', #9774, .T. ) ;
#6027=EDGE_LOOP ( 'NONE', ( #1797, #9898 ) ) ;
#6029=CARTESIAN_POINT ( 'NONE',  ( 0.000000000000000000, -20.00000000000000000, 0.000000000000000000 ) ) ;
#6032=CARTESIAN_POINT ( 'NONE',  ( -249.6727234477378090, 11.17009475772721494, 3.645778574476101763 ) ) ;
#6034=ADVANCED_FACE ( 'NONE', ( #7525 ), #5218, .F. ) ;
#6037=CARTESIAN_POINT ( 'NONE',  ( -243.1925160191523219, 7.478514345020445653, 9.062807753481795459 ) ) ;
#6038=ORIENTED_EDGE ( 'NONE', *, *, #12634, .T. ) ;
#6039=DIRECTION ( 'NONE',  ( 0.000000000000000000, 1.000000000000000000, 0.000000000000000000 ) ) ;
#6040=AXIS2_PLACEMENT_3D ( 'NONE', #12498, #10430, #506 ) ;
#6041=ORIENTED_EDGE ( 'NONE', *, *, #11291, .T. ) ;
#6042=AXIS2_PLACEMENT_3D ( 'NONE', #3408, #5550, #11629 ) ;
#6043=CARTESIAN_POINT ( 'NONE',  ( -239.2405902068692569, 1.531671734703150323, 11.64972311196225085 ) ) ;
#6044=ORIENTED_EDGE ( 'NONE', *, *, #4257, .T. ) ;
#6046=DIRECTION ( 'NONE',  ( 0.000000000000000000, 0.000000000000000000, 1.000000000000000000 ) ) ;
#6049=DIRECTION ( 'NONE',  ( 0.000000000000000000, 1.000000000000000000, 0.000000000000000000 ) ) ;
#6050=CONICAL_SURFACE ( 'NONE', #731, 5.500000000000005329, 0.7853981633974461696 ) ;
#6053=CIRCLE ( 'NONE', #9878, 6.499999999999999112 ) ;
#6056=ORIENTED_EDGE ( 'NONE', *, *, #371, .F. ) ;
#6057=CARTESIAN_POINT ( 'NONE',  ( -239.1331745461246783, -1.386667398511050253, -11.66814598037958461 ) ) ;
#6058=ORIENTED_EDGE ( 'NONE', *, *, #1829, .F. ) ;
#6067=CARTESIAN_POINT ( 'NONE',  ( -247.4721532363031429, -9.698102445084007428, -6.633777139480653950 ) ) ;
#6074=ADVANCED_FACE ( 'NONE', ( #4510 ), #3512, .F. ) ;
#6075=DIRECTION ( 'NONE',  ( 0.000000000000000000, 1.000000000000000000, 0.000000000000000000 ) ) ;
#6076=ORIENTED_EDGE ( 'NONE', *, *, #6958, .T. ) ;
#6080=CARTESIAN_POINT ( 'NONE',  ( -122.2593324768321992, 29.00000000000000000, 168.2755348299905052 ) ) ;
#6082=DIRECTION ( 'NONE',  ( 0.000000000000000000, 0.000000000000000000, -1.000000000000000000 ) ) ;
#6083=B_SPLINE_CURVE_WITH_KNOTS ( 'NONE', 3,
 ( #12130, #4255, #6200, #3249, #12522, #4187, #3182, #7459, #11532, #8267, #2387, #5185, #5324, #12330, #10254, #10457, #7263, #8335, #11329, #10320, #2191, #7391, #6465, #4318, #9394, #6332, #12393, #5257, #6270 ),
 .UNSPECIFIED., .F., .F.,
 ( 4, 2, 2, 1, 1, 2, 2, 2, 1, 1, 2, 2, 2, 1, 2, 2, 4 ),
 ( 0.000000000000000000, 0.06264877319547468293, 0.09397315979321198276, 0.1096353530920806812, 0.1174664497415151138, 0.1213819980662255715, 0.1252975463909360154, 0.1879463195863035341, 0.2192707061839873350, 0.2349328994828293049, 0.2427639961322546058, 0.2505950927816799068, 0.3132438659770597766, 0.3445682525747496561, 0.3602304458735945958, 0.3758926391724394800, 0.5011901855632154845 ),
 .UNSPECIFIED. ) ;
#6084=FACE_OUTER_BOUND ( 'NONE', #3132, .T. ) ;
#6085=DIRECTION ( 'NONE',  ( 0.000000000000000000, 1.000000000000000000, 0.000000000000000000 ) ) ;
#6087=CARTESIAN_POINT ( 'NONE',  ( -244.2185274273184064, -8.258776625530128257, 8.357937760093166801 ) ) ;
#6089=ORIENTED_EDGE ( 'NONE', *, *, #1874, .T. ) ;
#6092=CARTESIAN_POINT ( 'NONE',  ( 229.9901544136290568, -2.781634392067636519, 2.136699187716680992 ) ) ;
#6096=DIRECTION ( 'NONE',  ( 0.000000000000000000, 1.000000000000000000, 0.000000000000000000 ) ) ;
#6100=CARTESIAN_POINT ( 'NONE',  ( -245.4266968885101505, 8.952647108375709095, 7.610034337147152605 ) ) ;
#6103=ORIENTED_EDGE ( 'NONE', *, *, #416, .F. ) ;
#6104=DIRECTION ( 'NONE',  ( 0.000000000000000000, -1.000000000000000000, 0.000000000000000000 ) ) ;
#6114=CARTESIAN_POINT ( 'NONE',  ( 239.7985776503645354, -1.848645179573700004, 2.971954070984049956 ) ) ;
#6115=EDGE_LOOP ( 'NONE', ( #3629, #9364, #12642, #221 ) ) ;
#6116=CARTESIAN_POINT ( 'NONE',  ( -249.4432382447466807, 10.72467464915493984, -4.802290506997906938 ) ) ;
#6117=FACE_OUTER_BOUND ( 'NONE', #10656, .T. ) ;
#6120=CARTESIAN_POINT ( 'NONE',  ( -249.6793054724743399, -11.18791971366320404, 3.590677820429848399 ) ) ;
#6121=VERTEX_POINT ( 'NONE', #2450 ) ;
#6124=CARTESIAN_POINT ( 'NONE',  ( 197.8197553893915028, 18.00000000000000000, -64.27553482998990830 ) ) ;
#6125=CARTESIAN_POINT ( 'NONE',  ( -244.7823818367005515, -8.610125648031120349, -7.996289175493550339 ) ) ;
#6130=DIRECTION ( 'NONE',  ( 0.000000000000000000, 0.000000000000000000, 1.000000000000000000 ) ) ;
#6132=CARTESIAN_POINT ( 'NONE',  ( -229.8301233945847457, -7.761986000019901688, 8.855266263419107275 ) ) ;
#6138=ORIENTED_EDGE ( 'NONE', *, *, #5661, .F. ) ;
#6142=CARTESIAN_POINT ( 'NONE',  ( 197.8197553893920144, 30.00000000000000000, 70.77553482998851564 ) ) ;
#6150=CARTESIAN_POINT ( 'NONE',  ( -244.1927368917095009, -8.241533435392154772, 8.374943118319487567 ) ) ;
#6154=DIRECTION ( 'NONE',  ( 1.000000000000000000, 0.000000000000000000, 0.000000000000000000 ) ) ;
#6157=AXIS2_PLACEMENT_3D ( 'NONE', #596, #5727, #5252 ) ;
#6158=LINE ( 'NONE', #1674, #11250 ) ;
#6159=DIRECTION ( 'NONE',  ( 0.000000000000000000, 0.000000000000000000, 1.000000000000000000 ) ) ;
#6161=AXIS2_PLACEMENT_3D ( 'NONE', #2003, #6075, #2328 ) ;
#6166=CARTESIAN_POINT ( 'NONE',  ( -241.5784935620077363, 5.720435375430025893, 10.26436795268994651 ) ) ;
#6169=VERTEX_POINT ( 'NONE', #7713 ) ;
#6171=EDGE_CURVE ( 'NONE', #12220, #12270, #340, .T. ) ;
#6173=CARTESIAN_POINT ( 'NONE',  ( 0.000000000000000000, 22.00000000000000000, -245.7999999999999829 ) ) ;
#6174=ORIENTED_EDGE ( 'NONE', *, *, #1805, .T. ) ;
#6176=VECTOR ( 'NONE', #208, 1000.000000000000000 ) ;
#6177=LINE ( 'NONE', #10229, #9189 ) ;
#6178=CARTESIAN_POINT ( 'NONE',  ( 239.0232640335164263, 0.4900023590031949983, 3.465599286974978543 ) ) ;
#6179=DIRECTION ( 'NONE',  ( 0.000000000000000000, 1.000000000000000000, 0.000000000000000000 ) ) ;
#6180=AXIS2_PLACEMENT_3D ( 'NONE', #9570, #6652, #7516 ) ;
#6182=CARTESIAN_POINT ( 'NONE',  ( 71.82423009839129691, 28.60000000000000142, 197.3354503650404865 ) ) ;
#6185=EDGE_LOOP ( 'NONE', ( #7023, #10897, #7752, #6824 ) ) ;
#6187=ORIENTED_EDGE ( 'NONE', *, *, #9123, .T. ) ;
#6191=FACE_OUTER_BOUND ( 'NONE', #5088, .T. ) ;
#6192=ORIENTED_EDGE ( 'NONE', *, *, #4259, .F. ) ;
#6196=VECTOR ( 'NONE', #2048, 1000.000000000000114 ) ;
#6197=CARTESIAN_POINT ( 'NONE',  ( -243.1833766790699087, -7.470616520369461888, -9.069320236344923458 ) ) ;
#6200=CARTESIAN_POINT ( 'NONE',  ( 239.6582758811249789, -1.713542963182288936, 3.052483991793907947 ) ) ;
#6203=CARTESIAN_POINT ( 'NONE',  ( 197.8197553893920144, 30.00000000000000000, 64.27553482998850143 ) ) ;
#6204=ORIENTED_EDGE ( 'NONE', *, *, #11419, .T. ) ;
#6205=EDGE_LOOP ( 'NONE', ( #3684, #2611, #11370, #661 ) ) ;
#6210=CARTESIAN_POINT ( 'NONE',  ( 239.2334266249513917, -1.105838440500075848, -3.321566349845947119 ) ) ;
#6213=EDGE_CURVE ( 'NONE', #157, #3155, #1392, .T. ) ;
#6215=CARTESIAN_POINT ( 'NONE',  ( 71.82423009839129691, 30.00000000000000000, -197.3354503650404865 ) ) ;
#6217=CARTESIAN_POINT ( 'NONE',  ( -241.3472527821318181, -5.384021912605467364, 10.44389002220115614 ) ) ;
#6223=CARTESIAN_POINT ( 'NONE',  ( 229.9760382323824501, -1.128309064994147626, 3.321078061868915743 ) ) ;
#6224=ORIENTED_EDGE ( 'NONE', *, *, #4183, .T. ) ;
#6225=ORIENTED_EDGE ( 'NONE', *, *, #464, .T. ) ;
#6229=DIRECTION ( 'NONE',  ( 0.000000000000000000, 0.000000000000000000, -1.000000000000000000 ) ) ;
#6236=CARTESIAN_POINT ( 'NONE',  ( -241.3731105455106842, 5.422910281599071958, 10.42375653614991826 ) ) ;
#6245=VECTOR ( 'NONE', #11710, 1000.000000000000114 ) ;
#6247=CARTESIAN_POINT ( 'NONE',  ( 239.4370728336666048, 1.442813601903317977, 3.188799201111035320 ) ) ;
#6248=CARTESIAN_POINT ( 'NONE',  ( 0.000000000000000000, -2.957522019940860139E-14, 0.000000000000000000 ) ) ;
#6249=EDGE_CURVE ( 'NONE', #1505, #1172, #4109, .T. ) ;
#6251=CARTESIAN_POINT ( 'NONE',  ( -122.2593324768359935, 29.00000000000000000, -168.2755348299880040 ) ) ;
#6253=AXIS2_PLACEMENT_3D ( 'NONE', #7565, #8444, #11639 ) ;
#6254=AXIS2_PLACEMENT_3D ( 'NONE', #9180, #7249, #9251 ) ;
#6257=CLOSED_SHELL ( 'NONE', ( #5659, #4718, #9321, #2862, #12107, #8761, #818, #7824, #5903, #9463, #777, #12332, #8669, #9688, #5078, #5905, #9949, #10865, #13, #1844, #1343, #12492, #8767, #9573, #10643, #6632, #7339, #176, #9232, #3030, #12962, #10264, #10528, #11706, #10053, #9415, #4993, #5408, #4720, #11081, #8448, #10887, #297, #8158, #8292, #923, #8364, #4108, #5883, #5884, #2644, #3847, #578, #8012, #3262, #9565, #1103, #4116, #939, #460, #12817, #10216, #4521, #7588, #9295, #12439, #11428, #8512, #9765, #1915, #8843, #10435, #5301, #4820, #2150, #6034, #7455, #5080, #11599, #2007, #754, #12944, #12494, #11946, #6364, #12365, #13008, #9296, #10029, #6391, #3055, #10786, #7757, #4745, #12198, #8260, #1964, #9093, #1588, #10594, #8721, #10788, #10837, #2062, #7853, #3219, #682, #12819, #9076, #4639, #4748, #10561, #10932, #6074, #8811, #6571, #8028, #7823, #6331, #2443, #8486, #137, #3702, #7809, #9335, #2389, #1629, #12591, #10462, #11849, #3294, #8076, #602, #7274, #3672 ) ) ;
#6258=CARTESIAN_POINT ( 'NONE',  ( -197.8197553893909912, 30.00000000000000000, 69.77553482999131518 ) ) ;
#6260=CIRCLE ( 'NONE', #9645, 239.8169934640465044 ) ;
#6263=CARTESIAN_POINT ( 'NONE',  ( -248.5980333526342179, -9.980365686173904294, 6.207212898096353015 ) ) ;
#6264=ORIENTED_EDGE ( 'NONE', *, *, #10718, .T. ) ;
#6265=VECTOR ( 'NONE', #11366, 1000.000000000000000 ) ;
#6269=CARTESIAN_POINT ( 'NONE',  ( -245.2557111518780459, -8.868800241211268087, -7.708496933118081706 ) ) ;
#6270=CARTESIAN_POINT ( 'NONE',  ( 238.9743710777160857, 8.519355453646930632E-11, 3.499999942258626984 ) ) ;
#6272=CARTESIAN_POINT ( 'NONE',  ( 240.5378997430644858, 3.246179723024485764, 1.312253685488862009 ) ) ;
#6276=EDGE_LOOP ( 'NONE', ( #1173, #749, #143, #4118 ) ) ;
#6278=CARTESIAN_POINT ( 'NONE',  ( 0.000000000000000000, -20.00000000000000000, 0.000000000000000000 ) ) ;
#6279=CARTESIAN_POINT ( 'NONE',  ( -248.7692280201405310, 10.08940167824826339, 6.022204372445879805 ) ) ;
#6280=VECTOR ( 'NONE', #10894, 1000.000000000000000 ) ;
#6283=CARTESIAN_POINT ( 'NONE',  ( 71.82423009839129691, 19.40000000000000213, 202.4354503650404808 ) ) ;
#6285=FACE_OUTER_BOUND ( 'NONE', #7119, .T. ) ;
#6287=DIRECTION ( 'NONE',  ( 0.000000000000000000, 1.000000000000000000, 0.000000000000000000 ) ) ;
#6288=ORIENTED_EDGE ( 'NONE', *, *, #12515, .F. ) ;
#6289=DIRECTION ( 'NONE',  ( 0.000000000000000000, 1.000000000000000000, 0.000000000000000000 ) ) ;
#6292=DIRECTION ( 'NONE',  ( 0.000000000000000000, 0.000000000000000000, 1.000000000000000000 ) ) ;
#6293=VERTEX_POINT ( 'NONE', #12248 ) ;
#6300=DIRECTION ( 'NONE',  ( 0.000000000000000000, 0.000000000000000000, 1.000000000000000000 ) ) ;
#6303=CARTESIAN_POINT ( 'NONE',  ( -242.5648157350879899, 6.889953638923882906, 9.518299937401890176 ) ) ;
#6307=CARTESIAN_POINT ( 'NONE',  ( 0.000000000000000000, -20.00000000000000000, 0.000000000000000000 ) ) ;
#6312=FACE_OUTER_BOUND ( 'NONE', #3902, .T. ) ;
#6315=CARTESIAN_POINT ( 'NONE',  ( 239.4975972760159948, 1.524294660007503355, -3.150668453783941114 ) ) ;
#6316=CARTESIAN_POINT ( 'NONE',  ( -238.7193995381545335, 0.2079802334036294775, -11.74814885867293413 ) ) ;
#6319=EDGE_CURVE ( 'NONE', #1045, #7994, #5445, .T. ) ;
#6322=EDGE_LOOP ( 'NONE', ( #2551, #6417 ) ) ;
#6323=CARTESIAN_POINT ( 'NONE',  ( -122.2593324768321992, 29.00000000000000000, 173.7755348299905052 ) ) ;
#6325=CARTESIAN_POINT ( 'NONE',  ( -197.8197553893909912, 19.00000000000000000, 64.27553482999130097 ) ) ;
#6326=ORIENTED_EDGE ( 'NONE', *, *, #3506, .F. ) ;
#6330=CARTESIAN_POINT ( 'NONE',  ( -242.0448478369141299, -6.321212806544949991, -9.907269457473429242 ) ) ;
#6331=ADVANCED_FACE ( 'NONE', ( #11759 ), #972, .F. ) ;
#6332=CARTESIAN_POINT ( 'NONE',  ( 239.0381261355857703, -0.5585874493611364677, 3.455211367194953809 ) ) ;
#6334=CARTESIAN_POINT ( 'NONE',  ( 240.4535390813594233, 3.009067775009412582, -1.828999331050441102 ) ) ;
#6340=CYLINDRICAL_SURFACE ( 'NONE', #311, 249.7999999999999829 ) ;
#6341=LINE ( 'NONE', #10393, #9973 ) ;
#6342=CARTESIAN_POINT ( 'NONE',  ( 239.6467530156110683, -1.711397834369177140, -3.057326064312821945 ) ) ;
#6343=DIRECTION ( 'NONE',  ( 0.000000000000000000, -1.000000000000000000, 0.000000000000000000 ) ) ;
#6350=EDGE_LOOP ( 'NONE', ( #8760, #9919, #11538, #12464 ) ) ;
#6351=DIRECTION ( 'NONE',  ( 0.000000000000000000, 0.000000000000000000, -1.000000000000000000 ) ) ;
#6352=CARTESIAN_POINT ( 'NONE',  ( 229.9785025033683326, -1.551323116862773244, -3.145807476139447889 ) ) ;
#6354=VERTEX_POINT ( 'NONE', #10749 ) ;
#6356=DIRECTION ( 'NONE',  ( 0.000000000000000000, 1.000000000000000000, 0.000000000000000000 ) ) ;
#6363=CARTESIAN_POINT ( 'NONE',  ( 0.000000000000000000, 30.00000000000000000, -201.4999999999999716 ) ) ;
#6364=ADVANCED_FACE ( 'NONE', ( #7879 ), #8850, .F. ) ;
#6373=ORIENTED_EDGE ( 'NONE', *, *, #10460, .F. ) ;
#6377=DIRECTION ( 'NONE',  ( 0.000000000000000000, 1.000000000000000000, 0.000000000000000000 ) ) ;
#6379=CARTESIAN_POINT ( 'NONE',  ( 239.2304539311643623, 1.097329040102013931, -3.323615143739755862 ) ) ;
#6383=ORIENTED_EDGE ( 'NONE', *, *, #1030, .F. ) ;
#6384=CARTESIAN_POINT ( 'NONE',  ( -122.2593324768359935, 19.00000000000000000, -162.7755348299880040 ) ) ;
#6385=ORIENTED_EDGE ( 'NONE', *, *, #8882, .F. ) ;
#6386=LINE ( 'NONE', #12313, #7835 ) ;
#6390=ORIENTED_EDGE ( 'NONE', *, *, #7901, .T. ) ;
#6391=ADVANCED_FACE ( 'NONE', ( #4606 ), #2035, .F. ) ;
#6392=AXIS2_PLACEMENT_3D ( 'NONE', #2506, #12516, #11652 ) ;
#6393=DIRECTION ( 'NONE',  ( 0.000000000000000000, 1.000000000000000000, 0.000000000000000000 ) ) ;
#6398=AXIS2_PLACEMENT_3D ( 'NONE', #2527, #4520, #4455 ) ;
#6408=DIRECTION ( 'NONE',  ( 0.000000000000000000, 0.000000000000000000, -1.000000000000000000 ) ) ;
#6412=CARTESIAN_POINT ( 'NONE',  ( 0.000000000000000000, 21.50000000000000000, 0.000000000000000000 ) ) ;
#6416=CARTESIAN_POINT ( 'NONE',  ( -246.6344430662078366, -9.451372532214236344, 6.980988236095548416 ) ) ;
#6417=ORIENTED_EDGE ( 'NONE', *, *, #4600, .F. ) ;
#6418=CYLINDRICAL_SURFACE ( 'NONE', #5329, 5.500000000000005329 ) ;
#6420=DIRECTION ( 'NONE',  ( 0.000000000000000000, 0.000000000000000000, 1.000000000000000000 ) ) ;
#6421=VERTEX_POINT ( 'NONE', #4808 ) ;
#6424=FACE_OUTER_BOUND ( 'NONE', #5417, .T. ) ;
#6432=LINE ( 'NONE', #1361, #7316 ) ;
#6439=EDGE_LOOP ( 'NONE', ( #10211, #3818, #2704, #9302, #5024, #9762 ) ) ;
#6441=EDGE_CURVE ( 'NONE', #1401, #368, #3734, .T. ) ;
#6445=CARTESIAN_POINT ( 'NONE',  ( 7.960204194457795477E-16, 30.00000000000000000, -214.5000000000000000 ) ) ;
#6448=VERTEX_POINT ( 'NONE', #3745 ) ;
#6449=DIRECTION ( 'NONE',  ( 0.000000000000000000, 1.000000000000000000, 0.000000000000000000 ) ) ;
#6451=ORIENTED_EDGE ( 'NONE', *, *, #2540, .F. ) ;
#6454=CARTESIAN_POINT ( 'NONE',  ( -210.0000000000000000, 30.00000000000000000, -6.500000000000000000 ) ) ;
#6457=EDGE_CURVE ( 'NONE', #10014, #11841, #5459, .T. ) ;
#6460=DIRECTION ( 'NONE',  ( 0.000000000000000000, 1.000000000000000000, 0.000000000000000000 ) ) ;
#6461=DIRECTION ( 'NONE',  ( 0.000000000000000000, 1.000000000000000000, 0.000000000000000000 ) ) ;
#6462=AXIS2_PLACEMENT_3D ( 'NONE', #880, #9939, #6886 ) ;
#6465=CARTESIAN_POINT ( 'NONE',  ( 239.0693672988234653, -0.6815372136754875854, 3.433431997329027041 ) ) ;
#6471=AXIS2_PLACEMENT_3D ( 'NONE', #7636, #3429, #11777 ) ;
#6472=DIRECTION ( 'NONE',  ( 0.000000000000000000, 0.000000000000000000, 1.000000000000000000 ) ) ;
#6473=AXIS2_PLACEMENT_3D ( 'NONE', #7750, #6695, #10748 ) ;
#6476=FACE_OUTER_BOUND ( 'NONE', #4248, .T. ) ;
#6477=DIRECTION ( 'NONE',  ( 8.659560562354926695E-17, 0.7071067811865480168, -0.7071067811865470176 ) ) ;
#6478=CARTESIAN_POINT ( 'NONE',  ( 122.2593324768346008, 19.00000000000000000, 168.2755348299889988 ) ) ;
#6487=CARTESIAN_POINT ( 'NONE',  ( 240.6075165363166093, -3.437532598149585450, -0.7648284531270139741 ) ) ;
#6489=ORIENTED_EDGE ( 'NONE', *, *, #9910, .T. ) ;
#6490=VERTEX_POINT ( 'NONE', #7017 ) ;
#6493=CARTESIAN_POINT ( 'NONE',  ( 197.8197553893915028, 30.00000000000000000, -64.27553482998990830 ) ) ;
#6495=CONICAL_SURFACE ( 'NONE', #12865, 5.100000000000000533, 0.7853981633974503884 ) ;
#6502=EDGE_CURVE ( 'NONE', #3121, #11054, #2128, .T. ) ;
#6503=EDGE_LOOP ( 'NONE', ( #7561, #6878, #3879, #7157 ) ) ;
#6508=ORIENTED_EDGE ( 'NONE', *, *, #7960, .T. ) ;
#6510=CARTESIAN_POINT ( 'NONE',  ( 0.000000000000000000, 1.848645179567965036, -239.8169934640518193 ) ) ;
#6513=CIRCLE ( 'NONE', #12468, 5.099999999999993427 ) ;
#6514=DIRECTION ( 'NONE',  ( 0.000000000000000000, 0.000000000000000000, 1.000000000000000000 ) ) ;
#6515=CARTESIAN_POINT ( 'NONE',  ( -239.3015052057552623, 1.606977719895358092, -11.63957048466796351 ) ) ;
#6520=ORIENTED_EDGE ( 'NONE', *, *, #6741, .F. ) ;
#6521=DIRECTION ( 'NONE',  ( 0.000000000000000000, 1.000000000000000000, 0.000000000000000000 ) ) ;
#6526=CARTESIAN_POINT ( 'NONE',  ( -229.7195242555831385, 3.042667911008530623, 11.35573322796902396 ) ) ;
#6537=CARTESIAN_POINT ( 'NONE',  ( 0.000000000000000000, 21.50000000000000000, -249.7999999999999829 ) ) ;
#6541=CARTESIAN_POINT ( 'NONE',  ( -197.8197553893909912, 19.00000000000000000, 58.77553482999130807 ) ) ;
#6543=DIRECTION ( 'NONE',  ( 0.000000000000000000, 0.000000000000000000, 1.000000000000000000 ) ) ;
#6549=CONICAL_SURFACE ( 'NONE', #5908, 230.0000000000000000, 0.7853981633974476129 ) ;
#6551=VERTEX_POINT ( 'NONE', #4461 ) ;
#6552=ORIENTED_EDGE ( 'NONE', *, *, #7598, .F. ) ;
#6558=CIRCLE ( 'NONE', #593, 10.00000000000000888 ) ;
#6562=DIRECTION ( 'NONE',  ( 0.000000000000000000, -0.7071067811864890640, -0.7071067811866059705 ) ) ;
#6566=ORIENTED_EDGE ( 'NONE', *, *, #12916, .T. ) ;
#6571=ADVANCED_FACE ( 'NONE', ( #1213 ), #7976, .T. ) ;
#6573=CARTESIAN_POINT ( 'NONE',  ( 239.3580835734670700, 1.327753754258439889, -3.239279126375866458 ) ) ;
#6574=CARTESIAN_POINT ( 'NONE',  ( -239.4550024016175769, 1.775410295146655493, -11.61533115162393592 ) ) ;
#6575=CARTESIAN_POINT ( 'NONE',  ( 0.000000000000000000, -20.00000000000000000, 0.000000000000000000 ) ) ;
#6576=DIRECTION ( 'NONE',  ( 0.000000000000000000, 1.000000000000000000, 0.000000000000000000 ) ) ;
#6577=AXIS2_PLACEMENT_3D ( 'NONE', #3238, #323, #7319 ) ;
#6579=EDGE_CURVE ( 'NONE', #9887, #7619, #1167, .T. ) ;
#6582=ORIENTED_EDGE ( 'NONE', *, *, #4271, .T. ) ;
#6583=CARTESIAN_POINT ( 'NONE',  ( -238.9094463865829709, -0.9709988936793297887, 11.70980984558256388 ) ) ;
#6584=VERTEX_POINT ( 'NONE', #12415 ) ;
#6587=AXIS2_PLACEMENT_3D ( 'NONE', #7259, #1057, #5115 ) ;
#6588=CARTESIAN_POINT ( 'NONE',  ( 7.347880794884120722E-16, 29.00000000000000000, -213.5000000000000000 ) ) ;
#6599=VERTEX_POINT ( 'NONE', #8417 ) ;
#6601=VERTEX_POINT ( 'NONE', #8545 ) ;
#6606=EDGE_CURVE ( 'NONE', #7625, #6775, #349, .T. ) ;
#6612=CARTESIAN_POINT ( 'NONE',  ( 229.9996470147345349, 3.477012619071095934, -0.4608790345419201406 ) ) ;
#6619=CARTESIAN_POINT ( 'NONE',  ( 3.059167704270088292E-14, 11.79660968244690089, -249.7999999999999829 ) ) ;
#6625=CYLINDRICAL_SURFACE ( 'NONE', #12628, 5.500000000000005329 ) ;
#6628=ORIENTED_EDGE ( 'NONE', *, *, #5254, .F. ) ;
#6632=ADVANCED_FACE ( 'NONE', ( #8479 ), #4204, .F. ) ;
#6635=ORIENTED_EDGE ( 'NONE', *, *, #4125, .F. ) ;
#6636=CIRCLE ( 'NONE', #5355, 6.500000000000000000 ) ;
#6637=CARTESIAN_POINT ( 'NONE',  ( 71.82423009839129691, 18.00000000000000000, -197.3354503650404865 ) ) ;
#6638=AXIS2_PLACEMENT_3D ( 'NONE', #4903, #10040, #6046 ) ;
#6639=CARTESIAN_POINT ( 'NONE',  ( 239.2334266250973940, 1.105838440818801116, 3.321566349753109382 ) ) ;
#6640=DIRECTION ( 'NONE',  ( 0.000000000000000000, -1.000000000000000000, 0.000000000000000000 ) ) ;
#6642=FACE_OUTER_BOUND ( 'NONE', #611, .T. ) ;
#6646=CARTESIAN_POINT ( 'NONE',  ( -238.9600686717498377, -1.084978034942615244, 11.70002422621010929 ) ) ;
#6651=CARTESIAN_POINT ( 'NONE',  ( -242.9139448639247121, 7.229284210467626259, -9.262738307079473543 ) ) ;
#6652=DIRECTION ( 'NONE',  ( 0.000000000000000000, 1.000000000000000000, 0.000000000000000000 ) ) ;
#6653=AXIS2_PLACEMENT_3D ( 'NONE', #5600, #7599, #8664 ) ;
#6654=EDGE_CURVE ( 'NONE', #2131, #11915, #12024, .T. ) ;
#6655=CARTESIAN_POINT ( 'NONE',  ( 0.000000000000000000, 25.00000000000000000, 0.000000000000000000 ) ) ;
#6656=CARTESIAN_POINT ( 'NONE',  ( 0.000000000000000000, 30.00000000000000000, 208.0000000000000000 ) ) ;
#6658=CIRCLE ( 'NONE', #9618, 6.500000000000005329 ) ;
#6659=CARTESIAN_POINT ( 'NONE',  ( -229.7429378870860717, 4.500510568802750910, 10.87411266180416547 ) ) ;
#6662=VECTOR ( 'NONE', #3693, 1000.000000000000114 ) ;
#6665=EDGE_CURVE ( 'NONE', #158, #7755, #3396, .T. ) ;
#6667=CARTESIAN_POINT ( 'NONE',  ( -122.2593324768321992, 19.00000000000000000, 173.7755348299905052 ) ) ;
#6670=CIRCLE ( 'NONE', #10705, 239.0000000000000000 ) ;
#6672=FACE_OUTER_BOUND ( 'NONE', #12871, .T. ) ;
#6674=CIRCLE ( 'NONE', #1553, 249.7999999999999829 ) ;
#6676=DIRECTION ( 'NONE',  ( 0.000000000000000000, 0.000000000000000000, 1.000000000000000000 ) ) ;
#6677=DIRECTION ( 'NONE',  ( 0.000000000000000000, 1.000000000000000000, 0.000000000000000000 ) ) ;
#6680=CARTESIAN_POINT ( 'NONE',  ( 229.9996562797466026, 3.477621119227378710, 0.4561944637181986617 ) ) ;
#6684=CARTESIAN_POINT ( 'NONE',  ( -249.6784491604725531, 11.18557168014761061, -3.597985675038290587 ) ) ;
#6689=DIRECTION ( 'NONE',  ( 0.000000000000000000, 0.000000000000000000, 1.000000000000000000 ) ) ;
#6695=DIRECTION ( 'NONE',  ( 0.000000000000000000, 1.000000000000000000, 0.000000000000000000 ) ) ;
#6696=CARTESIAN_POINT ( 'NONE',  ( 71.82423009839129691, 19.40000000000000213, 197.3354503650404865 ) ) ;
#6697=VERTEX_POINT ( 'NONE', #5804 ) ;
#6699=EDGE_CURVE ( 'NONE', #1401, #5843, #4656, .T. ) ;
#6703=ORIENTED_EDGE ( 'NONE', *, *, #1396, .T. ) ;
#6705=ORIENTED_EDGE ( 'NONE', *, *, #4365, .F. ) ;
#6706=LINE ( 'NONE', #1766, #8800 ) ;
#6707=CARTESIAN_POINT ( 'NONE',  ( -239.5361044668155159, 1.848645179572584896, -11.60366368868220022 ) ) ;
#6709=VECTOR ( 'NONE', #11549, 1000.000000000000000 ) ;
#6710=DIRECTION ( 'NONE',  ( 0.000000000000000000, -0.7071067811865489050, -0.7071067811865460184 ) ) ;
#6711=CARTESIAN_POINT ( 'NONE',  ( 0.000000000000000000, 0.000000000000000000, 0.000000000000000000 ) ) ;
#6712=DIRECTION ( 'NONE',  ( 0.000000000000000000, 1.000000000000000000, 0.000000000000000000 ) ) ;
#6716=ORIENTED_EDGE ( 'NONE', *, *, #11027, .F. ) ;
#6717=DIRECTION ( 'NONE',  ( 0.000000000000000000, -1.000000000000000000, 0.000000000000000000 ) ) ;
#6722=DIRECTION ( 'NONE',  ( 0.000000000000000000, -1.000000000000000000, 0.000000000000000000 ) ) ;
#6723=EDGE_CURVE ( 'NONE', #1001, #4565, #10864, .T. ) ;
#6724=CARTESIAN_POINT ( 'NONE',  ( -229.8696931595135311, 8.856154740712108620, -7.760084353341174079 ) ) ;
#6729=AXIS2_PLACEMENT_3D ( 'NONE', #13032, #9967, #12970 ) ;
#6730=ORIENTED_EDGE ( 'NONE', *, *, #7292, .T. ) ;
#6732=ORIENTED_EDGE ( 'NONE', *, *, #2783, .F. ) ;
#6734=CARTESIAN_POINT ( 'NONE',  ( -248.5901226956339372, -9.992747119255737331, -6.181484274823088931 ) ) ;
#6735=EDGE_LOOP ( 'NONE', ( #6752, #12481, #11531, #8723 ) ) ;
#6737=LINE ( 'NONE', #8793, #5297 ) ;
#6741=EDGE_CURVE ( 'NONE', #12659, #3500, #5429, .T. ) ;
#6742=DIRECTION ( 'NONE',  ( 0.000000000000000000, -1.000000000000000000, 0.000000000000000000 ) ) ;
#6745=CARTESIAN_POINT ( 'NONE',  ( -229.8695287356393351, -8.851891635873659681, -7.764920136789899452 ) ) ;
#6748=CARTESIAN_POINT ( 'NONE',  ( -248.8393377457010729, 10.13317597125110225, -5.948217566805436896 ) ) ;
#6752=ORIENTED_EDGE ( 'NONE', *, *, #9689, .F. ) ;
#6754=FACE_OUTER_BOUND ( 'NONE', #12166, .T. ) ;
#6759=FACE_OUTER_BOUND ( 'NONE', #7334, .T. ) ;
#6760=CARTESIAN_POINT ( 'NONE',  ( 239.8763759935475548, 1.918973793112176640, -2.928207549571361312 ) ) ;
#6762=DIRECTION ( 'NONE',  ( 8.659560562355648996E-17, -0.7071067811864890640, 0.7071067811866059705 ) ) ;
#6763=EDGE_LOOP ( 'NONE', ( #1814, #7022, #11728, #11048 ) ) ;
#6764=ORIENTED_EDGE ( 'NONE', *, *, #8442, .F. ) ;
#6768=DIRECTION ( 'NONE',  ( 0.000000000000000000, 1.000000000000000000, 0.000000000000000000 ) ) ;
#6769=AXIS2_PLACEMENT_3D ( 'NONE', #6994, #8863, #3785 ) ;
#6772=CARTESIAN_POINT ( 'NONE',  ( 3.039165139883823160E-14, -9.830508068699650437, -248.1666666666509968 ) ) ;
#6773=DIRECTION ( 'NONE',  ( 0.000000000000000000, 0.7071067811865450192, 0.7071067811865500152 ) ) ;
#6774=FACE_OUTER_BOUND ( 'NONE', #3147, .T. ) ;
#6775=VERTEX_POINT ( 'NONE', #802 ) ;
#6776=DIRECTION ( 'NONE',  ( 0.000000000000000000, 1.000000000000000000, 0.000000000000000000 ) ) ;
#6779=CARTESIAN_POINT ( 'NONE',  ( -243.1520458356562528, 7.443371746708626446, -9.091683909951978393 ) ) ;
#6780=ORIENTED_EDGE ( 'NONE', *, *, #2512, .F. ) ;
#6781=DIRECTION ( 'NONE',  ( 0.000000000000000000, 1.000000000000000000, 0.000000000000000000 ) ) ;
#6790=DIRECTION ( 'NONE',  ( 0.000000000000000000, 1.000000000000000000, 0.000000000000000000 ) ) ;
#6801=AXIS2_PLACEMENT_3D ( 'NONE', #10587, #1460, #5525 ) ;
#6802=CYLINDRICAL_SURFACE ( 'NONE', #8099, 230.0000000000000000 ) ;
#6805=CARTESIAN_POINT ( 'NONE',  ( 0.000000000000000000, 0.000000000000000000, 0.000000000000000000 ) ) ;
#6807=CARTESIAN_POINT ( 'NONE',  ( 229.9800038605684733, 1.757442049980142862, 3.035487404091129271 ) ) ;
#6809=CARTESIAN_POINT ( 'NONE',  ( -249.7762712554156224, 11.55521436326935003, 2.133810498956889123 ) ) ;
#6818=EDGE_CURVE ( 'NONE', #9288, #2131, #9068, .T. ) ;
#6823=CARTESIAN_POINT ( 'NONE',  ( 240.3826708216974737, 2.772967769358989809, -2.135567781667440102 ) ) ;
#6824=ORIENTED_EDGE ( 'NONE', *, *, #1901, .F. ) ;
#6826=CARTESIAN_POINT ( 'NONE',  ( 0.000000000000000000, -1.848645179579245124, 0.000000000000000000 ) ) ;
#6828=VERTEX_POINT ( 'NONE', #10185 ) ;
#6834=CARTESIAN_POINT ( 'NONE',  ( 197.8197553893915028, 30.00000000000000000, -69.77553482998990830 ) ) ;
#6835=LINE ( 'NONE', #8766, #11348 ) ;
#6839=CARTESIAN_POINT ( 'NONE',  ( -238.9989076641871861, 1.159495722235804216, 11.69268798918628249 ) ) ;
#6841=EDGE_CURVE ( 'NONE', #12029, #3737, #7342, .T. ) ;
#6844=CARTESIAN_POINT ( 'NONE',  ( -238.7109915777814138, -2.671037648644427152E-08, -11.74999999995326050 ) ) ;
#6849=FACE_BOUND ( 'NONE', #11302, .T. ) ;
#6851=DIRECTION ( 'NONE',  ( 0.000000000000000000, 0.000000000000000000, -1.000000000000000000 ) ) ;
#6861=CARTESIAN_POINT ( 'NONE',  ( -249.6759349623802962, -11.17873215480379478, -3.619182053975217972 ) ) ;
#6864=DIRECTION ( 'NONE',  ( 0.000000000000000000, 0.000000000000000000, 1.000000000000000000 ) ) ;
#6869=CARTESIAN_POINT ( 'NONE',  ( -248.0831933713610056, 9.830508068705238856, -6.436117704883929314 ) ) ;
#6871=CARTESIAN_POINT ( 'NONE',  ( 229.9849648984647956, 2.315196995243969713, 2.634778663479427241 ) ) ;
#6873=CARTESIAN_POINT ( 'NONE',  ( -249.2901971947193829, 10.52637179445783566, -5.220957665098429956 ) ) ;
#6878=ORIENTED_EDGE ( 'NONE', *, *, #5568, .F. ) ;
#6880=DIRECTION ( 'NONE',  ( 0.000000000000000000, -1.000000000000000000, 0.000000000000000000 ) ) ;
#6881=AXIS2_PLACEMENT_3D ( 'NONE', #3542, #11692, #2545 ) ;
#6884=AXIS2_PLACEMENT_3D ( 'NONE', #10443, #6449, #12449 ) ;
#6885=EDGE_CURVE ( 'NONE', #2835, #11841, #4350, .T. ) ;
#6886=DIRECTION ( 'NONE',  ( 0.000000000000000000, 0.000000000000000000, 1.000000000000000000 ) ) ;
#6890=CARTESIAN_POINT ( 'NONE',  ( 239.7985776503625175, 1.848645179571945185, -2.971954070985139751 ) ) ;
#6893=DIRECTION ( 'NONE',  ( 0.000000000000000000, 1.000000000000000000, 0.000000000000000000 ) ) ;
#6897=ORIENTED_EDGE ( 'NONE', *, *, #9987, .T. ) ;
#6898=CIRCLE ( 'NONE', #1575, 2.000000000000001776 ) ;
#6899=DIRECTION ( 'NONE',  ( 0.000000000000000000, 1.000000000000000000, 0.000000000000000000 ) ) ;
#6906=CARTESIAN_POINT ( 'NONE',  ( 71.82423009839129691, 19.40000000000000213, -202.4354503650404808 ) ) ;
#6908=AXIS2_PLACEMENT_3D ( 'NONE', #9624, #4369, #3295 ) ;
#6909=VERTEX_POINT ( 'NONE', #12333 ) ;
#6910=CYLINDRICAL_SURFACE ( 'NONE', #7323, 5.099999999999993427 ) ;
#6911=EDGE_LOOP ( 'NONE', ( #2363, #11749, #3979, #1320, #7411 ) ) ;
#6912=CARTESIAN_POINT ( 'NONE',  ( -246.2764285610849129, 9.322503224274816702, -7.152604636902116120 ) ) ;
#6914=AXIS2_PLACEMENT_3D ( 'NONE', #9390, #6460, #4314 ) ;
#6915=CIRCLE ( 'NONE', #8831, 5.500000000000005329 ) ;
#6916=CARTESIAN_POINT ( 'NONE',  ( 0.000000000000000000, 18.00000000000000000, 208.0000000000000000 ) ) ;
#6917=DIRECTION ( 'NONE',  ( 0.000000000000000000, 1.000000000000000000, 0.000000000000000000 ) ) ;
#6920=FACE_BOUND ( 'NONE', #108, .T. ) ;
#6923=UNCERTAINTY_MEASURE_WITH_UNIT (LENGTH_MEASURE( 1.000000000000000082E-05 ), #2321, 'distance_accuracy_value', 'NONE');
#6927=EDGE_LOOP ( 'NONE', ( #12379, #4149, #3217, #9021 ) ) ;
#6928=CARTESIAN_POINT ( 'NONE',  ( -249.7834965323052074, -11.60135170610416822, -1.863160430645350418 ) ) ;
#6929=ORIENTED_EDGE ( 'NONE', *, *, #3382, .T. ) ;
#6932=CARTESIAN_POINT ( 'NONE',  ( 71.82423009839129691, 30.00000000000000000, -190.8354503650404865 ) ) ;
#6936=EDGE_CURVE ( 'NONE', #808, #3020, #3717, .T. ) ;
#6939=CARTESIAN_POINT ( 'NONE',  ( 0.000000000000000000, 19.00000000000000000, 0.000000000000000000 ) ) ;
#6944=LINE ( 'NONE', #10802, #8778 ) ;
#6946=EDGE_LOOP ( 'NONE', ( #9087, #629, #11019, #5901 ) ) ;
#6952=CARTESIAN_POINT ( 'NONE',  ( -245.2595250088976115, -8.869312996839244789, 7.707186824084115706 ) ) ;
#6954=CARTESIAN_POINT ( 'NONE',  ( 122.2593324768334071, 29.00000000000000000, -162.7755348299894820 ) ) ;
#6956=ORIENTED_EDGE ( 'NONE', *, *, #5890, .T. ) ;
#6958=EDGE_CURVE ( 'NONE', #7179, #1648, #325, .T. ) ;
#6959=EDGE_CURVE ( 'NONE', #13033, #4811, #4990, .T. ) ;
#6960=FACE_OUTER_BOUND ( 'NONE', #184, .T. ) ;
#6963=CARTESIAN_POINT ( 'NONE',  ( 0.000000000000000000, 0.000000000000000000, 0.000000000000000000 ) ) ;
#6969=EDGE_LOOP ( 'NONE', ( #9617, #3473, #3536, #6508 ) ) ;
#6970=CARTESIAN_POINT ( 'NONE',  ( -245.1951802367414075, 8.836085396024165206, -7.745290894946786686 ) ) ;
#6971=ORIENTED_EDGE ( 'NONE', *, *, #119, .T. ) ;
#6974=DIRECTION ( 'NONE',  ( 0.000000000000000000, 0.000000000000000000, 1.000000000000000000 ) ) ;
#6975=CARTESIAN_POINT ( 'NONE',  ( 0.000000000000000000, 18.00000000000000000, -230.0000000000000000 ) ) ;
#6976=CARTESIAN_POINT ( 'NONE',  ( 239.0147185140285728, 0.4456008733042243208, 3.471580854525857074 ) ) ;
#6978=EDGE_CURVE ( 'NONE', #4030, #1172, #8411, .T. ) ;
#6979=DIRECTION ( 'NONE',  ( 0.000000000000000000, 0.000000000000000000, 1.000000000000000000 ) ) ;
#6982=CIRCLE ( 'NONE', #5917, 248.7999999999999829 ) ;
#6985=CARTESIAN_POINT ( 'NONE',  ( -238.7146408298738720, -0.1451103193397513536, -11.74918806529056603 ) ) ;
#6988=CARTESIAN_POINT ( 'NONE',  ( -249.2689385757789466, -10.50219330951161467, -5.269387968823961543 ) ) ;
#6994=CARTESIAN_POINT ( 'NONE',  ( 0.000000000000000000, -2.772967769359314882, 0.000000000000000000 ) ) ;
#6996=CARTESIAN_POINT ( 'NONE',  ( 0.000000000000000000, 30.00000000000000000, 0.000000000000000000 ) ) ;
#6998=CONICAL_SURFACE ( 'NONE', #10397, 6.500000000000005329, 0.7853981633974476129 ) ;
#6999=CARTESIAN_POINT ( 'NONE',  ( -230.0000069428143377, -11.75013590190525115, 0.3790685594532250957 ) ) ;
#7001=CIRCLE ( 'NONE', #6587, 6.500000000000005329 ) ;
#7002=AXIS2_PLACEMENT_3D ( 'NONE', #7623, #11568, #5556 ) ;
#7006=AXIS2_PLACEMENT_3D ( 'NONE', #1729, #1530, #9856 ) ;
#7007=ORIENTED_EDGE ( 'NONE', *, *, #3335, .T. ) ;
#7008=CONICAL_SURFACE ( 'NONE', #623, 5.500000000000005329, 0.7853981633974461696 ) ;
#7009=EDGE_CURVE ( 'NONE', #5207, #13031, #10955, .T. ) ;
#7011=DIRECTION ( 'NONE',  ( 0.000000000000000000, 1.000000000000000000, 0.000000000000000000 ) ) ;
#7012=FACE_OUTER_BOUND ( 'NONE', #4711, .T. ) ;
#7015=AXIS2_PLACEMENT_3D ( 'NONE', #7111, #10431, #4233 ) ;
#7017=CARTESIAN_POINT ( 'NONE',  ( -197.8197553893909912, 18.00000000000000000, 70.77553482999131518 ) ) ;
#7018=ORIENTED_EDGE ( 'NONE', *, *, #4405, .F. ) ;
#7019=LINE ( 'NONE', #7086, #4239 ) ;
#7022=ORIENTED_EDGE ( 'NONE', *, *, #11779, .F. ) ;
#7023=ORIENTED_EDGE ( 'NONE', *, *, #8203, .F. ) ;
#7027=FACE_OUTER_BOUND ( 'NONE', #10372, .T. ) ;
#7028=CARTESIAN_POINT ( 'NONE',  ( -249.2564709990199958, 10.48830713231970790, 5.296988133095193341 ) ) ;
#7030=CIRCLE ( 'NONE', #5263, 230.0000000000000000 ) ;
#7033=CARTESIAN_POINT ( 'NONE',  ( -242.0448478360703177, 6.321212805588819705, 9.907269458070054213 ) ) ;
#7036=CARTESIAN_POINT ( 'NONE',  ( -239.2643540567006539, -1.566629693467802786, 11.64555736025064903 ) ) ;
#7039=CARTESIAN_POINT ( 'NONE',  ( -244.9693137024618750, 8.715706973424389048, -7.881056914057721130 ) ) ;
#7041=DIRECTION ( 'NONE',  ( 0.000000000000000000, 1.000000000000000000, 0.000000000000000000 ) ) ;
#7043=CARTESIAN_POINT ( 'NONE',  ( 71.82423009839129691, 28.60000000000000142, -202.4354503650404808 ) ) ;
#7048=EDGE_CURVE ( 'NONE', #58, #3502, #6915, .T. ) ;
#7051=ORIENTED_EDGE ( 'NONE', *, *, #6319, .F. ) ;
#7056=EDGE_CURVE ( 'NONE', #12848, #2492, #2296, .T. ) ;
#7063=CARTESIAN_POINT ( 'NONE',  ( -241.4114469337881133, -5.479936497601446632, -10.39393372303794294 ) ) ;
#7071=ORIENTED_EDGE ( 'NONE', *, *, #5542, .F. ) ;
#7072=VERTEX_POINT ( 'NONE', #3913 ) ;
#7073=VECTOR ( 'NONE', #544, 1000.000000000000000 ) ;
#7075=CARTESIAN_POINT ( 'NONE',  ( 0.000000000000000000, -1.848645179579245124, 239.8169934640528993 ) ) ;
#7076=CARTESIAN_POINT ( 'NONE',  ( 238.9743710625051278, -0.08886714779590801361, -3.499996468587203147 ) ) ;
#7077=VECTOR ( 'NONE', #7139, 999.9999999999998863 ) ;
#7078=CARTESIAN_POINT ( 'NONE',  ( -210.0000000000000000, 18.00000000000000000, 6.500000000000007994 ) ) ;
#7082=CARTESIAN_POINT ( 'NONE',  ( -244.2253259529525167, -8.263305842909222321, 8.353459642369911009 ) ) ;
#7086=CARTESIAN_POINT ( 'NONE',  ( 122.2593324768334071, 30.00000000000000000, -161.7755348299894820 ) ) ;
#7087=CARTESIAN_POINT ( 'NONE',  ( 229.9933911495604377, -3.037488298063726777, 1.754034819793648836 ) ) ;
#7093=FACE_OUTER_BOUND ( 'NONE', #2740, .T. ) ;
#7098=CARTESIAN_POINT ( 'NONE',  ( -244.3371393072379760, 8.336835368989806483, 8.280174500310611307 ) ) ;
#7101=VERTEX_POINT ( 'NONE', #11047 ) ;
#7102=CARTESIAN_POINT ( 'NONE',  ( -239.3739003381174939, -1.702175412253983611, 11.62699861431983273 ) ) ;
#7103=CIRCLE ( 'NONE', #8173, 6.500000000000005329 ) ;
#7105=EDGE_LOOP ( 'NONE', ( #11498, #9847 ) ) ;
#7106=VECTOR ( 'NONE', #6562, 1000.000000000000000 ) ;
#7107=DIRECTION ( 'NONE',  ( 0.000000000000000000, -1.000000000000000000, 0.000000000000000000 ) ) ;
#7111=CARTESIAN_POINT ( 'NONE',  ( 0.000000000000000000, 21.50000000000000000, 0.000000000000000000 ) ) ;
#7117=AXIS2_PLACEMENT_3D ( 'NONE', #3588, #2586, #10789 ) ;
#7119=EDGE_LOOP ( 'NONE', ( #9037, #8359, #5193, #10780 ) ) ;
#7120=CARTESIAN_POINT ( 'NONE',  ( -239.2060324344808748, -1.486384979126868844, -11.65560575368058949 ) ) ;
#7121=VERTEX_POINT ( 'NONE', #6114 ) ;
#7122=CARTESIAN_POINT ( 'NONE',  ( -249.7981860219790633, 11.73141662443953059, 0.7273454842090188999 ) ) ;
#7123=LINE ( 'NONE', #11181, #6196 ) ;
#7124=VECTOR ( 'NONE', #6773, 1000.000000000000000 ) ;
#7126=CARTESIAN_POINT ( 'NONE',  ( -249.7367190362209897, -11.37209550593751572, 2.959943712984164144 ) ) ;
#7130=EDGE_CURVE ( 'NONE', #2425, #3848, #7313, .T. ) ;
#7133=CARTESIAN_POINT ( 'NONE',  ( -246.8900737883909358, -9.535158805240152802, -6.866190024035137007 ) ) ;
#7135=AXIS2_PLACEMENT_3D ( 'NONE', #4060, #8139, #12202 ) ;
#7138=CARTESIAN_POINT ( 'NONE',  ( -229.9999859999076932, -11.74972595562163136, -0.7707053339805227665 ) ) ;
#7139=DIRECTION ( 'NONE',  ( 0.000000000000000000, -0.7071067811865771047, -0.7071067811865180408 ) ) ;
#7145=DIRECTION ( 'NONE',  ( 0.000000000000000000, 1.000000000000000000, 0.000000000000000000 ) ) ;
#7146=DIRECTION ( 'NONE',  ( 0.000000000000000000, 0.000000000000000000, 1.000000000000000000 ) ) ;
#7148=EDGE_CURVE ( 'NONE', #8308, #10559, #11240, .T. ) ;
#7151=CARTESIAN_POINT ( 'NONE',  ( -240.4180123854748672, -3.650278635874803168, 11.17777342477751645 ) ) ;
#7155=CARTESIAN_POINT ( 'NONE',  ( 3.059167704270088292E-14, -11.79660968244690089, -249.7999999999999829 ) ) ;
#7156=DIRECTION ( 'NONE',  ( 0.000000000000000000, 0.000000000000000000, -1.000000000000000000 ) ) ;
#7157=ORIENTED_EDGE ( 'NONE', *, *, #2273, .T. ) ;
#7158=ORIENTED_EDGE ( 'NONE', *, *, #7196, .T. ) ;
#7160=FACE_OUTER_BOUND ( 'NONE', #5847, .T. ) ;
#7164=CARTESIAN_POINT ( 'NONE',  ( -242.2164292014367675, 6.515245625900396576, 9.778246362781860768 ) ) ;
#7169=EDGE_LOOP ( 'NONE', ( #5487, #5123 ) ) ;
#7170=EDGE_CURVE ( 'NONE', #6828, #8275, #11358, .T. ) ;
#7173=FACE_OUTER_BOUND ( 'NONE', #4312, .T. ) ;
#7179=VERTEX_POINT ( 'NONE', #8388 ) ;
#7180=FACE_OUTER_BOUND ( 'NONE', #12136, .T. ) ;
#7181=EDGE_LOOP ( 'NONE', ( #3746, #9800, #6038, #12371 ) ) ;
#7182=DIRECTION ( 'NONE',  ( 0.000000000000000000, 1.000000000000000000, 0.000000000000000000 ) ) ;
#7190=CARTESIAN_POINT ( 'NONE',  ( -244.2426106971969375, -8.274791045078215390, -8.342083836208937342 ) ) ;
#7193=EDGE_CURVE ( 'NONE', #11448, #12886, #4528, .T. ) ;
#7194=CARTESIAN_POINT ( 'NONE',  ( 240.6084075703248857, 3.437342788132964788, -0.6677429275107119588 ) ) ;
#7196=EDGE_CURVE ( 'NONE', #7625, #1432, #12424, .T. ) ;
#7199=ORIENTED_EDGE ( 'NONE', *, *, #8442, .T. ) ;
#7200=VERTEX_POINT ( 'NONE', #6384 ) ;
#7203=DIRECTION ( 'NONE',  ( 0.000000000000000000, -1.000000000000000000, 0.000000000000000000 ) ) ;
#7204=AXIS2_PLACEMENT_3D ( 'NONE', #11356, #6096, #10147 ) ;
#7205=FACE_OUTER_BOUND ( 'NONE', #3285, .T. ) ;
#7209=AXIS2_PLACEMENT_3D ( 'NONE', #2861, #7942, #2067 ) ;
#7213=AXIS2_PLACEMENT_3D ( 'NONE', #9739, #627, #4677 ) ;
#7215=CARTESIAN_POINT ( 'NONE',  ( -240.8355308714235719, -4.526241346080312589, 10.84528472031096591 ) ) ;
#7220=CARTESIAN_POINT ( 'NONE',  ( 240.4969650423268774, -3.129188642545182475, -1.571450734204370203 ) ) ;
#7222=VERTEX_POINT ( 'NONE', #3361 ) ;
#7223=ORIENTED_EDGE ( 'NONE', *, *, #2957, .T. ) ;
#7224=EDGE_CURVE ( 'NONE', #12416, #6697, #928, .T. ) ;
#7225=CIRCLE ( 'NONE', #5074, 6.500000000000005329 ) ;
#7227=DIRECTION ( 'NONE',  ( 0.000000000000000000, 0.000000000000000000, 1.000000000000000000 ) ) ;
#7233=CARTESIAN_POINT ( 'NONE',  ( -242.9798744223148788, 7.293926268967702242, 9.214525213515678104 ) ) ;
#7236=ORIENTED_EDGE ( 'NONE', *, *, #12101, .F. ) ;
#7240=ORIENTED_EDGE ( 'NONE', *, *, #4349, .F. ) ;
#7248=EDGE_LOOP ( 'NONE', ( #8551, #215, #11986, #7445 ) ) ;
#7249=DIRECTION ( 'NONE',  ( 0.000000000000000000, 1.000000000000000000, 0.000000000000000000 ) ) ;
#7250=EDGE_CURVE ( 'NONE', #2818, #12433, #8255, .T. ) ;
#7255=CARTESIAN_POINT ( 'NONE',  ( -249.7634162168646981, -11.48172779929090659, 2.515098141978860280 ) ) ;
#7259=CARTESIAN_POINT ( 'NONE',  ( 122.2593324768334071, 18.00000000000000000, -168.2755348299895104 ) ) ;
#7261=CARTESIAN_POINT ( 'NONE',  ( -241.5784935629816914, -5.720435376789357207, -10.26436795190544515 ) ) ;
#7262=ORIENTED_EDGE ( 'NONE', *, *, #519, .T. ) ;
#7263=CARTESIAN_POINT ( 'NONE',  ( 239.2173603368114243, -1.070082897910355157, 3.332413334912896818 ) ) ;
#7268=CARTESIAN_POINT ( 'NONE',  ( -197.8197553893909912, 30.00000000000000000, 64.27553482999130097 ) ) ;
#7271=CARTESIAN_POINT ( 'NONE',  ( -245.3956592407778601, 8.937419274608522812, -7.627912038536615924 ) ) ;
#7274=ADVANCED_FACE ( 'NONE', ( #7180 ), #12627, .T. ) ;
#7275=CARTESIAN_POINT ( 'NONE',  ( 239.4141849552695192, -1.410389958860294168, -3.203344683049365926 ) ) ;
#7282=ORIENTED_EDGE ( 'NONE', *, *, #3957, .T. ) ;
#7284=CARTESIAN_POINT ( 'NONE',  ( -122.2593324768359935, 19.00000000000000000, -162.7755348299880040 ) ) ;
#7285=DIRECTION ( 'NONE',  ( 0.000000000000000000, 1.000000000000000000, 0.000000000000000000 ) ) ;
#7286=ORIENTED_EDGE ( 'NONE', *, *, #7130, .F. ) ;
#7289=DIRECTION ( 'NONE',  ( 0.000000000000000000, 1.000000000000000000, 0.000000000000000000 ) ) ;
#7291=AXIS2_PLACEMENT_3D ( 'NONE', #1477, #4595, #1612 ) ;
#7292=EDGE_CURVE ( 'NONE', #1505, #9162, #3252, .T. ) ;
#7296=CARTESIAN_POINT ( 'NONE',  ( -245.9694114402524576, 9.199502179615894448, 7.310239096702775718 ) ) ;
#7297=EDGE_LOOP ( 'NONE', ( #7563, #2147, #7236, #3946 ) ) ;
#7298=LINE ( 'NONE', #2285, #6265 ) ;
#7299=EDGE_LOOP ( 'NONE', ( #5073, #10292, #3547, #7262 ) ) ;
#7302=ORIENTED_EDGE ( 'NONE', *, *, #1227, .T. ) ;
#7304=CIRCLE ( 'NONE', #1767, 196.0000000000000000 ) ;
#7308=CARTESIAN_POINT ( 'NONE',  ( 0.000000000000000000, 1.848645179567965036, 0.000000000000000000 ) ) ;
#7310=CARTESIAN_POINT ( 'NONE',  ( -239.2405828798147525, 1.531662351602087524, -11.64972450408488136 ) ) ;
#7311=CARTESIAN_POINT ( 'NONE',  ( 3.039165139883816849E-14, 9.830508068699479907, -248.1666666666505137 ) ) ;
#7313=CIRCLE ( 'NONE', #10282, 240.3921568627444856 ) ;
#7316=VECTOR ( 'NONE', #5427, 1000.000000000000000 ) ;
#7319=DIRECTION ( 'NONE',  ( 0.000000000000000000, 0.000000000000000000, 1.000000000000000000 ) ) ;
#7323=AXIS2_PLACEMENT_3D ( 'NONE', #5973, #901, #1903 ) ;
#7327=CARTESIAN_POINT ( 'NONE',  ( -244.6792151818266916, -8.549823282788482359, -8.060814825372974113 ) ) ;
#7334=EDGE_LOOP ( 'NONE', ( #9552, #2645, #9738, #8617 ) ) ;
#7336=DIRECTION ( 'NONE',  ( 0.000000000000000000, 0.000000000000000000, 1.000000000000000000 ) ) ;
#7338=CARTESIAN_POINT ( 'NONE',  ( -249.3654635699440121, 10.61071050092431989, 5.052935794436599792 ) ) ;
#7339=ADVANCED_FACE ( 'NONE', ( #10769 ), #2616, .F. ) ;
#7342=CIRCLE ( 'NONE', #7135, 195.0000000000000000 ) ;
#7347=CARTESIAN_POINT ( 'NONE',  ( -247.6398763846271436, -9.748465891248590864, 6.561428695831911462 ) ) ;
#7349=ORIENTED_EDGE ( 'NONE', *, *, #7529, .F. ) ;
#7350=DIRECTION ( 'NONE',  ( 0.000000000000000000, 0.000000000000000000, 1.000000000000000000 ) ) ;
#7352=CARTESIAN_POINT ( 'NONE',  ( 229.9983167069754018, -3.387876257721513351, 0.9084892790186469558 ) ) ;
#7353=ORIENTED_EDGE ( 'NONE', *, *, #11124, .T. ) ;
#7360=DIRECTION ( 'NONE',  ( 0.000000000000000000, 0.000000000000000000, 1.000000000000000000 ) ) ;
#7364=ORIENTED_EDGE ( 'NONE', *, *, #3681, .F. ) ;
#7365=CARTESIAN_POINT ( 'NONE',  ( -122.2593324768359935, 19.00000000000000000, -168.2755348299880040 ) ) ;
#7366=EDGE_CURVE ( 'NONE', #6584, #10501, #3465, .T. ) ;
#7369=DIRECTION ( 'NONE',  ( 0.000000000000000000, 0.000000000000000000, -1.000000000000000000 ) ) ;
#7370=ORIENTED_EDGE ( 'NONE', *, *, #59, .T. ) ;
#7373=FACE_BOUND ( 'NONE', #10035, .T. ) ;
#7375=CARTESIAN_POINT ( 'NONE',  ( 239.0693672987491425, 0.6815372134079659139, -3.433431997376373168 ) ) ;
#7378=ORIENTED_EDGE ( 'NONE', *, *, #9789, .F. ) ;
#7379=CARTESIAN_POINT ( 'NONE',  ( -197.8197553893924976, 30.00000000000000000, -64.27553482998719403 ) ) ;
#7382=DIRECTION ( 'NONE',  ( 0.000000000000000000, 1.000000000000000000, 0.000000000000000000 ) ) ;
#7390=CARTESIAN_POINT ( 'NONE',  ( -241.2214908400834474, -5.194817168110312799, -10.54181336083197884 ) ) ;
#7391=CARTESIAN_POINT ( 'NONE',  ( 239.0883580246742781, -0.7438334348235525750, 3.420275401449059505 ) ) ;
#7395=ORIENTED_EDGE ( 'NONE', *, *, #5705, .F. ) ;
#7396=CONICAL_SURFACE ( 'NONE', #1645, 5.500000000000005329, 0.7853981633974461696 ) ;
#7398=FACE_BOUND ( 'NONE', #37, .T. ) ;
#7401=DIRECTION ( 'NONE',  ( 0.000000000000000000, -1.000000000000000000, 0.000000000000000000 ) ) ;
#7402=DIRECTION ( 'NONE',  ( 0.000000000000000000, 0.000000000000000000, -1.000000000000000000 ) ) ;
#7408=LINE ( 'NONE', #11416, #11516 ) ;
#7411=ORIENTED_EDGE ( 'NONE', *, *, #428, .T. ) ;
#7413=CYLINDRICAL_SURFACE ( 'NONE', #2300, 5.500000000000005329 ) ;
#7415=TOROIDAL_SURFACE ( 'NONE', #7836, 241.5000000000000000, 2.500000000000000000 ) ;
#7418=DIRECTION ( 'NONE',  ( 0.000000000000000000, 0.000000000000000000, 1.000000000000000000 ) ) ;
#7423=TOROIDAL_SURFACE ( 'NONE', #1676, 250.0000000000000000, 10.00000000000000000 ) ;
#7424=DIRECTION ( 'NONE',  ( 0.000000000000000000, 1.000000000000000000, 0.000000000000000000 ) ) ;
#7425=EDGE_CURVE ( 'NONE', #4744, #1370, #3563, .T. ) ;
#7427=ORIENTED_EDGE ( 'NONE', *, *, #4918, .F. ) ;
#7428=VECTOR ( 'NONE', #3882, 1000.000000000000000 ) ;
#7429=CARTESIAN_POINT ( 'NONE',  ( -122.2593324768321992, 19.00000000000000000, 162.7755348299905052 ) ) ;
#7432=AXIS2_PLACEMENT_3D ( 'NONE', #6325, #5316, #254 ) ;
#7433=AXIS2_PLACEMENT_3D ( 'NONE', #9652, #8404, #5460 ) ;
#7437=CARTESIAN_POINT ( 'NONE',  ( 238.9743710159888224, -9.335707311080796797E-14, -3.499999942258349428 ) ) ;
#7439=CARTESIAN_POINT ( 'NONE',  ( -238.7322507464853629, 0.3342974598293207422, -11.74538363270618468 ) ) ;
#7441=DIRECTION ( 'NONE',  ( 0.000000000000000000, 0.000000000000000000, -1.000000000000000000 ) ) ;
#7445=ORIENTED_EDGE ( 'NONE', *, *, #1492, .F. ) ;
#7446=DIRECTION ( 'NONE',  ( 0.000000000000000000, 1.000000000000000000, 0.000000000000000000 ) ) ;
#7452=CARTESIAN_POINT ( 'NONE',  ( -240.1208361041844910, -2.772967769359084844, -11.41810622433049893 ) ) ;
#7455=ADVANCED_FACE ( 'NONE', ( #11840 ), #12576, .F. ) ;
#7456=CARTESIAN_POINT ( 'NONE',  ( -240.2602214610158455, -3.236828995517413876, -11.30545424822241252 ) ) ;
#7458=CONICAL_SURFACE ( 'NONE', #6398, 196.0000000000000000, 0.7853981633974758125 ) ;
#7459=CARTESIAN_POINT ( 'NONE',  ( 239.4793126110744197, -1.500292815854004980, 3.162144597934753332 ) ) ;
#7461=PRODUCT_CONTEXT ( 'NONE', #7982, 'mechanical' ) ;
#7468=CARTESIAN_POINT ( 'NONE',  ( 122.2593324768346008, 30.00000000000000000, 174.7755348299889988 ) ) ;
#7473=CARTESIAN_POINT ( 'NONE',  ( 0.000000000000000000, -11.79660968244690089, 247.7999999999999829 ) ) ;
#7474=DIRECTION ( 'NONE',  ( 0.000000000000000000, -1.000000000000000000, 0.000000000000000000 ) ) ;
#7479=AXIS2_PLACEMENT_3D ( 'NONE', #976, #8976, #3904 ) ;
#7480=CARTESIAN_POINT ( 'NONE',  ( -239.1867390642027544, -1.460152697550930689, 11.65892209769657661 ) ) ;
#7484=EDGE_LOOP ( 'NONE', ( #12168, #1556 ) ) ;
#7487=TOROIDAL_SURFACE ( 'NONE', #11958, 250.0000000000000000, 10.00000000000000000 ) ;
#7490=CARTESIAN_POINT ( 'NONE',  ( 0.000000000000000000, 0.000000000000000000, 0.000000000000000000 ) ) ;
#7495=EDGE_LOOP ( 'NONE', ( #10828, #5541, #2959, #10129 ) ) ;
#7498=CYLINDRICAL_SURFACE ( 'NONE', #7635, 5.100000000000000533 ) ;
#7502=LINE ( 'NONE', #9440, #4526 ) ;
#7505=EDGE_CURVE ( 'NONE', #6601, #10050, #8989, .T. ) ;
#7508=CARTESIAN_POINT ( 'NONE',  ( -239.1986688623609325, 1.476435535276028110, -11.65686989423240938 ) ) ;
#7510=ORIENTED_EDGE ( 'NONE', *, *, #790, .T. ) ;
#7513=ORIENTED_EDGE ( 'NONE', *, *, #1270, .T. ) ;
#7515=CARTESIAN_POINT ( 'NONE',  ( -243.9217790931375305, 8.053804838624140316, -8.555499775521546724 ) ) ;
#7516=DIRECTION ( 'NONE',  ( 0.000000000000000000, 0.000000000000000000, 1.000000000000000000 ) ) ;
#7522=FACE_OUTER_BOUND ( 'NONE', #11151, .T. ) ;
#7523=CONICAL_SURFACE ( 'NONE', #12000, 6.500000000000005329, 0.7853981633974476129 ) ;
#7525=FACE_OUTER_BOUND ( 'NONE', #105, .T. ) ;
#7529=EDGE_CURVE ( 'NONE', #9614, #5812, #2196, .T. ) ;
#7530=CARTESIAN_POINT ( 'NONE',  ( 197.8197553893920144, 29.00000000000000000, 64.27553482998850143 ) ) ;
#7536=DIRECTION ( 'NONE',  ( 0.000000000000000000, 0.000000000000000000, 1.000000000000000000 ) ) ;
#7549=CONICAL_SURFACE ( 'NONE', #8403, 6.500000000000005329, 0.7853981633974476129 ) ;
#7554=DIRECTION ( 'NONE',  ( 8.659560562354926695E-17, 0.7071067811865480168, -0.7071067811865470176 ) ) ;
#7561=ORIENTED_EDGE ( 'NONE', *, *, #1227, .F. ) ;
#7562=LINE ( 'NONE', #3487, #12110 ) ;
#7563=ORIENTED_EDGE ( 'NONE', *, *, #9863, .T. ) ;
#7565=CARTESIAN_POINT ( 'NONE',  ( 0.000000000000000000, 19.00000000000000000, 0.000000000000000000 ) ) ;
#7566=FACE_OUTER_BOUND ( 'NONE', #9135, .T. ) ;
#7568=CARTESIAN_POINT ( 'NONE',  ( 239.4068548684666951, 1.402387639960759103, -3.207804078284339777 ) ) ;
#7570=CARTESIAN_POINT ( 'NONE',  ( 0.000000000000000000, 0.000000000000000000, -250.0000000000000000 ) ) ;
#7571=FACE_OUTER_BOUND ( 'NONE', #2538, .T. ) ;
#7574=AXIS2_PLACEMENT_3D ( 'NONE', #12778, #9578, #3714 ) ;
#7575=ORIENTED_EDGE ( 'NONE', *, *, #107, .F. ) ;
#7576=CARTESIAN_POINT ( 'NONE',  ( -240.2520669369037023, 3.209691513938345064, -11.31204477735925451 ) ) ;
#7581=LINE ( 'NONE', #8776, #9250 ) ;
#7583=CARTESIAN_POINT ( 'NONE',  ( -229.8106098029694522, 7.168838942085261401, 9.341759543542826449 ) ) ;
#7588=ADVANCED_FACE ( 'NONE', ( #8103 ), #6910, .F. ) ;
#7590=CARTESIAN_POINT ( 'NONE',  ( 0.000000000000000000, 0.000000000000000000, -249.7999999999999829 ) ) ;
#7593=DIRECTION ( 'NONE',  ( 0.000000000000000000, 1.000000000000000000, 0.000000000000000000 ) ) ;
#7598=EDGE_CURVE ( 'NONE', #1614, #3781, #3017, .T. ) ;
#7599=DIRECTION ( 'NONE',  ( 0.000000000000000000, -1.000000000000000000, 0.000000000000000000 ) ) ;
#7600=AXIS2_PLACEMENT_3D ( 'NONE', #10607, #11423, #9602 ) ;
#7602=CARTESIAN_POINT ( 'NONE',  ( -229.8401422497489932, -8.039079579276160459, -8.578028158269177084 ) ) ;
#7604=DIRECTION ( 'NONE',  ( 8.659560562354926695E-17, -0.7071067811865480168, 0.7071067811865470176 ) ) ;
#7608=ORIENTED_EDGE ( 'NONE', *, *, #11421, .T. ) ;
#7618=DIRECTION ( 'NONE',  ( 0.000000000000000000, 1.000000000000000000, 0.000000000000000000 ) ) ;
#7619=VERTEX_POINT ( 'NONE', #1704 ) ;
#7623=CARTESIAN_POINT ( 'NONE',  ( -122.2593324768321992, 30.00000000000000000, 168.2755348299905052 ) ) ;
#7625=VERTEX_POINT ( 'NONE', #11900 ) ;
#7631=CYLINDRICAL_SURFACE ( 'NONE', #3495, 5.500000000000005329 ) ;
#7632=VECTOR ( 'NONE', #8323, 1000.000000000000000 ) ;
#7634=VERTEX_POINT ( 'NONE', #1774 ) ;
#7635=AXIS2_PLACEMENT_3D ( 'NONE', #5490, #9551, #2806 ) ;
#7636=CARTESIAN_POINT ( 'NONE',  ( 0.000000000000000000, 0.000000000000000000, 0.000000000000000000 ) ) ;
#7637=ORIENTED_EDGE ( 'NONE', *, *, #8326, .T. ) ;
#7638=CARTESIAN_POINT ( 'NONE',  ( -242.7734209817145370, 7.097132676516893390, -9.364576599533018353 ) ) ;
#7640=CONICAL_SURFACE ( 'NONE', #11274, 249.7999999999999829, 0.7853981633975309906 ) ;
#7643=CARTESIAN_POINT ( 'NONE',  ( 0.000000000000000000, 19.00000000000000000, 208.0000000000000000 ) ) ;
#7644=CARTESIAN_POINT ( 'NONE',  ( -240.9194688706963063, -4.677296209585168008, -10.77948277536260591 ) ) ;
#7645=CIRCLE ( 'NONE', #9770, 5.500000000000005329 ) ;
#7652=ORIENTED_EDGE ( 'NONE', *, *, #1769, .F. ) ;
#7653=FACE_OUTER_BOUND ( 'NONE', #8754, .T. ) ;
#7654=ORIENTED_EDGE ( 'NONE', *, *, #107, .T. ) ;
#7656=CARTESIAN_POINT ( 'NONE',  ( 0.000000000000000000, 29.00000000000000000, 208.0000000000000000 ) ) ;
#7657=DIRECTION ( 'NONE',  ( 0.000000000000000000, 0.000000000000000000, -1.000000000000000000 ) ) ;
#7659=DIRECTION ( 'NONE',  ( 0.000000000000000000, 1.000000000000000000, 0.000000000000000000 ) ) ;
#7660=EDGE_CURVE ( 'NONE', #8275, #6828, #5841, .T. ) ;
#7661=CARTESIAN_POINT ( 'NONE',  ( -240.1208361041834962, -2.772967769359314882, 11.41810622433041900 ) ) ;
#7665=CARTESIAN_POINT ( 'NONE',  ( -229.6996680450365318, -0.7764858098324382008, -11.75000000000000178 ) ) ;
#7667=CIRCLE ( 'NONE', #1929, 196.0000000000000000 ) ;
#7671=ORIENTED_EDGE ( 'NONE', *, *, #2892, .T. ) ;
#7672=PRODUCT_DEFINITION ( 'UNKNOWN', '', #9170, #8887 ) ;
#7679=CARTESIAN_POINT ( 'NONE',  ( 0.000000000000000000, 30.00000000000000000, 208.0000000000000000 ) ) ;
#7680=CARTESIAN_POINT ( 'NONE',  ( 240.1364042142066921, 2.243206690540103576, -2.686876444944948261 ) ) ;
#7683=PLANE ( 'NONE',  #4334 ) ;
#7690=VERTEX_POINT ( 'NONE', #2227 ) ;
#7692=CARTESIAN_POINT ( 'NONE',  ( -246.7009519923207108, 9.473788075149697008, 6.950529152119087506 ) ) ;
#7693=CARTESIAN_POINT ( 'NONE',  ( -122.2593324768321992, 19.00000000000000000, 162.7755348299905052 ) ) ;
#7698=ORIENTED_EDGE ( 'NONE', *, *, #6171, .F. ) ;
#7701=CARTESIAN_POINT ( 'NONE',  ( -240.4180123852993916, 3.650278635439865305, -11.17777342488509440 ) ) ;
#7704=EDGE_CURVE ( 'NONE', #552, #1965, #6898, .T. ) ;
#7711=DIRECTION ( 'NONE',  ( 0.000000000000000000, 0.7071067811865450192, 0.7071067811865500152 ) ) ;
#7712=AXIS2_PLACEMENT_3D ( 'NONE', #11361, #2222, #6300 ) ;
#7713=CARTESIAN_POINT ( 'NONE',  ( -197.8197553893909912, 30.00000000000000000, 57.77553482999130807 ) ) ;
#7714=CIRCLE ( 'NONE', #5586, 5.499999999999998224 ) ;
#7719=CARTESIAN_POINT ( 'NONE',  ( -249.7981860224685704, -11.73141662623283565, -0.7273454552846162491 ) ) ;
#7721=VECTOR ( 'NONE', #6085, 1000.000000000000000 ) ;
#7723=CARTESIAN_POINT ( 'NONE',  ( 71.82423009839129691, 19.40000000000000213, 192.2354503650404922 ) ) ;
#7726=CARTESIAN_POINT ( 'NONE',  ( 0.000000000000000000, 18.00000000000000000, 0.000000000000000000 ) ) ;
#7731=CARTESIAN_POINT ( 'NONE',  ( -229.8013896584316171, -6.844199613598257237, -9.558601023545847397 ) ) ;
#7732=AXIS2_PLACEMENT_3D ( 'NONE', #2439, #6776, #9693 ) ;
#7735=CARTESIAN_POINT ( 'NONE',  ( -249.7931653178112299, 11.67801679592136033, 1.333825769639327197 ) ) ;
#7739=EDGE_CURVE ( 'NONE', #12258, #7200, #2209, .T. ) ;
#7740=ORIENTED_EDGE ( 'NONE', *, *, #3019, .T. ) ;
#7743=CARTESIAN_POINT ( 'NONE',  ( 0.000000000000000000, -2.926905849962176352E-14, 0.000000000000000000 ) ) ;
#7745=AXIS2_PLACEMENT_3D ( 'NONE', #8347, #4267, #11545 ) ;
#7746=CIRCLE ( 'NONE', #8189, 5.499999999999998224 ) ;
#7748=CARTESIAN_POINT ( 'NONE',  ( 71.82423009839129691, 30.00000000000000000, 197.3354503650404865 ) ) ;
#7750=CARTESIAN_POINT ( 'NONE',  ( 197.8197553893915028, 30.00000000000000000, -64.27553482998990830 ) ) ;
#7752=ORIENTED_EDGE ( 'NONE', *, *, #8978, .T. ) ;
#7755=VERTEX_POINT ( 'NONE', #3218 ) ;
#7757=ADVANCED_FACE ( 'NONE', ( #12491 ), #4538, .F. ) ;
#7761=DIRECTION ( 'NONE',  ( 0.000000000000000000, 0.000000000000000000, 1.000000000000000000 ) ) ;
#7763=VECTOR ( 'NONE', #8065, 1000.000000000000000 ) ;
#7764=DIRECTION ( 'NONE',  ( 0.000000000000000000, 1.000000000000000000, 0.000000000000000000 ) ) ;
#7765=CARTESIAN_POINT ( 'NONE',  ( 122.2593324768334071, 30.00000000000000000, -168.2755348299895104 ) ) ;
#7767=EDGE_CURVE ( 'NONE', #2492, #1001, #7298, .T. ) ;
#7771=CARTESIAN_POINT ( 'NONE',  ( -243.1473425732729936, 7.439266815432667990, -9.095043743639278588 ) ) ;
#7772=EDGE_LOOP ( 'NONE', ( #1625, #9630, #6385, #4211 ) ) ;
#7775=LINE ( 'NONE', #10977, #3381 ) ;
#7776=DIRECTION ( 'NONE',  ( 0.000000000000000000, -1.000000000000000000, 0.000000000000000000 ) ) ;
#7781=SHAPE_DEFINITION_REPRESENTATION ( #3697, #11156 ) ;
#7790=CARTESIAN_POINT ( 'NONE',  ( 197.8197553893920144, 29.00000000000000000, 69.77553482998851564 ) ) ;
#7791=DIRECTION ( 'NONE',  ( 0.000000000000000000, 1.000000000000000000, 0.000000000000000000 ) ) ;
#7792=CARTESIAN_POINT ( 'NONE',  ( -247.5777789808319369, -9.724056904989312855, -6.595774162712118915 ) ) ;
#7794=CYLINDRICAL_SURFACE ( 'NONE', #260, 3.499999999999964917 ) ;
#7796=CARTESIAN_POINT ( 'NONE',  ( -229.9961401285962381, -11.67517309355853783, -1.533254299341943128 ) ) ;
#7798=CARTESIAN_POINT ( 'NONE',  ( -249.7845036514871424, 11.60839712335144114, -1.818694302537078977 ) ) ;
#7803=LINE ( 'NONE', #2860, #10319 ) ;
#7804=LINE ( 'NONE', #2665, #7952 ) ;
#7809=ADVANCED_FACE ( 'NONE', ( #10620, #8498 ), #7683, .F. ) ;
#7810=ORIENTED_EDGE ( 'NONE', *, *, #10265, .F. ) ;
#7812=ORIENTED_EDGE ( 'NONE', *, *, #2578, .F. ) ;
#7814=CARTESIAN_POINT ( 'NONE',  ( 239.7985776503645354, -1.848645179573700004, 2.971954070984049956 ) ) ;
#7822=CARTESIAN_POINT ( 'NONE',  ( -247.5777789797446928, 9.724056904727886419, 6.595774163021543401 ) ) ;
#7823=ADVANCED_FACE ( 'NONE', ( #5554 ), #2625, .T. ) ;
#7824=ADVANCED_FACE ( 'NONE', ( #563 ), #3413, .F. ) ;
#7825=ORIENTED_EDGE ( 'NONE', *, *, #6723, .F. ) ;
#7829=CARTESIAN_POINT ( 'NONE',  ( -246.5049976578405051, 9.406509142110611066, -7.041467212631606465 ) ) ;
#7832=DIRECTION ( 'NONE',  ( 0.000000000000000000, 0.000000000000000000, 1.000000000000000000 ) ) ;
#7834=DIRECTION ( 'NONE',  ( 0.000000000000000000, 1.000000000000000000, 0.000000000000000000 ) ) ;
#7835=VECTOR ( 'NONE', #9253, 1000.000000000000000 ) ;
#7836=AXIS2_PLACEMENT_3D ( 'NONE', #5881, #3803, #12012 ) ;
#7837=DIRECTION ( 'NONE',  ( 0.000000000000000000, 0.000000000000000000, -1.000000000000000000 ) ) ;
#7845=CARTESIAN_POINT ( 'NONE',  ( -238.7984611738133651, -0.6745683551878548512, -11.73164972064059697 ) ) ;
#7849=EDGE_LOOP ( 'NONE', ( #4304, #642, #9850, #10500 ) ) ;
#7851=CARTESIAN_POINT ( 'NONE',  ( -248.9866437208148682, -10.23506904034385201, -5.772678315709418584 ) ) ;
#7852=ORIENTED_EDGE ( 'NONE', *, *, #11514, .F. ) ;
#7853=ADVANCED_FACE ( 'NONE', ( #11275 ), #6050, .F. ) ;
#7857=DIRECTION ( 'NONE',  ( 0.000000000000000000, 1.000000000000000000, 0.000000000000000000 ) ) ;
#7858=CARTESIAN_POINT ( 'NONE',  ( 122.2593324768346008, 18.00000000000000000, 174.7755348299889988 ) ) ;
#7859=CIRCLE ( 'NONE', #11269, 5.500000000000005329 ) ;
#7862=CARTESIAN_POINT ( 'NONE',  ( 0.000000000000000000, 11.79660968244690089, 0.000000000000000000 ) ) ;
#7864=CARTESIAN_POINT ( 'NONE',  ( 229.9934143309166075, 3.039192421457848958, 1.750862794997881666 ) ) ;
#7865=CARTESIAN_POINT ( 'NONE',  ( -249.7006323033828039, 11.24927497855769687, -3.394647652268084403 ) ) ;
#7872=EDGE_CURVE ( 'NONE', #7994, #6551, #3194, .T. ) ;
#7876=CARTESIAN_POINT ( 'NONE',  ( -240.1208361041844910, -2.772967769359084844, -11.41810622433049893 ) ) ;
#7879=FACE_OUTER_BOUND ( 'NONE', #3233, .T. ) ;
#7885=CARTESIAN_POINT ( 'NONE',  ( 240.1364042142084259, -2.243206690542109971, 2.686876444943266051 ) ) ;
#7886=VERTEX_POINT ( 'NONE', #6142 ) ;
#7890=DIRECTION ( 'NONE',  ( 0.000000000000000000, 0.000000000000000000, 1.000000000000000000 ) ) ;
#7897=CARTESIAN_POINT ( 'NONE',  ( -239.4550142662953078, 1.775421008909468634, 11.61532944475347584 ) ) ;
#7898=EDGE_LOOP ( 'NONE', ( #12387, #2115, #11802, #3718 ) ) ;
#7899=VECTOR ( 'NONE', #3636, 1000.000000000000000 ) ;
#7900=AXIS2_PLACEMENT_3D ( 'NONE', #12926, #10995, #4058 ) ;
#7901=EDGE_CURVE ( 'NONE', #5790, #11150, #1366, .T. ) ;
#7904=CARTESIAN_POINT ( 'NONE',  ( 240.0821326536456581, 2.149019271550664634, 2.771577408253355301 ) ) ;
#7906=DIRECTION ( 'NONE',  ( 0.000000000000000000, -1.000000000000000000, 0.000000000000000000 ) ) ;
#7908=DIRECTION ( 'NONE',  ( -1.000000000000000000, 0.000000000000000000, 0.000000000000000000 ) ) ;
#7912=ORIENTED_EDGE ( 'NONE', *, *, #4257, .F. ) ;
#7914=CARTESIAN_POINT ( 'NONE',  ( -239.1986675930642718, -1.476433817035277762, -11.65687006250814406 ) ) ;
#7915=AXIS2_PLACEMENT_3D ( 'NONE', #4523, #8798, #12667 ) ;
#7920=ORIENTED_EDGE ( 'NONE', *, *, #3621, .F. ) ;
#7925=AXIS2_PLACEMENT_3D ( 'NONE', #7748, #4737, #10677 ) ;
#7928=DIRECTION ( 'NONE',  ( 0.000000000000000000, 0.000000000000000000, -1.000000000000000000 ) ) ;
#7931=EDGE_CURVE ( 'NONE', #10501, #6584, #305, .T. ) ;
#7938=AXIS2_PLACEMENT_3D ( 'NONE', #6182, #10235, #12308 ) ;
#7942=DIRECTION ( 'NONE',  ( 0.000000000000000000, 1.000000000000000000, 0.000000000000000000 ) ) ;
#7943=CONICAL_SURFACE ( 'NONE', #3896, 6.500000000000005329, 0.7853981633974490562 ) ;
#7946=AXIS2_PLACEMENT_3D ( 'NONE', #2375, #4242, #5171 ) ;
#7947=CARTESIAN_POINT ( 'NONE',  ( 122.2593324768346008, 30.00000000000000000, 168.2755348299889988 ) ) ;
#7950=CARTESIAN_POINT ( 'NONE',  ( -240.1208361041834962, -2.772967769359314882, 11.41810622433041900 ) ) ;
#7952=VECTOR ( 'NONE', #2604, 999.9999999999998863 ) ;
#7954=DIRECTION ( 'NONE',  ( 0.000000000000000000, 1.000000000000000000, 0.000000000000000000 ) ) ;
#7959=AXIS2_PLACEMENT_3D ( 'NONE', #1966, #6039, #2887 ) ;
#7960=EDGE_CURVE ( 'NONE', #11915, #2131, #9877, .T. ) ;
#7962=ORIENTED_EDGE ( 'NONE', *, *, #3531, .F. ) ;
#7963=CARTESIAN_POINT ( 'NONE',  ( -249.5790707038086396, 10.95560708660684668, 4.250203461109054004 ) ) ;
#7972=CARTESIAN_POINT ( 'NONE',  ( -245.8522126038347437, 9.151584522525213927, -7.371153475566105229 ) ) ;
#7973=ORIENTED_EDGE ( 'NONE', *, *, #4288, .F. ) ;
#7976=TOROIDAL_SURFACE ( 'NONE', #1593, 238.4705882352940307, 2.000000000000000000 ) ;
#7978=CARTESIAN_POINT ( 'NONE',  ( 240.3599429726978087, 2.697249171176622884, 2.233886006030612936 ) ) ;
#7980=DIRECTION ( 'NONE',  ( 0.000000000000000000, 0.000000000000000000, -1.000000000000000000 ) ) ;
#7982=APPLICATION_CONTEXT ( 'automotive_design' ) ;
#7985=UNCERTAINTY_MEASURE_WITH_UNIT (LENGTH_MEASURE( 1.000000000000000082E-05 ), #9750, 'distance_accuracy_value', 'NONE');
#7987=ORIENTED_EDGE ( 'NONE', *, *, #10314, .T. ) ;
#7993=CARTESIAN_POINT ( 'NONE',  ( -249.7994463215831900, -11.74985191748826097, -0.3872576506385510542 ) ) ;
#7994=VERTEX_POINT ( 'NONE', #6283 ) ;
#7998=DIRECTION ( 'NONE',  ( 0.000000000000000000, 0.000000000000000000, -1.000000000000000000 ) ) ;
#7999=AXIS2_PLACEMENT_3D ( 'NONE', #6696, #9883, #3545 ) ;
#8001=FACE_OUTER_BOUND ( 'NONE', #8855, .T. ) ;
#8004=EDGE_CURVE ( 'NONE', #4811, #4563, #2266, .T. ) ;
#8009=ORIENTED_EDGE ( 'NONE', *, *, #7009, .T. ) ;
#8011=CARTESIAN_POINT ( 'NONE',  ( 0.000000000000000000, -3.327561323230890267, 0.000000000000000000 ) ) ;
#8012=ADVANCED_FACE ( 'NONE', ( #7205 ), #1375, .T. ) ;
#8013=CARTESIAN_POINT ( 'NONE',  ( -240.1208361041844910, 2.772967769358964940, -11.41810622433052025 ) ) ;
#8021=DIRECTION ( 'NONE',  ( 0.000000000000000000, -1.000000000000000000, 0.000000000000000000 ) ) ;
#8022=EDGE_LOOP ( 'NONE', ( #451, #1478 ) ) ;
#8023=ORIENTED_EDGE ( 'NONE', *, *, #5236, .F. ) ;
#8027=CARTESIAN_POINT ( 'NONE',  ( -249.1881502579952610, 10.41621036585313753, 5.437499737840824743 ) ) ;
#8028=ADVANCED_FACE ( 'NONE', ( #4199 ), #4980, .T. ) ;
#8031=CARTESIAN_POINT ( 'NONE',  ( -245.2557111572319855, 8.868800243844628284, 7.708496930521410384 ) ) ;
#8034=CARTESIAN_POINT ( 'NONE',  ( -239.1416205847678782, -1.396290246587958306, 11.66676345160061778 ) ) ;
#8036=CARTESIAN_POINT ( 'NONE',  ( -246.6649006626714424, 9.461692665233195854, -6.966985663954976538 ) ) ;
#8038=AXIS2_PLACEMENT_3D ( 'NONE', #11807, #10993, #10791 ) ;
#8041=EDGE_CURVE ( 'NONE', #8160, #7755, #10593, .T. ) ;
#8042=DIRECTION ( 'NONE',  ( 0.000000000000000000, 1.000000000000000000, 0.000000000000000000 ) ) ;
#8043=CARTESIAN_POINT ( 'NONE',  ( 239.4538130491550305, 1.465952997544165859, 3.178207852339172579 ) ) ;
#8045=DIRECTION ( 'NONE',  ( 8.659560562354913137E-17, -0.7071067811865489050, 0.7071067811865460184 ) ) ;
#8051=DIRECTION ( 'NONE',  ( 0.000000000000000000, 0.000000000000000000, 1.000000000000000000 ) ) ;
#8052=ORIENTED_EDGE ( 'NONE', *, *, #6441, .F. ) ;
#8053=CARTESIAN_POINT ( 'NONE',  ( -249.1369139481503794, -10.36343465104323869, 5.538914405783208039 ) ) ;
#8054=ORIENTED_EDGE ( 'NONE', *, *, #3655, .T. ) ;
#8055=CIRCLE ( 'NONE', #8910, 240.3921568627444856 ) ;
#8060=CARTESIAN_POINT ( 'NONE',  ( -242.5648157360982964, -6.889953639954495834, -9.518299936636116954 ) ) ;
#8063=CIRCLE ( 'NONE', #2309, 5.500000000000005329 ) ;
#8065=DIRECTION ( 'NONE',  ( 8.659560562354963673E-17, 0.7071067811865450192, -0.7071067811865500152 ) ) ;
#8066=CIRCLE ( 'NONE', #192, 6.499999999999999112 ) ;
#8067=AXIS2_PLACEMENT_3D ( 'NONE', #4549, #5434, #8631 ) ;
#8068=VECTOR ( 'NONE', #5964, 1000.000000000000114 ) ;
#8069=CARTESIAN_POINT ( 'NONE',  ( 3.059167704270087661E-14, 25.50000000000000000, -249.7999999999999545 ) ) ;
#8075=DIRECTION ( 'NONE',  ( 0.000000000000000000, 0.000000000000000000, 1.000000000000000000 ) ) ;
#8076=ADVANCED_FACE ( 'NONE', ( #6920, #11979, #10662, #783, #11912, #10979, #722, #5532, #2831, #1851, #1535, #2400, #6849, #5914, #2528 ), #4773, .F. ) ;
#8078=CARTESIAN_POINT ( 'NONE',  ( -239.7946578092510208, 2.116498006234943219, -11.55893420607628563 ) ) ;
#8079=AXIS2_PLACEMENT_3D ( 'NONE', #1389, #6461, #389 ) ;
#8084=CARTESIAN_POINT ( 'NONE',  ( -243.0711418327976219, -7.372150984762692261, 9.149572407291026721 ) ) ;
#8086=ORIENTED_EDGE ( 'NONE', *, *, #8041, .T. ) ;
#8088=FACE_BOUND ( 'NONE', #12241, .T. ) ;
#8091=ORIENTED_EDGE ( 'NONE', *, *, #624, .F. ) ;
#8092=EDGE_LOOP ( 'NONE', ( #9199, #5476, #698, #9236 ) ) ;
#8094=CARTESIAN_POINT ( 'NONE',  ( 197.8197553893920144, 19.00000000000000000, 58.77553482998850853 ) ) ;
#8096=DIRECTION ( 'NONE',  ( 0.000000000000000000, 0.000000000000000000, -1.000000000000000000 ) ) ;
#8099=AXIS2_PLACEMENT_3D ( 'NONE', #8998, #5799, #10857 ) ;
#8101=CARTESIAN_POINT ( 'NONE',  ( -245.6948533149643765, 9.079155719285296300, 7.458842562578837487 ) ) ;
#8103=FACE_OUTER_BOUND ( 'NONE', #9584, .T. ) ;
#8107=CIRCLE ( 'NONE', #2762, 5.499999999999998224 ) ;
#8108=CYLINDRICAL_SURFACE ( 'NONE', #1822, 245.7999999999999829 ) ;
#8111=DIRECTION ( 'NONE',  ( 0.000000000000000000, -1.000000000000000000, 0.000000000000000000 ) ) ;
#8112=CARTESIAN_POINT ( 'NONE',  ( -210.0000000000000000, 19.40000000000000213, 0.000000000000000000 ) ) ;
#8114=CARTESIAN_POINT ( 'NONE',  ( -122.2593324768359935, 29.00000000000000000, -173.7755348299880040 ) ) ;
#8119=CARTESIAN_POINT ( 'NONE',  ( -238.7110724325390834, -0.02063703527941252586, -11.74998174837370968 ) ) ;
#8121=CARTESIAN_POINT ( 'NONE',  ( 197.8197553893915028, 19.00000000000000000, -69.77553482998990830 ) ) ;
#8122=ORIENTED_EDGE ( 'NONE', *, *, #12656, .T. ) ;
#8124=CIRCLE ( 'NONE', #6392, 10.00000000000000888 ) ;
#8125=CARTESIAN_POINT ( 'NONE',  ( -249.6835501130389048, 11.19967427147338590, -3.553901703851193083 ) ) ;
#8127=CARTESIAN_POINT ( 'NONE',  ( -122.2593324768359935, 19.00000000000000000, -168.2755348299880040 ) ) ;
#8128=ORIENTED_EDGE ( 'NONE', *, *, #1992, .F. ) ;
#8134=CARTESIAN_POINT ( 'NONE',  ( -246.7156022646194629, -9.478660876070511776, -6.943882023634849077 ) ) ;
#8135=CARTESIAN_POINT ( 'NONE',  ( -122.2593324768321992, 18.00000000000000000, 161.7755348299905052 ) ) ;
#8139=DIRECTION ( 'NONE',  ( 0.000000000000000000, -1.000000000000000000, 0.000000000000000000 ) ) ;
#8144=AXIS2_PLACEMENT_3D ( 'NONE', #12106, #4971, #178 ) ;
#8147=FACE_OUTER_BOUND ( 'NONE', #7299, .T. ) ;
#8148=VECTOR ( 'NONE', #550, 1000.000000000000000 ) ;
#8149=CARTESIAN_POINT ( 'NONE',  ( 0.000000000000000000, 30.00000000000000000, -208.0000000000000000 ) ) ;
#8152=AXIS2_PLACEMENT_3D ( 'NONE', #2667, #8748, #3675 ) ;
#8153=CARTESIAN_POINT ( 'NONE',  ( -240.7240246252840734, -4.307698619074218804, 10.93373802362567027 ) ) ;
#8155=VERTEX_POINT ( 'NONE', #913 ) ;
#8158=ADVANCED_FACE ( 'NONE', ( #979 ), #2896, .F. ) ;
#8159=DIRECTION ( 'NONE',  ( 0.000000000000000000, 0.000000000000000000, -1.000000000000000000 ) ) ;
#8160=VERTEX_POINT ( 'NONE', #11039 ) ;
#8163=CARTESIAN_POINT ( 'NONE',  ( 0.000000000000000000, 19.00000000000000000, 208.0000000000000000 ) ) ;
#8170=CARTESIAN_POINT ( 'NONE',  ( -242.3794917440154961, 6.695067658262285448, 9.656064787098769031 ) ) ;
#8171=ORIENTED_EDGE ( 'NONE', *, *, #8004, .T. ) ;
#8173=AXIS2_PLACEMENT_3D ( 'NONE', #1833, #4614, #3754 ) ;
#8176=VERTEX_POINT ( 'NONE', #1978 ) ;
#8177=AXIS2_PLACEMENT_3D ( 'NONE', #9736, #621, #10811 ) ;
#8179=ORIENTED_EDGE ( 'NONE', *, *, #4159, .F. ) ;
#8182=LINE ( 'NONE', #11035, #1051 ) ;
#8188=CARTESIAN_POINT ( 'NONE',  ( -122.2593324768321992, 30.00000000000000000, 173.7755348299905052 ) ) ;
#8189=AXIS2_PLACEMENT_3D ( 'NONE', #3257, #9523, #1464 ) ;
#8190=CARTESIAN_POINT ( 'NONE',  ( 71.82423009839129691, 30.00000000000000000, -203.8354503650404865 ) ) ;
#8191=ORIENTED_EDGE ( 'NONE', *, *, #11372, .F. ) ;
#8193=EDGE_LOOP ( 'NONE', ( #8179, #5015, #1444, #3920 ) ) ;
#8194=CARTESIAN_POINT ( 'NONE',  ( -249.0239419981220124, 10.26696505005539350, -5.714577088569218866 ) ) ;
#8198=CARTESIAN_POINT ( 'NONE',  ( -249.6369960391978680, -11.07262528782856670, 3.948341303013173764 ) ) ;
#8203=EDGE_CURVE ( 'NONE', #6584, #10068, #3970, .T. ) ;
#8204=CARTESIAN_POINT ( 'NONE',  ( -243.8684449830084020, -8.017731004131830375, -8.590997629223123155 ) ) ;
#8209=CARTESIAN_POINT ( 'NONE',  ( -229.9250651581393754, -10.17993753377408872, 5.880500963262212721 ) ) ;
#8210=EDGE_CURVE ( 'NONE', #2492, #3412, #396, .T. ) ;
#8218=AXIS2_PLACEMENT_3D ( 'NONE', #6307, #2231, #9300 ) ;
#8220=DIRECTION ( 'NONE',  ( 0.000000000000000000, 0.000000000000000000, 1.000000000000000000 ) ) ;
#8224=CARTESIAN_POINT ( 'NONE',  ( -244.6749594711698705, -8.549245790843562176, 8.062606907241317344 ) ) ;
#8228=CARTESIAN_POINT ( 'NONE',  ( 197.8197553893920144, 19.00000000000000000, 69.77553482998851564 ) ) ;
#8230=ORIENTED_EDGE ( 'NONE', *, *, #3606, .T. ) ;
#8231=EDGE_LOOP ( 'NONE', ( #7962, #502, #2840, #6138 ) ) ;
#8232=CARTESIAN_POINT ( 'NONE',  ( -197.8197553893924976, 19.00000000000000000, -69.77553482998720824 ) ) ;
#8234=EDGE_CURVE ( 'NONE', #4193, #612, #1157, .T. ) ;
#8238=CARTESIAN_POINT ( 'NONE',  ( -244.2426106971964543, 8.274791045078206508, 8.342083836226366955 ) ) ;
#8241=ORIENTED_EDGE ( 'NONE', *, *, #11372, .T. ) ;
#8244=ORIENTED_EDGE ( 'NONE', *, *, #3436, .T. ) ;
#8245=DIRECTION ( 'NONE',  ( 0.000000000000000000, -1.000000000000000000, 0.000000000000000000 ) ) ;
#8247=CARTESIAN_POINT ( 'NONE',  ( 239.0281511860673049, 0.5135531388252957408, 3.462181616324999212 ) ) ;
#8254=VERTEX_POINT ( 'NONE', #6445 ) ;
#8255=LINE ( 'NONE', #6258, #1565 ) ;
#8256=AXIS2_PLACEMENT_3D ( 'NONE', #12586, #12709, #524 ) ;
#8259=DIRECTION ( 'NONE',  ( 0.000000000000000000, 0.000000000000000000, -1.000000000000000000 ) ) ;
#8260=ADVANCED_FACE ( 'NONE', ( #2497 ), #103, .F. ) ;
#8261=CARTESIAN_POINT ( 'NONE',  ( -249.7900429577784678, -11.65124970439946139, 1.521630468629134203 ) ) ;
#8265=LINE ( 'NONE', #4185, #407 ) ;
#8266=CARTESIAN_POINT ( 'NONE',  ( -242.4885533050452580, -6.811171350273821368, -9.574815118338978692 ) ) ;
#8267=CARTESIAN_POINT ( 'NONE',  ( 239.4667603742667836, -1.483520951478357830, 3.170043417407540698 ) ) ;
#8274=FACE_OUTER_BOUND ( 'NONE', #189, .T. ) ;
#8275=VERTEX_POINT ( 'NONE', #11380 ) ;
#8278=CARTESIAN_POINT ( 'NONE',  ( -197.8197553893924976, 19.00000000000000000, -69.77553482998720824 ) ) ;
#8280=DIRECTION ( 'NONE',  ( 0.000000000000000000, 0.000000000000000000, -1.000000000000000000 ) ) ;
#8283=LINE ( 'NONE', #3261, #3445 ) ;
#8284=VECTOR ( 'NONE', #4328, 1000.000000000000000 ) ;
#8289=DIRECTION ( 'NONE',  ( 0.000000000000000000, 1.000000000000000000, 0.000000000000000000 ) ) ;
#8291=CARTESIAN_POINT ( 'NONE',  ( 240.3826708216974737, -2.772967769359219847, 2.135567781667135012 ) ) ;
#8292=ADVANCED_FACE ( 'NONE', ( #4491 ), #7549, .F. ) ;
#8293=CARTESIAN_POINT ( 'NONE',  ( 229.9760321542115662, -1.127100313231406803, -3.321498603606710898 ) ) ;
#8296=AXIS2_PLACEMENT_3D ( 'NONE', #5999, #12125, #12326 ) ;
#8297=CARTESIAN_POINT ( 'NONE',  ( 240.1760274753965518, -2.306688218040592986, 2.632364499240650968 ) ) ;
#8299=AXIS2_PLACEMENT_3D ( 'NONE', #9372, #238, #4296 ) ;
#8303=CARTESIAN_POINT ( 'NONE',  ( -243.2454781773737977, 7.524012760887466733, 9.025130269038724506 ) ) ;
#8305=CONICAL_SURFACE ( 'NONE', #12974, 195.0000000000000000, 0.7853981633974476129 ) ;
#8306=EDGE_LOOP ( 'NONE', ( #1883, #4291, #6383, #4095 ) ) ;
#8308=VERTEX_POINT ( 'NONE', #9376 ) ;
#8309=DIRECTION ( 'NONE',  ( 0.000000000000000000, 0.000000000000000000, -1.000000000000000000 ) ) ;
#8312=VECTOR ( 'NONE', #5130, 1000.000000000000000 ) ;
#8313=CARTESIAN_POINT ( 'NONE',  ( -210.0000000000000000, 18.00000000000000000, 0.000000000000000000 ) ) ;
#8314=DIRECTION ( 'NONE',  ( 0.000000000000000000, 0.000000000000000000, -1.000000000000000000 ) ) ;
#8317=DIRECTION ( 'NONE',  ( 0.000000000000000000, 0.000000000000000000, 1.000000000000000000 ) ) ;
#8322=ORIENTED_EDGE ( 'NONE', *, *, #1571, .T. ) ;
#8323=DIRECTION ( 'NONE',  ( 8.659560562354926695E-17, -0.7071067811865480168, 0.7071067811865470176 ) ) ;
#8326=EDGE_CURVE ( 'NONE', #10046, #11448, #3625, .T. ) ;
#8328=CARTESIAN_POINT ( 'NONE',  ( -249.7846912502906207, -11.60973349240726549, 1.810138451173344931 ) ) ;
#8333=CARTESIAN_POINT ( 'NONE',  ( -242.2164292014763305, -6.515245625945103924, -9.778246362750261156 ) ) ;
#8335=CARTESIAN_POINT ( 'NONE',  ( 239.2087834361827277, -1.051957556907570090, 3.338183402683874146 ) ) ;
#8337=DIRECTION ( 'NONE',  ( -1.000000000000000000, -0.000000000000000000, -0.000000000000000000 ) ) ;
#8338=AXIS2_PLACEMENT_3D ( 'NONE', #2826, #2692, #9969 ) ;
#8341=CONICAL_SURFACE ( 'NONE', #247, 6.500000000000005329, 0.7853981633974490562 ) ;
#8345=CARTESIAN_POINT ( 'NONE',  ( 3.053044470274351535E-14, 30.00000000000000000, 248.7999999999999829 ) ) ;
#8346=CARTESIAN_POINT ( 'NONE',  ( 239.2711857403947988, -1.179132569181245316, -3.296284915250143221 ) ) ;
#8347=CARTESIAN_POINT ( 'NONE',  ( 71.82423009839129691, 19.40000000000000213, -197.3354503650404865 ) ) ;
#8351=CARTESIAN_POINT ( 'NONE',  ( -197.8197553893909912, 30.00000000000000000, 64.27553482999130097 ) ) ;
#8353=DIRECTION ( 'NONE',  ( 0.000000000000000000, 1.000000000000000000, 0.000000000000000000 ) ) ;
#8355=B_SPLINE_CURVE_WITH_KNOTS ( 'NONE', 3,
 ( #10972, #7897, #3901, #2958, #11970, #6043, #3762, #12037, #840, #2144, #2750, #2889, #10096, #1842, #6839, #8839, #11031, #10900, #970, #12167, #5846, #778, #11099 ),
 .UNSPECIFIED., .F., .F.,
 ( 4, 2, 2, 1, 1, 2, 2, 2, 2, 1, 2, 2, 4 ),
 ( 0.000000000000000000, 0.06250953674349737921, 0.09376430511523958788, 0.1093916893011107061, 0.1172053813940463346, 0.1211122274405143084, 0.1250190734869822962, 0.1875286102303734270, 0.2187833786020739191, 0.2344107627879288558, 0.2422244548808562548, 0.2500381469737836260, 0.5000762939474624469 ),
 .UNSPECIFIED. ) ;
#8357=LINE ( 'NONE', #7284, #1715 ) ;
#8358=CARTESIAN_POINT ( 'NONE',  ( 229.9733680233430846, -0.2312567328850919368, 3.499999999999965361 ) ) ;
#8359=ORIENTED_EDGE ( 'NONE', *, *, #8511, .T. ) ;
#8360=VERTEX_POINT ( 'NONE', #4818 ) ;
#8361=DIRECTION ( 'NONE',  ( 0.000000000000000000, 0.000000000000000000, 1.000000000000000000 ) ) ;
#8364=ADVANCED_FACE ( 'NONE', ( #6642 ), #7631, .F. ) ;
#8365=DIRECTION ( 'NONE',  ( 0.000000000000000000, -1.000000000000000000, 0.000000000000000000 ) ) ;
#8368=B_SPLINE_CURVE_WITH_KNOTS ( 'NONE', 3,
 ( #8013, #2620, #3691, #9620, #9687, #8078, #703, #6707 ),
 .UNSPECIFIED., .F., .F.,
 ( 4, 2, 2, 4 ),
 ( 0.000000000000000000, 0.2500000000000095479, 0.5000000000000190958, 1.000000000000000000 ),
 .UNSPECIFIED. ) ;
#8369=CARTESIAN_POINT ( 'NONE',  ( 122.2593324768334071, 30.00000000000000000, -168.2755348299895104 ) ) ;
#8370=ORIENTED_EDGE ( 'NONE', *, *, #2370, .T. ) ;
#8375=ORIENTED_EDGE ( 'NONE', *, *, #5385, .F. ) ;
#8377=AXIS2_PLACEMENT_3D ( 'NONE', #7947, #13011, #10011 ) ;
#8380=FACE_BOUND ( 'NONE', #8386, .T. ) ;
#8382=LINE ( 'NONE', #11438, #6662 ) ;
#8383=CARTESIAN_POINT ( 'NONE',  ( -238.7112176159036778, 0.03609691783649805058, -11.74994919738963439 ) ) ;
#8386=EDGE_LOOP ( 'NONE', ( #1002, #8903 ) ) ;
#8388=CARTESIAN_POINT ( 'NONE',  ( 6.735557395310435121E-16, 19.00000000000000000, 202.4999999999999716 ) ) ;
#8389=ORIENTED_EDGE ( 'NONE', *, *, #2540, .T. ) ;
#8390=DIRECTION ( 'NONE',  ( 0.000000000000000000, 0.000000000000000000, 1.000000000000000000 ) ) ;
#8395=CARTESIAN_POINT ( 'NONE',  ( 0.000000000000000000, 0.000000000000000000, 0.000000000000000000 ) ) ;
#8396=CARTESIAN_POINT ( 'NONE',  ( 197.8197553893915028, 29.00000000000000000, -69.77553482998990830 ) ) ;
#8398=CARTESIAN_POINT ( 'NONE',  ( -229.9801196668058481, 11.35475723081091992, 3.046485053526966968 ) ) ;
#8399=EDGE_CURVE ( 'NONE', #11942, #12887, #9826, .T. ) ;
#8403=AXIS2_PLACEMENT_3D ( 'NONE', #5305, #9560, #443 ) ;
#8404=DIRECTION ( 'NONE',  ( 0.000000000000000000, 1.000000000000000000, 0.000000000000000000 ) ) ;
#8409=CARTESIAN_POINT ( 'NONE',  ( -249.2689385757807941, 10.50219330951863306, 5.269387968809968292 ) ) ;
#8411=CIRCLE ( 'NONE', #11167, 6.500000000000005329 ) ;
#8417=CARTESIAN_POINT ( 'NONE',  ( 197.8197553893915028, 29.00000000000000000, -58.77553482998990830 ) ) ;
#8419=ORIENTED_EDGE ( 'NONE', *, *, #9595, .T. ) ;
#8420=CARTESIAN_POINT ( 'NONE',  ( 0.000000000000000000, 18.00000000000000000, 201.4999999999999716 ) ) ;
#8422=CARTESIAN_POINT ( 'NONE',  ( 229.9901773315476987, -2.783473308305698168, -2.134081248093457006 ) ) ;
#8423=ORIENTED_EDGE ( 'NONE', *, *, #1510, .F. ) ;
#8434=CARTESIAN_POINT ( 'NONE',  ( -197.8197553893924976, 30.00000000000000000, -69.77553482998720824 ) ) ;
#8436=ORIENTED_EDGE ( 'NONE', *, *, #3506, .T. ) ;
#8439=ORIENTED_EDGE ( 'NONE', *, *, #9485, .T. ) ;
#8442=EDGE_CURVE ( 'NONE', #12258, #5446, #12895, .T. ) ;
#8444=DIRECTION ( 'NONE',  ( 0.000000000000000000, -1.000000000000000000, 0.000000000000000000 ) ) ;
#8447=CARTESIAN_POINT ( 'NONE',  ( 238.9937480947141353, 0.3586231075815122793, -3.486222115670320587 ) ) ;
#8448=ADVANCED_FACE ( 'NONE', ( #10966 ), #5697, .F. ) ;
#8449=DIRECTION ( 'NONE',  ( 0.000000000000000000, 0.000000000000000000, -1.000000000000000000 ) ) ;
#8451=CARTESIAN_POINT ( 'NONE',  ( 0.000000000000000000, 11.79660968244690089, 0.000000000000000000 ) ) ;
#8454=DIRECTION ( 'NONE',  ( 0.000000000000000000, 0.000000000000000000, -1.000000000000000000 ) ) ;
#8458=CARTESIAN_POINT ( 'NONE',  ( 0.000000000000000000, 1.848645179567965036, 239.8169934640517624 ) ) ;
#8465=DIRECTION ( 'NONE',  ( 0.000000000000000000, 1.000000000000000000, 0.000000000000000000 ) ) ;
#8467=CARTESIAN_POINT ( 'NONE',  ( 240.3826708216974737, 2.772967769358989809, -2.135567781667440102 ) ) ;
#8468=FACE_OUTER_BOUND ( 'NONE', #1288, .T. ) ;
#8472=CARTESIAN_POINT ( 'NONE',  ( 0.000000000000000000, 22.00000000000000000, 0.000000000000000000 ) ) ;
#8475=CARTESIAN_POINT ( 'NONE',  ( 3.059167704270088292E-14, 21.50000000000000000, 249.7999999999999829 ) ) ;
#8479=FACE_OUTER_BOUND ( 'NONE', #8808, .T. ) ;
#8481=DIRECTION ( 'NONE',  ( 0.000000000000000000, 1.000000000000000000, 0.000000000000000000 ) ) ;
#8486=ADVANCED_FACE ( 'NONE', ( #570 ), #10698, .T. ) ;
#8489=VECTOR ( 'NONE', #11750, 1000.000000000000000 ) ;
#8493=CARTESIAN_POINT ( 'NONE',  ( 0.000000000000000000, 11.79660968244690089, 0.000000000000000000 ) ) ;
#8497=VERTEX_POINT ( 'NONE', #12762 ) ;
#8498=FACE_OUTER_BOUND ( 'NONE', #4027, .T. ) ;
#8505=VECTOR ( 'NONE', #8598, 1000.000000000000000 ) ;
#8511=EDGE_CURVE ( 'NONE', #157, #1185, #2744, .T. ) ;
#8512=ADVANCED_FACE ( 'NONE', ( #1770 ), #2850, .F. ) ;
#8517=ORIENTED_EDGE ( 'NONE', *, *, #5236, .T. ) ;
#8518=LINE ( 'NONE', #5174, #4009 ) ;
#8522=CIRCLE ( 'NONE', #2746, 248.1666666666679930 ) ;
#8528=CARTESIAN_POINT ( 'NONE',  ( 197.8197553893915028, 19.00000000000000000, -69.77553482998990830 ) ) ;
#8534=CIRCLE ( 'NONE', #1291, 239.8169934640564804 ) ;
#8535=DIRECTION ( 'NONE',  ( 0.000000000000000000, 0.000000000000000000, 1.000000000000000000 ) ) ;
#8545=CARTESIAN_POINT ( 'NONE',  ( -238.7109915808064500, 2.244475480116206709E-14, 11.74999999995203126 ) ) ;
#8550=VERTEX_POINT ( 'NONE', #33 ) ;
#8551=ORIENTED_EDGE ( 'NONE', *, *, #2059, .F. ) ;
#8556=AXIS2_PLACEMENT_3D ( 'NONE', #10230, #10931, #2986 ) ;
#8571=LINE ( 'NONE', #10361, #1739 ) ;
#8573=CIRCLE ( 'NONE', #4308, 249.7999999999999829 ) ;
#8574=CARTESIAN_POINT ( 'NONE',  ( 239.7985776503625175, 1.848645179571945185, -2.971954070985139751 ) ) ;
#8579=ORIENTED_EDGE ( 'NONE', *, *, #1085, .F. ) ;
#8592=CARTESIAN_POINT ( 'NONE',  ( -240.4375400851813822, -3.701007121282966494, -11.16264886370965570 ) ) ;
#8598=DIRECTION ( 'NONE',  ( 8.659560562354926695E-17, 0.7071067811865480168, -0.7071067811865470176 ) ) ;
#8599=EDGE_LOOP ( 'NONE', ( #12356, #7654 ) ) ;
#8603=CARTESIAN_POINT ( 'NONE',  ( 197.8197553893915028, 29.00000000000000000, -64.27553482998990830 ) ) ;
#8604=CARTESIAN_POINT ( 'NONE',  ( -197.8197553893924976, 19.00000000000000000, -64.27553482998719403 ) ) ;
#8612=CARTESIAN_POINT ( 'NONE',  ( -229.7367722661449250, -4.144097499581555155, -11.00169393300851084 ) ) ;
#8615=CARTESIAN_POINT ( 'NONE',  ( 71.82423009839129691, 18.00000000000000000, 197.3354503650404865 ) ) ;
#8617=ORIENTED_EDGE ( 'NONE', *, *, #13037, .F. ) ;
#8621=CARTESIAN_POINT ( 'NONE',  ( 0.000000000000000000, 29.00000000000000000, 213.5000000000000000 ) ) ;
#8623=DIRECTION ( 'NONE',  ( 0.000000000000000000, 1.000000000000000000, 0.000000000000000000 ) ) ;
#8625=DIRECTION ( 'NONE',  ( 0.000000000000000000, 1.000000000000000000, 0.000000000000000000 ) ) ;
#8627=MECHANICAL_DESIGN_GEOMETRIC_PRESENTATION_REPRESENTATION('',(#9477),#8841);
#8630=ORIENTED_EDGE ( 'NONE', *, *, #10626, .F. ) ;
#8631=DIRECTION ( 'NONE',  ( 0.000000000000000000, 0.000000000000000000, 1.000000000000000000 ) ) ;
#8632=ORIENTED_EDGE ( 'NONE', *, *, #6958, .F. ) ;
#8634=VECTOR ( 'NONE', #12589, 1000.000000000000114 ) ;
#8635=DIRECTION ( 'NONE',  ( 0.000000000000000000, -0.7071067811865489050, -0.7071067811865460184 ) ) ;
#8641=FACE_BOUND ( 'NONE', #12052, .T. ) ;
#8647=CARTESIAN_POINT ( 'NONE',  ( -241.0175249737202989, 4.851820797274892350, -10.70187039120737005 ) ) ;
#8649=EDGE_CURVE ( 'NONE', #5629, #1965, #8782, .T. ) ;
#8653=CARTESIAN_POINT ( 'NONE',  ( -229.7304563602428402, 3.778965902296226975, 11.13238168007022288 ) ) ;
#8662=FACE_OUTER_BOUND ( 'NONE', #11960, .T. ) ;
#8664=DIRECTION ( 'NONE',  ( 0.000000000000000000, 0.000000000000000000, -1.000000000000000000 ) ) ;
#8667=CARTESIAN_POINT ( 'NONE',  ( 229.9733680233429993, 8.492964294626340574E-17, 3.499999999999964917 ) ) ;
#8669=ADVANCED_FACE ( 'NONE', ( #2418 ), #10059, .F. ) ;
#8673=ORIENTED_EDGE ( 'NONE', *, *, #4371, .T. ) ;
#8675=LINE ( 'NONE', #4598, #4630 ) ;
#8676=CARTESIAN_POINT ( 'NONE',  ( 122.2593324768334071, 19.00000000000000000, -173.7755348299895104 ) ) ;
#8680=DIRECTION ( 'NONE',  ( 0.000000000000000000, 0.000000000000000000, 1.000000000000000000 ) ) ;
#8681=DIRECTION ( 'NONE',  ( 0.000000000000000000, 1.000000000000000000, 0.000000000000000000 ) ) ;
#8688=ORIENTED_EDGE ( 'NONE', *, *, #2555, .T. ) ;
#8694=DIRECTION ( 'NONE',  ( 0.000000000000000000, 0.000000000000000000, 1.000000000000000000 ) ) ;
#8695=DIRECTION ( 'NONE',  ( -1.000000000000000000, -0.000000000000000000, -0.000000000000000000 ) ) ;
#8698=CIRCLE ( 'NONE', #12108, 5.500000000000005329 ) ;
#8704=ORIENTED_EDGE ( 'NONE', *, *, #10314, .F. ) ;
#8705=CARTESIAN_POINT ( 'NONE',  ( -244.6749594661061167, 8.549245787831393883, -8.062606910321274967 ) ) ;
#8708=AXIS2_PLACEMENT_3D ( 'NONE', #11464, #3318, #8535 ) ;
#8710=CARTESIAN_POINT ( 'NONE',  ( 240.2816503055146882, -2.505215826205224872, -2.444791323730728827 ) ) ;
#8711=CARTESIAN_POINT ( 'NONE',  ( -122.2593324768359935, 30.00000000000000000, -161.7755348299880040 ) ) ;
#8716=DIRECTION ( 'NONE',  ( 0.000000000000000000, -1.000000000000000000, 0.000000000000000000 ) ) ;
#8721=ADVANCED_FACE ( 'NONE', ( #12485 ), #9360, .F. ) ;
#8722=VECTOR ( 'NONE', #6015, 1000.000000000000114 ) ;
#8723=ORIENTED_EDGE ( 'NONE', *, *, #7224, .F. ) ;
#8726=CARTESIAN_POINT ( 'NONE',  ( -248.9051445895378833, -10.17462340911300522, -5.878044170152538328 ) ) ;
#8727=EDGE_LOOP ( 'NONE', ( #434, #5627, #5686, #1987, #2491, #7920, #3271, #1620, #8853, #5294 ) ) ;
#8730=LINE ( 'NONE', #6932, #1253 ) ;
#8731=CARTESIAN_POINT ( 'NONE',  ( 197.8197553893920144, 29.00000000000000000, 58.77553482998850853 ) ) ;
#8733=CARTESIAN_POINT ( 'NONE',  ( -239.9867712987591801, -2.433335514368112129, 11.49559079283389096 ) ) ;
#8736=CARTESIAN_POINT ( 'NONE',  ( -229.7036025737252203, -1.539969265571519363, -11.67378731463722019 ) ) ;
#8737=AXIS2_PLACEMENT_3D ( 'NONE', #10666, #12671, #1669 ) ;
#8738=CARTESIAN_POINT ( 'NONE',  ( -249.7276455219525815, 11.33491751851197549, 3.110604576379348174 ) ) ;
#8739=DIRECTION ( 'NONE',  ( 0.000000000000000000, 1.000000000000000000, 0.000000000000000000 ) ) ;
#8743=CARTESIAN_POINT ( 'NONE',  ( 0.000000000000000000, -20.00000000000000000, 0.000000000000000000 ) ) ;
#8748=DIRECTION ( 'NONE',  ( 0.000000000000000000, 1.000000000000000000, 0.000000000000000000 ) ) ;
#8750=DIRECTION ( 'NONE',  ( 0.000000000000000000, 1.000000000000000000, 0.000000000000000000 ) ) ;
#8751=FACE_BOUND ( 'NONE', #9238, .T. ) ;
#8754=EDGE_LOOP ( 'NONE', ( #144, #4799, #7223, #6326 ) ) ;
#8758=EDGE_LOOP ( 'NONE', ( #7973, #9035, #10770, #2381 ) ) ;
#8760=ORIENTED_EDGE ( 'NONE', *, *, #11124, .F. ) ;
#8761=ADVANCED_FACE ( 'NONE', ( #5358 ), #3214, .T. ) ;
#8764=CARTESIAN_POINT ( 'NONE',  ( -122.2593324768321992, 30.00000000000000000, 168.2755348299905052 ) ) ;
#8765=( NAMED_UNIT ( * ) PLANE_ANGLE_UNIT ( ) SI_UNIT ( $, .RADIAN. ) );
#8766=CARTESIAN_POINT ( 'NONE',  ( 3.053044470274351535E-14, 25.00000000000000000, -249.2999999999999829 ) ) ;
#8767=ADVANCED_FACE ( 'NONE', ( #359 ), #10285, .F. ) ;
#8772=CARTESIAN_POINT ( 'NONE',  ( -243.1145437067741852, 7.410518231008048851, -9.118492838939154410 ) ) ;
#8776=CARTESIAN_POINT ( 'NONE',  ( 122.2593324768334071, 30.00000000000000000, -174.7755348299895104 ) ) ;
#8777=FACE_OUTER_BOUND ( 'NONE', #6927, .T. ) ;
#8778=VECTOR ( 'NONE', #9797, 1000.000000000000000 ) ;
#8779=CARTESIAN_POINT ( 'NONE',  ( 3.010181832304193602E-14, 0.000000000000000000, 245.7999999999999829 ) ) ;
#8782=CIRCLE ( 'NONE', #1116, 249.7999999999999829 ) ;
#8784=ORIENTED_EDGE ( 'NONE', *, *, #12515, .T. ) ;
#8788=ORIENTED_EDGE ( 'NONE', *, *, #8004, .F. ) ;
#8791=AXIS2_PLACEMENT_3D ( 'NONE', #4269, #10269, #7402 ) ;
#8793=CARTESIAN_POINT ( 'NONE',  ( -122.2593324768321992, 30.00000000000000000, 174.7755348299905052 ) ) ;
#8795=EDGE_CURVE ( 'NONE', #12496, #534, #12615, .T. ) ;
#8797=DIRECTION ( 'NONE',  ( 8.659560562355171982E-17, 0.7071067811865280328, -0.7071067811865670016 ) ) ;
#8798=DIRECTION ( 'NONE',  ( 0.000000000000000000, -1.000000000000000000, 0.000000000000000000 ) ) ;
#8800=VECTOR ( 'NONE', #5764, 1000.000000000000000 ) ;
#8801=CARTESIAN_POINT ( 'NONE',  ( -229.9800961966465707, -11.35427705715375168, -3.048062575764186821 ) ) ;
#8803=CONICAL_SURFACE ( 'NONE', #12218, 5.500000000000005329, 0.7853981633974461696 ) ;
#8804=CARTESIAN_POINT ( 'NONE',  ( -249.3500139047057473, 10.59807002901562001, -5.074486595297502234 ) ) ;
#8807=EDGE_LOOP ( 'NONE', ( #3206, #3977, #10295, #5791 ) ) ;
#8808=EDGE_LOOP ( 'NONE', ( #7395, #7353, #2977, #2722 ) ) ;
#8809=DIRECTION ( 'NONE',  ( 0.000000000000000000, 1.000000000000000000, 0.000000000000000000 ) ) ;
#8810=CARTESIAN_POINT ( 'NONE',  ( 0.000000000000000000, 0.000000000000000000, -245.7999999999999829 ) ) ;
#8811=ADVANCED_FACE ( 'NONE', ( #11626 ), #5379, .T. ) ;
#8818=FACE_OUTER_BOUND ( 'NONE', #6205, .T. ) ;
#8819=CARTESIAN_POINT ( 'NONE',  ( 240.2701176883045093, 2.464548987102257449, -2.493043655922373425 ) ) ;
#8821=EDGE_CURVE ( 'NONE', #1614, #5331, #12823, .T. ) ;
#8827=ORIENTED_EDGE ( 'NONE', *, *, #5254, .T. ) ;
#8828=CARTESIAN_POINT ( 'NONE',  ( 197.8197553893915028, 18.00000000000000000, -70.77553482998990830 ) ) ;
#8829=CARTESIAN_POINT ( 'NONE',  ( 239.0281511860549699, -0.5135531387677250148, -3.462181616333541712 ) ) ;
#8831=AXIS2_PLACEMENT_3D ( 'NONE', #2836, #1791, #8051 ) ;
#8834=ORIENTED_EDGE ( 'NONE', *, *, #5052, .T. ) ;
#8838=EDGE_CURVE ( 'NONE', #12848, #2425, #5831, .T. ) ;
#8839=CARTESIAN_POINT ( 'NONE',  ( -238.9707249590438494, 1.103996713823099496, 11.69802420356912087 ) ) ;
#8841=( GEOMETRIC_REPRESENTATION_CONTEXT ( 3 ) GLOBAL_UNCERTAINTY_ASSIGNED_CONTEXT ( ( #6923 ) ) GLOBAL_UNIT_ASSIGNED_CONTEXT ( ( #2321, #333, #3377 ) ) REPRESENTATION_CONTEXT ( 'NONE', 'WORKASPACE' ) );
#8842=VECTOR ( 'NONE', #1099, 1000.000000000000000 ) ;
#8843=ADVANCED_FACE ( 'NONE', ( #5749 ), #11972, .F. ) ;
#8847=CARTESIAN_POINT ( 'NONE',  ( -229.7748312726236293, 5.886477795347762942, -10.17644301346884816 ) ) ;
#8850=CONICAL_SURFACE ( 'NONE', #10121, 6.500000000000005329, 0.7853981633974476129 ) ;
#8853=ORIENTED_EDGE ( 'NONE', *, *, #7767, .T. ) ;
#8855=EDGE_LOOP ( 'NONE', ( #5894, #9026, #6373, #11016 ) ) ;
#8858=CARTESIAN_POINT ( 'NONE',  ( -248.7692280202239772, -10.08940167826270340, -6.022204372421657403 ) ) ;
#8861=DIRECTION ( 'NONE',  ( 0.000000000000000000, 1.000000000000000000, 0.000000000000000000 ) ) ;
#8862=CARTESIAN_POINT ( 'NONE',  ( -122.2593324768321992, 19.00000000000000000, 168.2755348299905052 ) ) ;
#8863=DIRECTION ( 'NONE',  ( 0.000000000000000000, -1.000000000000000000, 0.000000000000000000 ) ) ;
#8864=DIRECTION ( 'NONE',  ( 0.000000000000000000, -1.000000000000000000, 0.000000000000000000 ) ) ;
#8867=CARTESIAN_POINT ( 'NONE',  ( 229.9902049636500863, 2.785755589373224428, 2.131144504211401891 ) ) ;
#8868=CARTESIAN_POINT ( 'NONE',  ( -249.7994463212561982, 11.74985191749823699, 0.3872576247023094553 ) ) ;
#8875=CONICAL_SURFACE ( 'NONE', #7600, 5.499999999999998224, 0.7853981633974461696 ) ;
#8879=CARTESIAN_POINT ( 'NONE',  ( 71.82423009839129691, 30.00000000000000000, 197.3354503650404865 ) ) ;
#8880=CARTESIAN_POINT ( 'NONE',  ( 240.3371538976029456, 2.621326596184952340, -2.332469087881691383 ) ) ;
#8882=EDGE_CURVE ( 'NONE', #7690, #10052, #2178, .T. ) ;
#8885=EDGE_LOOP ( 'NONE', ( #6716, #2791, #4467, #11855 ) ) ;
#8886=ORIENTED_EDGE ( 'NONE', *, *, #2074, .F. ) ;
#8887=PRODUCT_DEFINITION_CONTEXT ( 'detailed design', #3002, 'design' ) ;
#8889=EDGE_LOOP ( 'NONE', ( #1204, #5974, #10971, #9933 ) ) ;
#8894=EDGE_CURVE ( 'NONE', #5845, #10191, #3876, .T. ) ;
#8897=DIRECTION ( 'NONE',  ( 8.659560562354693735E-17, 0.7071067811865670016, -0.7071067811865280328 ) ) ;
#8902=CARTESIAN_POINT ( 'NONE',  ( 0.000000000000000000, 21.50000000000000000, 0.000000000000000000 ) ) ;
#8903=ORIENTED_EDGE ( 'NONE', *, *, #2512, .T. ) ;
#8904=CARTESIAN_POINT ( 'NONE',  ( 3.034674768287141263E-14, -11.79660968244690089, -247.7999999999999829 ) ) ;
#8907=CIRCLE ( 'NONE', #4220, 5.500000000000005329 ) ;
#8908=CIRCLE ( 'NONE', #4221, 196.0000000000000000 ) ;
#8910=AXIS2_PLACEMENT_3D ( 'NONE', #9671, #10805, #6689 ) ;
#8912=CONICAL_SURFACE ( 'NONE', #2716, 249.7999999999999829, 0.7853981633974066456 ) ;
#8914=EDGE_CURVE ( 'NONE', #12886, #11448, #11122, .T. ) ;
#8916=AXIS2_PLACEMENT_3D ( 'NONE', #9419, #7285, #6292 ) ;
#8919=ORIENTED_EDGE ( 'NONE', *, *, #1899, .T. ) ;
#8920=CARTESIAN_POINT ( 'NONE',  ( -238.9571479262659750, -1.076402584257635686, -11.70061130326932464 ) ) ;
#8925=CARTESIAN_POINT ( 'NONE',  ( -249.7762712555648932, -11.55521436350650255, -2.133810497648569893 ) ) ;
#8937=FACE_OUTER_BOUND ( 'NONE', #8306, .T. ) ;
#8939=CARTESIAN_POINT ( 'NONE',  ( -229.8892649129228971, -9.344369417327452965, 7.164599271245471357 ) ) ;
#8942=CARTESIAN_POINT ( 'NONE',  ( -249.7841416269946535, 11.60584252726589938, 1.834925605678527027 ) ) ;
#8948=CARTESIAN_POINT ( 'NONE',  ( 197.8197553893920144, 19.00000000000000000, 69.77553482998851564 ) ) ;
#8950=LINE ( 'NONE', #9015, #3463 ) ;
#8952=CARTESIAN_POINT ( 'NONE',  ( -245.3311829420961487, -8.905423748641078774, 7.665289358291517807 ) ) ;
#8953=ORIENTED_EDGE ( 'NONE', *, *, #3863, .T. ) ;
#8957=ORIENTED_EDGE ( 'NONE', *, *, #10605, .T. ) ;
#8960=EDGE_LOOP ( 'NONE', ( #6705, #11068, #9025, #382 ) ) ;
#8962=DIRECTION ( 'NONE',  ( 0.000000000000000000, 0.000000000000000000, 1.000000000000000000 ) ) ;
#8965=CARTESIAN_POINT ( 'NONE',  ( -243.1520458356093286, -7.443371746667396316, 9.091683909978234723 ) ) ;
#8968=ORIENTED_EDGE ( 'NONE', *, *, #11588, .F. ) ;
#8970=ORIENTED_EDGE ( 'NONE', *, *, #8210, .T. ) ;
#8971=CARTESIAN_POINT ( 'NONE',  ( -246.6693634553872982, 9.463199073315145426, -6.964939579051701024 ) ) ;
#8976=DIRECTION ( 'NONE',  ( 0.000000000000000000, -1.000000000000000000, 0.000000000000000000 ) ) ;
#8978=EDGE_CURVE ( 'NONE', #10501, #9249, #5548, .T. ) ;
#8979=CARTESIAN_POINT ( 'NONE',  ( -229.9257603561380847, 10.20286607437010495, -5.878144477166547865 ) ) ;
#8985=CARTESIAN_POINT ( 'NONE',  ( -239.5361044668159991, -1.848645179572815156, -11.60366368868215758 ) ) ;
#8988=ORIENTED_EDGE ( 'NONE', *, *, #1514, .T. ) ;
#8989=B_SPLINE_CURVE_WITH_KNOTS ( 'NONE', 3,
 ( #4496, #2686, #12641, #1578, #11646, #3501, #2500, #12701, #6583, #10638, #11714, #6646, #5640, #11096, #2819, #10970, #8034, #12165, #4959, #10032, #7480, #7036, #7102, #11026 ),
 .UNSPECIFIED., .F., .F.,
 ( 4, 2, 2, 1, 1, 2, 2, 2, 2, 1, 1, 2, 2, 4 ),
 ( 0.5000762939474624469, 0.6250572204606649196, 0.6875476837172660449, 0.7187929153455667741, 0.7344155311597135860, 0.7422268390667906557, 0.7500381469738676143, 0.8125286102304378755, 0.8437738418587181766, 0.8593964576728634341, 0.8672077655799359519, 0.8711134195334776509, 0.8750190734870191278, 1.000000000000000000 ),
 .UNSPECIFIED. ) ;
#8990=EDGE_CURVE ( 'NONE', #3329, #11853, #1549, .T. ) ;
#8991=CARTESIAN_POINT ( 'NONE',  ( -249.7843163504504389, -11.60707272974070214, -1.827122155921521607 ) ) ;
#8998=CARTESIAN_POINT ( 'NONE',  ( 0.000000000000000000, 0.000000000000000000, 0.000000000000000000 ) ) ;
#9002=CARTESIAN_POINT ( 'NONE',  ( -229.9414646403920699, -10.54384660290364728, 5.199876785550554992 ) ) ;
#9006=EDGE_CURVE ( 'NONE', #4577, #889, #1009, .T. ) ;
#9008=EDGE_LOOP ( 'NONE', ( #6044, #10703 ) ) ;
#9011=DIRECTION ( 'NONE',  ( 0.000000000000000000, 1.000000000000000000, 0.000000000000000000 ) ) ;
#9013=CARTESIAN_POINT ( 'NONE',  ( 0.000000000000000000, -11.79660968244690089, 0.000000000000000000 ) ) ;
#9015=CARTESIAN_POINT ( 'NONE',  ( 71.82423009839129691, 30.00000000000000000, -192.2354503650404922 ) ) ;
#9017=TOROIDAL_SURFACE ( 'NONE', #8177, 238.4705882352940307, 2.000000000000000000 ) ;
#9021=ORIENTED_EDGE ( 'NONE', *, *, #10342, .F. ) ;
#9022=PLANE ( 'NONE',  #632 ) ;
#9025=ORIENTED_EDGE ( 'NONE', *, *, #135, .T. ) ;
#9026=ORIENTED_EDGE ( 'NONE', *, *, #1678, .T. ) ;
#9034=CARTESIAN_POINT ( 'NONE',  ( -242.2132964870923502, 6.511711374314640643, 9.780601349828243585 ) ) ;
#9035=ORIENTED_EDGE ( 'NONE', *, *, #117, .F. ) ;
#9037=ORIENTED_EDGE ( 'NONE', *, *, #763, .F. ) ;
#9042=CARTESIAN_POINT ( 'NONE',  ( 122.2593324768334071, 19.00000000000000000, -162.7755348299894820 ) ) ;
#9045=CARTESIAN_POINT ( 'NONE',  ( 71.82423009839129691, 19.40000000000000213, -192.2354503650404922 ) ) ;
#9054=EDGE_CURVE ( 'NONE', #6584, #9162, #8950, .T. ) ;
#9063=VECTOR ( 'NONE', #12434, 1000.000000000000114 ) ;
#9068=LINE ( 'NONE', #4925, #7763 ) ;
#9070=DIRECTION ( 'NONE',  ( 0.000000000000000000, 0.000000000000000000, -1.000000000000000000 ) ) ;
#9071=ORIENTED_EDGE ( 'NONE', *, *, #12357, .T. ) ;
#9072=EDGE_LOOP ( 'NONE', ( #10067, #1367, #9948, #6204 ) ) ;
#9074=DIRECTION ( 'NONE',  ( 0.000000000000000000, 0.000000000000000000, 1.000000000000000000 ) ) ;
#9076=ADVANCED_FACE ( 'NONE', ( #1818 ), #2820, .F. ) ;
#9077=DIRECTION ( 'NONE',  ( 0.000000000000000000, 0.000000000000000000, 1.000000000000000000 ) ) ;
#9085=CARTESIAN_POINT ( 'NONE',  ( 197.8197553893920144, 19.00000000000000000, 64.27553482998850143 ) ) ;
#9087=ORIENTED_EDGE ( 'NONE', *, *, #7292, .F. ) ;
#9088=ORIENTED_EDGE ( 'NONE', *, *, #2012, .T. ) ;
#9089=DIRECTION ( 'NONE',  ( 0.000000000000000000, 1.000000000000000000, 0.000000000000000000 ) ) ;
#9091=CARTESIAN_POINT ( 'NONE',  ( -249.6759349623767434, 11.17873215479417581, 3.619182054004953741 ) ) ;
#9093=ADVANCED_FACE ( 'NONE', ( #3941 ), #18, .F. ) ;
#9096=CARTESIAN_POINT ( 'NONE',  ( -243.2136795380932313, 7.496740017165948622, 9.047741631695624065 ) ) ;
#9099=ORIENTED_EDGE ( 'NONE', *, *, #5467, .F. ) ;
#9100=CARTESIAN_POINT ( 'NONE',  ( -245.3969493176502397, 8.938055201219498258, -7.627167029064186643 ) ) ;
#9103=CARTESIAN_POINT ( 'NONE',  ( 122.2593324768346008, 30.00000000000000000, 168.2755348299889988 ) ) ;
#9108=LINE ( 'NONE', #11110, #704 ) ;
#9115=CARTESIAN_POINT ( 'NONE',  ( -249.3105109839375189, -10.55009524026396228, 5.172972615363025106 ) ) ;
#9122=CARTESIAN_POINT ( 'NONE',  ( -244.4357566112991549, -8.400224617168833063, -8.216123742228331750 ) ) ;
#9123=EDGE_CURVE ( 'NONE', #9288, #5992, #9854, .T. ) ;
#9128=CARTESIAN_POINT ( 'NONE',  ( -229.8105890609549817, -7.167558729527323536, 9.342082834280224901 ) ) ;
#9132=AXIS2_PLACEMENT_3D ( 'NONE', #2739, #9089, #3420 ) ;
#9135=EDGE_LOOP ( 'NONE', ( #10210, #1297, #5430, #8128 ) ) ;
#9137=CARTESIAN_POINT ( 'NONE',  ( 197.8197553893920144, 30.00000000000000000, 57.77553482998850143 ) ) ;
#9140=DIRECTION ( 'NONE',  ( 0.000000000000000000, 0.000000000000000000, 1.000000000000000000 ) ) ;
#9142=AXIS2_PLACEMENT_3D ( 'NONE', #12080, #1823, #1015 ) ;
#9144=CARTESIAN_POINT ( 'NONE',  ( -241.5622318746700046, -5.708434620867652853, 10.27645530603111723 ) ) ;
#9149=CARTESIAN_POINT ( 'NONE',  ( 229.9733680233431130, -0.2284314955805349379, -3.499999999999966249 ) ) ;
#9154=EDGE_CURVE ( 'NONE', #12564, #8176, #4073, .T. ) ;
#9156=DIRECTION ( 'NONE',  ( 0.000000000000000000, 0.7071067811865480168, 0.7071067811865470176 ) ) ;
#9160=CARTESIAN_POINT ( 'NONE',  ( -245.0777337327412795, 8.776737542119800395, 7.814324100309848475 ) ) ;
#9162=VERTEX_POINT ( 'NONE', #1945 ) ;
#9170=PRODUCT_DEFINITION_FORMATION_WITH_SPECIFIED_SOURCE ( 'ANY', '', #334, .NOT_KNOWN. ) ;
#9171=DIRECTION ( 'NONE',  ( 0.000000000000000000, 1.000000000000000000, 0.000000000000000000 ) ) ;
#9173=CARTESIAN_POINT ( 'NONE',  ( 122.2593324768334071, 19.00000000000000000, -168.2755348299895104 ) ) ;
#9180=CARTESIAN_POINT ( 'NONE',  ( 0.000000000000000000, 29.00000000000000000, 0.000000000000000000 ) ) ;
#9185=CARTESIAN_POINT ( 'NONE',  ( -249.2062170167872068, 10.43176588139601257, -5.409795435560969423 ) ) ;
#9187=DIRECTION ( 'NONE',  ( 0.000000000000000000, -1.000000000000000000, 0.000000000000000000 ) ) ;
#9189=VECTOR ( 'NONE', #7041, 1000.000000000000000 ) ;
#9193=CARTESIAN_POINT ( 'NONE',  ( -243.2454781611184274, -7.524012747006318946, -9.025130280554842344 ) ) ;
#9198=LINE ( 'NONE', #12400, #7077 ) ;
#9199=ORIENTED_EDGE ( 'NONE', *, *, #6741, .T. ) ;
#9201=AXIS2_PLACEMENT_3D ( 'NONE', #4235, #1179, #8317 ) ;
#9205=VECTOR ( 'NONE', #149, 1000.000000000000000 ) ;
#9211=AXIS2_PLACEMENT_3D ( 'NONE', #5838, #10218, #897 ) ;
#9212=CARTESIAN_POINT ( 'NONE',  ( -243.1473425731909117, -7.439266815360506158, 9.095043743685003790 ) ) ;
#9215=CARTESIAN_POINT ( 'NONE',  ( 71.82423009839129691, 28.60000000000000142, -197.3354503650404865 ) ) ;
#9220=EDGE_CURVE ( 'NONE', #8160, #6601, #6670, .T. ) ;
#9229=CIRCLE ( 'NONE', #508, 239.0000000000000000 ) ;
#9231=CARTESIAN_POINT ( 'NONE',  ( -245.5121636011789690, 8.994012744481606703, 7.561165849620649304 ) ) ;
#9232=ADVANCED_FACE ( 'NONE', ( #6285 ), #10539, .F. ) ;
#9236=ORIENTED_EDGE ( 'NONE', *, *, #10581, .T. ) ;
#9238=EDGE_LOOP ( 'NONE', ( #10005, #3168 ) ) ;
#9241=CARTESIAN_POINT ( 'NONE',  ( 239.1910253111598479, 1.013189013438377417, 3.350157823592870177 ) ) ;
#9249=VERTEX_POINT ( 'NONE', #10335 ) ;
#9250=VECTOR ( 'NONE', #10840, 1000.000000000000000 ) ;
#9251=DIRECTION ( 'NONE',  ( 0.000000000000000000, 0.000000000000000000, -1.000000000000000000 ) ) ;
#9252=ORIENTED_EDGE ( 'NONE', *, *, #12273, .T. ) ;
#9253=DIRECTION ( 'NONE',  ( 0.000000000000000000, 1.000000000000000000, 0.000000000000000000 ) ) ;
#9255=VECTOR ( 'NONE', #771, 1000.000000000000000 ) ;
#9257=CARTESIAN_POINT ( 'NONE',  ( -249.2062170165277166, -10.43176588117700021, 5.409795435997606816 ) ) ;
#9258=ORIENTED_EDGE ( 'NONE', *, *, #1419, .T. ) ;
#9263=CARTESIAN_POINT ( 'NONE',  ( -243.4706526255369283, -7.711678295906986058, -8.866250711340882162 ) ) ;
#9264=VECTOR ( 'NONE', #1746, 1000.000000000000000 ) ;
#9269=CARTESIAN_POINT ( 'NONE',  ( 122.2593324768346008, 30.00000000000000000, 168.2755348299889988 ) ) ;
#9272=COLOUR_RGB ( '', 0.08235294, 0.09019608, 0.10196078) ;
#9274=DIRECTION ( 'NONE',  ( 0.000000000000000000, -1.000000000000000000, 0.000000000000000000 ) ) ;
#9275=AXIS2_PLACEMENT_3D ( 'NONE', #12369, #5157, #8309 ) ;
#9278=LINE ( 'NONE', #11723, #9205 ) ;
#9279=DIRECTION ( 'NONE',  ( 0.000000000000000000, 0.000000000000000000, -1.000000000000000000 ) ) ;
#9282=AXIS2_PLACEMENT_3D ( 'NONE', #11597, #8716, #12651 ) ;
#9283=ORIENTED_EDGE ( 'NONE', *, *, #9825, .F. ) ;
#9284=CARTESIAN_POINT ( 'NONE',  ( 240.3826708216964789, -2.772967769359314882, -2.135567781667015108 ) ) ;
#9285=CIRCLE ( 'NONE', #10985, 6.500000000000005329 ) ;
#9286=CARTESIAN_POINT ( 'NONE',  ( 229.9983178831911630, -3.387952982252648404, -0.9078284637049901518 ) ) ;
#9288=VERTEX_POINT ( 'NONE', #2139 ) ;
#9289=CARTESIAN_POINT ( 'NONE',  ( 240.3371538976037982, -2.621326596188751079, 2.332469087876801517 ) ) ;
#9292=DIRECTION ( 'NONE',  ( 0.000000000000000000, 0.000000000000000000, -1.000000000000000000 ) ) ;
#9294=CARTESIAN_POINT ( 'NONE',  ( -245.4374131353386304, 8.957880035620332748, 7.603877364227019875 ) ) ;
#9295=ADVANCED_FACE ( 'NONE', ( #11412 ), #12833, .F. ) ;
#9296=ADVANCED_FACE ( 'NONE', ( #408 ), #3888, .F. ) ;
#9300=DIRECTION ( 'NONE',  ( 0.000000000000000000, 0.000000000000000000, 1.000000000000000000 ) ) ;
#9301=ORIENTED_EDGE ( 'NONE', *, *, #2955, .F. ) ;
#9302=ORIENTED_EDGE ( 'NONE', *, *, #11298, .F. ) ;
#9304=CARTESIAN_POINT ( 'NONE',  ( 0.000000000000000000, -20.00000000000000000, 248.7999999999999829 ) ) ;
#9314=ORIENTED_EDGE ( 'NONE', *, *, #9890, .F. ) ;
#9315=LINE ( 'NONE', #4244, #7632 ) ;
#9316=CARTESIAN_POINT ( 'NONE',  ( -197.8197553893924976, 29.00000000000000000, -64.27553482998719403 ) ) ;
#9317=CARTESIAN_POINT ( 'NONE',  ( -248.8927262316770737, -10.16869272925975309, 5.887412070189221858 ) ) ;
#9321=ADVANCED_FACE ( 'NONE', ( #9344 ), #5592, .F. ) ;
#9323=CARTESIAN_POINT ( 'NONE',  ( 0.000000000000000000, 29.00000000000000000, -208.0000000000000000 ) ) ;
#9324=CARTESIAN_POINT ( 'NONE',  ( -247.3797639054675415, -9.674571922432775750, -6.668012154483388798 ) ) ;
#9335=ADVANCED_FACE ( 'NONE', ( #1145 ), #11474, .T. ) ;
#9338=CARTESIAN_POINT ( 'NONE',  ( 197.8197553893920144, 30.00000000000000000, 70.77553482998851564 ) ) ;
#9339=DIRECTION ( 'NONE',  ( 0.000000000000000000, -1.000000000000000000, 0.000000000000000000 ) ) ;
#9340=AXIS2_PLACEMENT_3D ( 'NONE', #1626, #9745, #3889 ) ;
#9342=EDGE_CURVE ( 'NONE', #11150, #9966, #12204, .T. ) ;
#9344=FACE_OUTER_BOUND ( 'NONE', #7849, .T. ) ;
#9347=CARTESIAN_POINT ( 'NONE',  ( -246.6527294680201408, -9.457576189692451507, 6.972573804907313821 ) ) ;
#9352=CARTESIAN_POINT ( 'NONE',  ( 0.000000000000000000, 1.438959988998140160E-15, 11.75000000000000000 ) ) ;
#9357=CARTESIAN_POINT ( 'NONE',  ( 3.061616997868383121E-14, 0.000000000000000000, 250.0000000000000000 ) ) ;
#9358=CIRCLE ( 'NONE', #7015, 249.7999999999999829 ) ;
#9360=CYLINDRICAL_SURFACE ( 'NONE', #3235, 5.500000000000005329 ) ;
#9362=CARTESIAN_POINT ( 'NONE',  ( -240.2602214610376450, 3.236828995589876357, 11.30545424820408229 ) ) ;
#9364=ORIENTED_EDGE ( 'NONE', *, *, #8821, .F. ) ;
#9369=EDGE_LOOP ( 'NONE', ( #2550, #1545, #9416, #3963 ) ) ;
#9370=EDGE_CURVE ( 'NONE', #808, #11582, #5602, .T. ) ;
#9372=CARTESIAN_POINT ( 'NONE',  ( 0.000000000000000000, 19.00000000000000000, -208.0000000000000000 ) ) ;
#9376=CARTESIAN_POINT ( 'NONE',  ( 0.000000000000000000, -19.00000000000000000, -230.0000000000000000 ) ) ;
#9378=DIRECTION ( 'NONE',  ( 0.000000000000000000, 0.000000000000000000, 1.000000000000000000 ) ) ;
#9380=ORIENTED_EDGE ( 'NONE', *, *, #375, .F. ) ;
#9384=DIRECTION ( 'NONE',  ( 0.000000000000000000, 0.000000000000000000, 1.000000000000000000 ) ) ;
#9390=CARTESIAN_POINT ( 'NONE',  ( 0.000000000000000000, 30.00000000000000000, -208.0000000000000000 ) ) ;
#9392=CARTESIAN_POINT ( 'NONE',  ( -242.8048495217675509, -7.129644031679399419, -9.341687344795504444 ) ) ;
#9394=CARTESIAN_POINT ( 'NONE',  ( 239.0427084576793959, -0.5779638303088237006, 3.452011086608069323 ) ) ;
#9397=CONICAL_SURFACE ( 'NONE', #5781, 230.0000000000000000, 0.7853981633974476129 ) ;
#9400=VECTOR ( 'NONE', #8042, 1000.000000000000000 ) ;
#9403=DIRECTION ( 'NONE',  ( 0.000000000000000000, -1.000000000000000000, 0.000000000000000000 ) ) ;
#9406=CARTESIAN_POINT ( 'NONE',  ( -248.6772030003816667, 10.03733143285744767, 6.108624101570837794 ) ) ;
#9407=CARTESIAN_POINT ( 'NONE',  ( 239.4470891770056653, -1.456698945183192651, -3.182458632634282303 ) ) ;
#9409=DIRECTION ( 'NONE',  ( 0.000000000000000000, 1.000000000000000000, 0.000000000000000000 ) ) ;
#9412=EDGE_CURVE ( 'NONE', #5790, #10498, #4589, .T. ) ;
#9413=CARTESIAN_POINT ( 'NONE',  ( 0.000000000000000000, 3.327561323230765034, 0.000000000000000000 ) ) ;
#9415=ADVANCED_FACE ( 'NONE', ( #5667 ), #7943, .F. ) ;
#9416=ORIENTED_EDGE ( 'NONE', *, *, #201, .T. ) ;
#9418=CARTESIAN_POINT ( 'NONE',  ( 0.000000000000000000, 30.00000000000000000, 208.0000000000000000 ) ) ;
#9419=CARTESIAN_POINT ( 'NONE',  ( 122.2593324768346008, 29.00000000000000000, 168.2755348299889988 ) ) ;
#9426=AXIS2_PLACEMENT_3D ( 'NONE', #12809, #4670, #1485 ) ;
#9432=EDGE_LOOP ( 'NONE', ( #961, #11839, #11989, #773 ) ) ;
#9439=AXIS2_PLACEMENT_3D ( 'NONE', #9503, #6576, #10636 ) ;
#9440=CARTESIAN_POINT ( 'NONE',  ( 122.2593324768346008, 19.00000000000000000, 162.7755348299889988 ) ) ;
#9441=FACE_OUTER_BOUND ( 'NONE', #6735, .T. ) ;
#9444=CARTESIAN_POINT ( 'NONE',  ( -238.7110076764417670, 0.01030032076102859601, -11.74999636971691963 ) ) ;
#9450=CARTESIAN_POINT ( 'NONE',  ( 0.000000000000000000, -19.00000000000000000, -230.0000000000000000 ) ) ;
#9456=DIRECTION ( 'NONE',  ( 0.000000000000000000, -1.000000000000000000, 0.000000000000000000 ) ) ;
#9460=CARTESIAN_POINT ( 'NONE',  ( -229.6996680450366171, 1.438960022146944131E-15, 11.75000000000000000 ) ) ;
#9461=SURFACE_STYLE_USAGE ( .BOTH. , #12460 ) ;
#9463=ADVANCED_FACE ( 'NONE', ( #5732 ), #2532, .T. ) ;
#9465=EDGE_CURVE ( 'NONE', #6828, #3384, #11864, .T. ) ;
#9469=DIRECTION ( 'NONE',  ( 0.000000000000000000, 1.000000000000000000, 0.000000000000000000 ) ) ;
#9474=DIRECTION ( 'NONE',  ( 0.000000000000000000, -1.000000000000000000, 0.000000000000000000 ) ) ;
#9476=DIRECTION ( 'NONE',  ( 8.659560562354913137E-17, -0.7071067811865489050, 0.7071067811865460184 ) ) ;
#9477=STYLED_ITEM ( 'NONE', ( #3313 ), #5959 ) ;
#9481=ORIENTED_EDGE ( 'NONE', *, *, #12395, .F. ) ;
#9484=CARTESIAN_POINT ( 'NONE',  ( 197.8197553893915028, 19.00000000000000000, -58.77553482998990830 ) ) ;
#9485=EDGE_CURVE ( 'NONE', #7994, #11942, #10794, .T. ) ;
#9489=DIRECTION ( 'NONE',  ( 0.000000000000000000, -1.000000000000000000, 0.000000000000000000 ) ) ;
#9491=LINE ( 'NONE', #10494, #3689 ) ;
#9492=DIRECTION ( 'NONE',  ( 8.659560562354963673E-17, 0.7071067811865450192, -0.7071067811865500152 ) ) ;
#9493=EDGE_LOOP ( 'NONE', ( #11667, #2737, #8171, #2032 ) ) ;
#9494=DIRECTION ( 'NONE',  ( 1.000000000000000000, 0.000000000000000000, 0.000000000000000000 ) ) ;
#9495=VERTEX_POINT ( 'NONE', #476 ) ;
#9500=CARTESIAN_POINT ( 'NONE',  ( 0.000000000000000000, 19.00000000000000000, -195.0000000000000000 ) ) ;
#9501=CARTESIAN_POINT ( 'NONE',  ( 239.1299809604698794, 0.8683754746916950706, -3.391597751417305240 ) ) ;
#9502=CARTESIAN_POINT ( 'NONE',  ( -238.9888240692591239, 1.140781236982990166, -11.69457573833076758 ) ) ;
#9503=CARTESIAN_POINT ( 'NONE',  ( 71.82423009839129691, 30.00000000000000000, 197.3354503650404865 ) ) ;
#9517=CARTESIAN_POINT ( 'NONE',  ( 122.2593324768334071, 30.00000000000000000, -168.2755348299895104 ) ) ;
#9521=AXIS2_PLACEMENT_3D ( 'NONE', #3906, #583, #11978 ) ;
#9523=DIRECTION ( 'NONE',  ( 0.000000000000000000, 1.000000000000000000, 0.000000000000000000 ) ) ;
#9526=CARTESIAN_POINT ( 'NONE',  ( 7.960204194457791533E-16, 18.00000000000000000, -201.4999999999999716 ) ) ;
#9530=CARTESIAN_POINT ( 'NONE',  ( -246.5915682055979801, -9.436693423004101078, 7.000847393551240749 ) ) ;
#9531=CARTESIAN_POINT ( 'NONE',  ( 240.5112511684797880, -3.170498834991128945, -1.486196988779163952 ) ) ;
#9535=DIRECTION ( 'NONE',  ( 0.000000000000000000, 0.000000000000000000, 1.000000000000000000 ) ) ;
#9537=AXIS2_PLACEMENT_3D ( 'NONE', #8743, #1940, #9874 ) ;
#9538=EDGE_CURVE ( 'NONE', #1045, #9651, #12794, .T. ) ;
#9547=EDGE_CURVE ( 'NONE', #6775, #8308, #1533, .T. ) ;
#9551=DIRECTION ( 'NONE',  ( 0.000000000000000000, 1.000000000000000000, 0.000000000000000000 ) ) ;
#9552=ORIENTED_EDGE ( 'NONE', *, *, #12657, .F. ) ;
#9554=CIRCLE ( 'NONE', #9132, 6.500000000000005329 ) ;
#9556=CARTESIAN_POINT ( 'NONE',  ( 197.8197553893920144, 29.00000000000000000, 64.27553482998850143 ) ) ;
#9558=DIRECTION ( 'NONE',  ( 0.000000000000000000, 1.000000000000000000, 0.000000000000000000 ) ) ;
#9559=CIRCLE ( 'NONE', #8079, 6.500000000000005329 ) ;
#9560=DIRECTION ( 'NONE',  ( 0.000000000000000000, 1.000000000000000000, 0.000000000000000000 ) ) ;
#9561=CARTESIAN_POINT ( 'NONE',  ( 3.056106087272219914E-14, 22.00000000000000000, 249.2999999999999829 ) ) ;
#9563=ORIENTED_EDGE ( 'NONE', *, *, #755, .T. ) ;
#9565=ADVANCED_FACE ( 'NONE', ( #3728 ), #7794, .F. ) ;
#9569=DIRECTION ( 'NONE',  ( 0.000000000000000000, 1.000000000000000000, 0.000000000000000000 ) ) ;
#9570=CARTESIAN_POINT ( 'NONE',  ( -210.0000000000000000, 30.00000000000000000, 0.000000000000000000 ) ) ;
#9573=ADVANCED_FACE ( 'NONE', ( #7173 ), #4934, .F. ) ;
#9577=CARTESIAN_POINT ( 'NONE',  ( -229.7832113950239545, 6.204037592689317648, 9.986088990952895372 ) ) ;
#9578=DIRECTION ( 'NONE',  ( 0.000000000000000000, -1.000000000000000000, 0.000000000000000000 ) ) ;
#9583=LINE ( 'NONE', #4514, #8505 ) ;
#9584=EDGE_LOOP ( 'NONE', ( #78, #5700, #6730, #1861 ) ) ;
#9586=LINE ( 'NONE', #8278, #11594 ) ;
#9587=CARTESIAN_POINT ( 'NONE',  ( -197.8197553893924976, 18.00000000000000000, -70.77553482998720824 ) ) ;
#9589=DIRECTION ( 'NONE',  ( 0.000000000000000000, -1.000000000000000000, 0.000000000000000000 ) ) ;
#9593=CARTESIAN_POINT ( 'NONE',  ( 229.9733680233431130, 4.286263893147487610E-16, -3.499999999999964917 ) ) ;
#9594=CARTESIAN_POINT ( 'NONE',  ( 0.000000000000000000, 11.79660968244690089, 249.7999999999999829 ) ) ;
#9595=EDGE_CURVE ( 'NONE', #2165, #5446, #2588, .T. ) ;
#9598=DIRECTION ( 'NONE',  ( 0.000000000000000000, 1.000000000000000000, 0.000000000000000000 ) ) ;
#9600=ORIENTED_EDGE ( 'NONE', *, *, #5789, .T. ) ;
#9602=DIRECTION ( 'NONE',  ( 0.000000000000000000, 0.000000000000000000, -1.000000000000000000 ) ) ;
#9610=VERTEX_POINT ( 'NONE', #8114 ) ;
#9614=VERTEX_POINT ( 'NONE', #2040 ) ;
#9617=ORIENTED_EDGE ( 'NONE', *, *, #6818, .F. ) ;
#9618=AXIS2_PLACEMENT_3D ( 'NONE', #610, #3535, #2537 ) ;
#9620=CARTESIAN_POINT ( 'NONE',  ( -239.9867712987582706, 2.433335514366328667, -11.49559079283426755 ) ) ;
#9621=CONICAL_SURFACE ( 'NONE', #11974, 6.500000000000005329, 0.7853981633974518317 ) ;
#9622=EDGE_CURVE ( 'NONE', #10706, #8254, #12392, .T. ) ;
#9624=CARTESIAN_POINT ( 'NONE',  ( 0.000000000000000000, -3.327561323230890267, 238.4705882352940307 ) ) ;
#9625=LINE ( 'NONE', #2563, #6245 ) ;
#9627=EDGE_LOOP ( 'NONE', ( #10307, #111, #9968, #766 ) ) ;
#9630=ORIENTED_EDGE ( 'NONE', *, *, #11829, .T. ) ;
#9633=DIRECTION ( 'NONE',  ( 0.000000000000000000, 1.000000000000000000, 0.000000000000000000 ) ) ;
#9637=VECTOR ( 'NONE', #11611, 1000.000000000000000 ) ;
#9639=AXIS2_PLACEMENT_3D ( 'NONE', #9556, #11435, #1498 ) ;
#9640=CARTESIAN_POINT ( 'NONE',  ( 71.82423009839129691, 30.00000000000000000, 203.8354503650404865 ) ) ;
#9645=AXIS2_PLACEMENT_3D ( 'NONE', #4665, #3804, #2794 ) ;
#9651=VERTEX_POINT ( 'NONE', #10233 ) ;
#9652=CARTESIAN_POINT ( 'NONE',  ( -122.2593324768359935, 30.00000000000000000, -168.2755348299880040 ) ) ;
#9655=CARTESIAN_POINT ( 'NONE',  ( -229.6996680450365034, 7.200459016985159977E-17, -11.75000000000000000 ) ) ;
#9658=EDGE_CURVE ( 'NONE', #368, #1401, #1326, .T. ) ;
#9661=CARTESIAN_POINT ( 'NONE',  ( 3.059167704270088292E-14, 0.000000000000000000, 249.7999999999999829 ) ) ;
#9666=CARTESIAN_POINT ( 'NONE',  ( -122.2593324768321992, 19.00000000000000000, 168.2755348299905052 ) ) ;
#9667=ORIENTED_EDGE ( 'NONE', *, *, #1901, .T. ) ;
#9671=CARTESIAN_POINT ( 'NONE',  ( 0.000000000000000000, -2.772967769359314882, 0.000000000000000000 ) ) ;
#9677=DIRECTION ( 'NONE',  ( 0.000000000000000000, 0.000000000000000000, 1.000000000000000000 ) ) ;
#9678=CONICAL_SURFACE ( 'NONE', #1391, 195.0000000000000000, 0.7853981633974476129 ) ;
#9679=ORIENTED_EDGE ( 'NONE', *, *, #11690, .F. ) ;
#9681=CARTESIAN_POINT ( 'NONE',  ( 71.82423009839129691, 30.00000000000000000, -190.8354503650404865 ) ) ;
#9682=EDGE_LOOP ( 'NONE', ( #10831, #8688, #1857, #3059 ) ) ;
#9684=ORIENTED_EDGE ( 'NONE', *, *, #2892, .F. ) ;
#9687=CARTESIAN_POINT ( 'NONE',  ( -239.9440496357930499, 2.353898415756322304, -11.51208791644674001 ) ) ;
#9688=ADVANCED_FACE ( 'NONE', ( #10105 ), #10478, .F. ) ;
#9689=EDGE_CURVE ( 'NONE', #6909, #12416, #2100, .T. ) ;
#9691=CARTESIAN_POINT ( 'NONE',  ( -197.8197553893924976, 30.00000000000000000, -64.27553482998719403 ) ) ;
#9692=VERTEX_POINT ( 'NONE', #4103 ) ;
#9693=DIRECTION ( 'NONE',  ( 0.000000000000000000, 0.000000000000000000, 1.000000000000000000 ) ) ;
#9695=CARTESIAN_POINT ( 'NONE',  ( -241.5622318768846810, 5.708434624212912922, -10.27645530435382426 ) ) ;
#9699=DIRECTION ( 'NONE',  ( 0.000000000000000000, 0.000000000000000000, -1.000000000000000000 ) ) ;
#9700=CARTESIAN_POINT ( 'NONE',  ( -229.7307169744397584, 3.794695336103924177, -11.12700569152495689 ) ) ;
#9706=ORIENTED_EDGE ( 'NONE', *, *, #870, .F. ) ;
#9709=EDGE_CURVE ( 'NONE', #1760, #2672, #12375, .T. ) ;
#9710=CARTESIAN_POINT ( 'NONE',  ( -249.1360723393657395, -10.36505329229039596, -5.534757211193051418 ) ) ;
#9713=CARTESIAN_POINT ( 'NONE',  ( 0.000000000000000000, 25.50000000000000000, 249.7999999999999545 ) ) ;
#9714=DIRECTION ( 'NONE',  ( 0.000000000000000000, 0.000000000000000000, 1.000000000000000000 ) ) ;
#9715=DIRECTION ( 'NONE',  ( 0.000000000000000000, 0.000000000000000000, -1.000000000000000000 ) ) ;
#9719=CARTESIAN_POINT ( 'NONE',  ( 229.9750438049949537, 0.9064452134480361911, -3.388396133414032896 ) ) ;
#9722=CARTESIAN_POINT ( 'NONE',  ( -249.7544427809737613, 11.44486579037191554, 2.664765662472057262 ) ) ;
#9727=ORIENTED_EDGE ( 'NONE', *, *, #10382, .F. ) ;
#9728=ORIENTED_EDGE ( 'NONE', *, *, #7056, .T. ) ;
#9734=DIRECTION ( 'NONE',  ( 0.000000000000000000, 1.000000000000000000, 0.000000000000000000 ) ) ;
#9736=CARTESIAN_POINT ( 'NONE',  ( 0.000000000000000000, -3.327561323230890267, 0.000000000000000000 ) ) ;
#9738=ORIENTED_EDGE ( 'NONE', *, *, #10196, .F. ) ;
#9739=CARTESIAN_POINT ( 'NONE',  ( -122.2593324768321992, 30.00000000000000000, 168.2755348299905052 ) ) ;
#9744=ORIENTED_EDGE ( 'NONE', *, *, #59, .F. ) ;
#9745=DIRECTION ( 'NONE',  ( 0.000000000000000000, 1.000000000000000000, 0.000000000000000000 ) ) ;
#9748=CARTESIAN_POINT ( 'NONE',  ( 122.2593324768334071, 29.00000000000000000, -168.2755348299895104 ) ) ;
#9750=( LENGTH_UNIT ( ) NAMED_UNIT ( * ) SI_UNIT ( .MILLI., .METRE. ) );
#9751=CARTESIAN_POINT ( 'NONE',  ( -248.0831933713610056, 9.830508068705238856, 6.436117704883899115 ) ) ;
#9758=DIRECTION ( 'NONE',  ( 0.000000000000000000, 1.000000000000000000, 0.000000000000000000 ) ) ;
#9760=ORIENTED_EDGE ( 'NONE', *, *, #790, .F. ) ;
#9761=CARTESIAN_POINT ( 'NONE',  ( -242.4218346718328974, 6.744440870307020219, -9.622654846098170012 ) ) ;
#9762=ORIENTED_EDGE ( 'NONE', *, *, #8649, .F. ) ;
#9763=CIRCLE ( 'NONE', #11046, 5.500000000000005329 ) ;
#9765=ADVANCED_FACE ( 'NONE', ( #12245 ), #3098, .F. ) ;
#9767=DIRECTION ( 'NONE',  ( 0.000000000000000000, 1.000000000000000000, 0.000000000000000000 ) ) ;
#9770=AXIS2_PLACEMENT_3D ( 'NONE', #9085, #7954, #10953 ) ;
#9774=EDGE_LOOP ( 'NONE', ( #8122, #7158 ) ) ;
#9776=AXIS2_PLACEMENT_3D ( 'NONE', #4265, #3124, #10394 ) ;
#9781=CARTESIAN_POINT ( 'NONE',  ( -248.7201528609607237, -10.06060527426557272, -6.070293049022396303 ) ) ;
#9787=AXIS2_PLACEMENT_3D ( 'NONE', #1802, #2909, #10060 ) ;
#9789=EDGE_CURVE ( 'NONE', #10014, #11582, #422, .T. ) ;
#9794=AXIS2_PLACEMENT_3D ( 'NONE', #6916, #4767, #6974 ) ;
#9795=CARTESIAN_POINT ( 'NONE',  ( -249.5826926912396573, 10.95569487812031184, -4.257357224325097000 ) ) ;
#9797=DIRECTION ( 'NONE',  ( 0.000000000000000000, 1.000000000000000000, 0.000000000000000000 ) ) ;
#9800=ORIENTED_EDGE ( 'NONE', *, *, #9154, .T. ) ;
#9801=CARTESIAN_POINT ( 'NONE',  ( -122.2593324768321992, 30.00000000000000000, 174.7755348299905052 ) ) ;
#9802=DIRECTION ( 'NONE',  ( 0.000000000000000000, 0.000000000000000000, -1.000000000000000000 ) ) ;
#9806=CARTESIAN_POINT ( 'NONE',  ( 71.82423009839129691, 19.40000000000000213, -202.4354503650404808 ) ) ;
#9809=CARTESIAN_POINT ( 'NONE',  ( 240.1760274753961824, 2.306688218039924188, -2.632364499241238054 ) ) ;
#9816=EDGE_LOOP ( 'NONE', ( #44, #12383, #1364, #733 ) ) ;
#9820=ORIENTED_EDGE ( 'NONE', *, *, #1992, .T. ) ;
#9825=EDGE_CURVE ( 'NONE', #12286, #6909, #473, .T. ) ;
#9826=LINE ( 'NONE', #5898, #7124 ) ;
#9832=CARTESIAN_POINT ( 'NONE',  ( -243.1949234309863641, 7.480730381643192928, -9.061063658798671483 ) ) ;
#9833=VERTEX_POINT ( 'NONE', #4423 ) ;
#9834=AXIS2_PLACEMENT_3D ( 'NONE', #9173, #3029, #3969 ) ;
#9835=AXIS2_PLACEMENT_3D ( 'NONE', #5101, #5034, #11235 ) ;
#9840=CARTESIAN_POINT ( 'NONE',  ( -229.9694381604553541, 11.13630876764823263, -3.767427992309325457 ) ) ;
#9847=ORIENTED_EDGE ( 'NONE', *, *, #1571, .F. ) ;
#9849=DIRECTION ( 'NONE',  ( 0.000000000000000000, 0.000000000000000000, -1.000000000000000000 ) ) ;
#9850=ORIENTED_EDGE ( 'NONE', *, *, #12261, .T. ) ;
#9852=CARTESIAN_POINT ( 'NONE',  ( -249.5485775756386033, -10.89766932192311621, -4.396091616435120919 ) ) ;
#9854=CIRCLE ( 'NONE', #10921, 5.100000000000000533 ) ;
#9856=DIRECTION ( 'NONE',  ( 0.000000000000000000, 0.000000000000000000, 1.000000000000000000 ) ) ;
#9859=CONICAL_SURFACE ( 'NONE', #5823, 5.500000000000005329, 0.7853981633974461696 ) ;
#9863=EDGE_CURVE ( 'NONE', #5331, #1614, #7714, .T. ) ;
#9867=CARTESIAN_POINT ( 'NONE',  ( 229.9999970288534712, 3.499804753153490378, -0.2337124727541820546 ) ) ;
#9869=CARTESIAN_POINT ( 'NONE',  ( -249.7048772684788105, 11.25744417597311475, 3.375279421353320597 ) ) ;
#9870=DIRECTION ( 'NONE',  ( 0.000000000000000000, 0.000000000000000000, 1.000000000000000000 ) ) ;
#9871=FACE_OUTER_BOUND ( 'NONE', #8807, .T. ) ;
#9874=DIRECTION ( 'NONE',  ( 0.000000000000000000, 0.000000000000000000, 1.000000000000000000 ) ) ;
#9877=CIRCLE ( 'NONE', #5848, 6.500000000000000000 ) ;
#9878=AXIS2_PLACEMENT_3D ( 'NONE', #10329, #1206, #3455 ) ;
#9880=DIRECTION ( 'NONE',  ( 0.000000000000000000, 0.000000000000000000, 1.000000000000000000 ) ) ;
#9882=DIRECTION ( 'NONE',  ( 0.000000000000000000, 1.000000000000000000, 0.000000000000000000 ) ) ;
#9883=DIRECTION ( 'NONE',  ( 0.000000000000000000, 1.000000000000000000, 0.000000000000000000 ) ) ;
#9887=VERTEX_POINT ( 'NONE', #10568 ) ;
#9888=EDGE_LOOP ( 'NONE', ( #8632, #9071, #4050, #625 ) ) ;
#9890=EDGE_CURVE ( 'NONE', #7200, #4744, #5498, .T. ) ;
#9897=FACE_OUTER_BOUND ( 'NONE', #8758, .T. ) ;
#9898=ORIENTED_EDGE ( 'NONE', *, *, #8914, .F. ) ;
#9899=DIRECTION ( 'NONE',  ( 8.659560562354913137E-17, -0.7071067811865489050, 0.7071067811865460184 ) ) ;
#9901=CARTESIAN_POINT ( 'NONE',  ( -248.0831933713610056, 9.830508068705238856, -6.436117704883929314 ) ) ;
#9903=TOROIDAL_SURFACE ( 'NONE', #3934, 247.7999999999999829, 2.000000000000000000 ) ;
#9907=CARTESIAN_POINT ( 'NONE',  ( 240.2816503055764485, 2.505215826442440896, 2.444791323487650825 ) ) ;
#9908=CARTESIAN_POINT ( 'NONE',  ( -197.8197553893909912, 19.00000000000000000, 64.27553482999130097 ) ) ;
#9909=CARTESIAN_POINT ( 'NONE',  ( -229.6996680450365034, 7.200459016985159977E-17, -11.75000000000000000 ) ) ;
#9910=EDGE_CURVE ( 'NONE', #7179, #1904, #8382, .T. ) ;
#9916=ORIENTED_EDGE ( 'NONE', *, *, #1165, .F. ) ;
#9917=CARTESIAN_POINT ( 'NONE',  ( -238.7452658386391420, -0.4192328095118098008, -11.74262570625762692 ) ) ;
#9918=AXIS2_PLACEMENT_3D ( 'NONE', #6080, #10009, #8075 ) ;
#9919=ORIENTED_EDGE ( 'NONE', *, *, #1708, .F. ) ;
#9920=ORIENTED_EDGE ( 'NONE', *, *, #1742, .F. ) ;
#9922=ORIENTED_EDGE ( 'NONE', *, *, #218, .F. ) ;
#9930=CARTESIAN_POINT ( 'NONE',  ( -249.7634162175664301, 11.48172780046974850, -2.515098136597289979 ) ) ;
#9933=ORIENTED_EDGE ( 'NONE', *, *, #4675, .T. ) ;
#9937=CIRCLE ( 'NONE', #4191, 10.00000000000000888 ) ;
#9939=DIRECTION ( 'NONE',  ( 0.000000000000000000, 1.000000000000000000, 0.000000000000000000 ) ) ;
#9941=CARTESIAN_POINT ( 'NONE',  ( 240.0429366796199702, 2.111384149270551625, -2.791848677271159485 ) ) ;
#9942=CONICAL_SURFACE ( 'NONE', #8256, 5.499999999999998224, 0.7853981633974461696 ) ;
#9943=B_SPLINE_CURVE_WITH_KNOTS ( 'NONE', 3,
 ( #10209, #8358, #11149, #2145, #6223, #11417, #1016, #1152, #3270, #5142, #6092, #7087, #5212, #2020, #7352, #10410, #5071, #1286, #2274, #9286, #11350, #156, #4079, #8422, #2215, #12354, #4209, #1217, #6352, #8293, #5349, #10343, #9149, #3205 ),
 .UNSPECIFIED., .F., .F.,
 ( 4, 2, 2, 2, 2, 2, 2, 2, 2, 2, 2, 2, 2, 2, 2, 2, 4 ),
 ( 8.253566423007127763E-20, 0.0006839223821429840340, 0.001367844764285967851, 0.002051767146428951343, 0.002735689528571936136, 0.003419611910714920929, 0.004103534292857904421, 0.004787456675000889214, 0.005471379057143873140, 0.006155301439286857933, 0.006839223821429841858, 0.007523146203572825784, 0.008207068585715808842, 0.008890990967858792768, 0.009574913350001776693, 0.01025883573214476062, 0.01094275811428774454 ),
 .UNSPECIFIED. ) ;
#9946=CARTESIAN_POINT ( 'NONE',  ( 3.059167704270088292E-14, 0.000000000000000000, 249.7999999999999829 ) ) ;
#9948=ORIENTED_EDGE ( 'NONE', *, *, #5467, .T. ) ;
#9949=ADVANCED_FACE ( 'NONE', ( #2814 ), #2598, .T. ) ;
#9951=DIRECTION ( 'NONE',  ( 0.000000000000000000, 0.000000000000000000, 1.000000000000000000 ) ) ;
#9962=EDGE_CURVE ( 'NONE', #6293, #1635, #12406, .T. ) ;
#9966=VERTEX_POINT ( 'NONE', #6772 ) ;
#9967=DIRECTION ( 'NONE',  ( 0.000000000000000000, -1.000000000000000000, 0.000000000000000000 ) ) ;
#9968=ORIENTED_EDGE ( 'NONE', *, *, #1420, .F. ) ;
#9969=DIRECTION ( 'NONE',  ( 0.000000000000000000, 0.000000000000000000, 1.000000000000000000 ) ) ;
#9973=VECTOR ( 'NONE', #10023, 1000.000000000000114 ) ;
#9974=AXIS2_PLACEMENT_3D ( 'NONE', #11488, #28, #2219 ) ;
#9975=CARTESIAN_POINT ( 'NONE',  ( -229.7432275410588716, 4.515244320528268851, -10.86800257939080971 ) ) ;
#9985=CARTESIAN_POINT ( 'NONE',  ( -239.0190678775036304, -1.196910341722188242, -11.68891451112129864 ) ) ;
#9987=EDGE_CURVE ( 'NONE', #1760, #5790, #8573, .T. ) ;
#9990=CARTESIAN_POINT ( 'NONE',  ( -249.7838850256695764, -11.60404975226508739, -1.846229155068394467 ) ) ;
#9993=EDGE_CURVE ( 'NONE', #5790, #1760, #4407, .T. ) ;
#9996=CARTESIAN_POINT ( 'NONE',  ( -247.9656915563521977, -9.808762669708828597, -6.469331566110803955 ) ) ;
#10001=CARTESIAN_POINT ( 'NONE',  ( -229.9923139574567585, -11.59881862766272320, 1.917681925180096281 ) ) ;
#10005=ORIENTED_EDGE ( 'NONE', *, *, #8882, .T. ) ;
#10007=AXIS2_PLACEMENT_3D ( 'NONE', #10822, #12825, #11836 ) ;
#10009=DIRECTION ( 'NONE',  ( 0.000000000000000000, 1.000000000000000000, 0.000000000000000000 ) ) ;
#10011=DIRECTION ( 'NONE',  ( 0.000000000000000000, 0.000000000000000000, 1.000000000000000000 ) ) ;
#10013=CARTESIAN_POINT ( 'NONE',  ( -242.9139448622711654, -7.229284208925894184, 9.262738308019747180 ) ) ;
#10014=VERTEX_POINT ( 'NONE', #11141 ) ;
#10023=DIRECTION ( 'NONE',  ( 8.659560562354913137E-17, -0.7071067811865489050, 0.7071067811865460184 ) ) ;
#10028=CARTESIAN_POINT ( 'NONE',  ( 0.000000000000000000, 3.327561323230765034, 238.4705882352940307 ) ) ;
#10029=ADVANCED_FACE ( 'NONE', ( #1877 ), #948, .F. ) ;
#10032=CARTESIAN_POINT ( 'NONE',  ( -239.1821278489683209, -1.453791005755859400, 11.65971745006329385 ) ) ;
#10035=EDGE_LOOP ( 'NONE', ( #8241, #7510 ) ) ;
#10037=VECTOR ( 'NONE', #9899, 1000.000000000000114 ) ;
#10040=DIRECTION ( 'NONE',  ( 0.000000000000000000, 1.000000000000000000, 0.000000000000000000 ) ) ;
#10041=CARTESIAN_POINT ( 'NONE',  ( 238.9791647118827029, 0.1781744854528612421, 3.496576182270254574 ) ) ;
#10042=CARTESIAN_POINT ( 'NONE',  ( 122.2593324768346008, 30.00000000000000000, 168.2755348299889988 ) ) ;
#10046=VERTEX_POINT ( 'NONE', #6017 ) ;
#10050=VERTEX_POINT ( 'NONE', #2995 ) ;
#10051=DIRECTION ( 'NONE',  ( 0.000000000000000000, 0.000000000000000000, -1.000000000000000000 ) ) ;
#10052=VERTEX_POINT ( 'NONE', #7078 ) ;
#10053=ADVANCED_FACE ( 'NONE', ( #6084 ), #10134, .F. ) ;
#10057=CARTESIAN_POINT ( 'NONE',  ( 71.82423009839129691, 30.00000000000000000, -203.8354503650404865 ) ) ;
#10059=TOROIDAL_SURFACE ( 'NONE', #70, 250.0000000000000000, 10.00000000000000000 ) ;
#10060=DIRECTION ( 'NONE',  ( 0.000000000000000000, 0.000000000000000000, 1.000000000000000000 ) ) ;
#10065=CARTESIAN_POINT ( 'NONE',  ( -229.8697759883668539, -8.858708711567949479, 7.758056923234300406 ) ) ;
#10067=ORIENTED_EDGE ( 'NONE', *, *, #2878, .F. ) ;
#10068=VERTEX_POINT ( 'NONE', #5203 ) ;
#10071=CARTESIAN_POINT ( 'NONE',  ( 0.000000000000000000, 1.848645179567965036, 0.000000000000000000 ) ) ;
#10073=CIRCLE ( 'NONE', #293, 5.500000000000005329 ) ;
#10074=DIRECTION ( 'NONE',  ( 0.000000000000000000, -1.000000000000000000, 0.000000000000000000 ) ) ;
#10075=AXIS2_PLACEMENT_3D ( 'NONE', #1442, #9758, #573 ) ;
#10079=CARTESIAN_POINT ( 'NONE',  ( -243.9217790761123581, -8.053804826441991693, 8.555499786857474476 ) ) ;
#10084=DIRECTION ( 'NONE',  ( 0.000000000000000000, 0.000000000000000000, 1.000000000000000000 ) ) ;
#10085=EDGE_LOOP ( 'NONE', ( #10755, #7007 ) ) ;
#10089=CARTESIAN_POINT ( 'NONE',  ( -248.3468897629254286, 9.892776367310945673, 6.340645126600181314 ) ) ;
#10092=CARTESIAN_POINT ( 'NONE',  ( -242.3262939448890450, 6.637532586066957840, 9.695808799222838559 ) ) ;
#10095=ORIENTED_EDGE ( 'NONE', *, *, #12961, .T. ) ;
#10096=CARTESIAN_POINT ( 'NONE',  ( -239.0839813628342370, 1.310043309152621571, 11.67696021899406134 ) ) ;
#10105=FACE_OUTER_BOUND ( 'NONE', #12851, .T. ) ;
#10107=FACE_OUTER_BOUND ( 'NONE', #5249, .T. ) ;
#10109=ORIENTED_EDGE ( 'NONE', *, *, #5154, .F. ) ;
#10110=CARTESIAN_POINT ( 'NONE',  ( -238.7109915777814138, -2.671037648644427152E-08, -11.74999999995326050 ) ) ;
#10112=ORIENTED_EDGE ( 'NONE', *, *, #4901, .T. ) ;
#10114=CARTESIAN_POINT ( 'NONE',  ( -249.7006323030246051, -11.24927497773904861, 3.394647654957348326 ) ) ;
#10115=ORIENTED_EDGE ( 'NONE', *, *, #2273, .F. ) ;
#10116=EDGE_CURVE ( 'NONE', #3851, #167, #9278, .T. ) ;
#10119=CARTESIAN_POINT ( 'NONE',  ( -240.0143494547118337, 2.418590315959113113, 11.50416929268522281 ) ) ;
#10120=CARTESIAN_POINT ( 'NONE',  ( -246.6923348785073244, -9.470909649843260780, -6.954450552458404822 ) ) ;
#10121=AXIS2_PLACEMENT_3D ( 'NONE', #3612, #7618, #9677 ) ;
#10122=CONICAL_SURFACE ( 'NONE', #8218, 248.7999999999999829, 0.7853981633974348453 ) ;
#10125=EDGE_CURVE ( 'NONE', #497, #1017, #12777, .T. ) ;
#10128=CARTESIAN_POINT ( 'NONE',  ( 122.2593324768346008, 29.00000000000000000, 173.7755348299889988 ) ) ;
#10129=ORIENTED_EDGE ( 'NONE', *, *, #816, .T. ) ;
#10130=EDGE_LOOP ( 'NONE', ( #4545, #10625 ) ) ;
#10132=CARTESIAN_POINT ( 'NONE',  ( 0.000000000000000000, 29.00000000000000000, 0.000000000000000000 ) ) ;
#10134=CYLINDRICAL_SURFACE ( 'NONE', #6023, 5.500000000000005329 ) ;
#10139=EDGE_CURVE ( 'NONE', #5992, #11915, #8283, .T. ) ;
#10140=ORIENTED_EDGE ( 'NONE', *, *, #11632, .F. ) ;
#10141=FACE_BOUND ( 'NONE', #10085, .T. ) ;
#10143=ORIENTED_EDGE ( 'NONE', *, *, #5955, .F. ) ;
#10147=DIRECTION ( 'NONE',  ( 0.000000000000000000, 0.000000000000000000, 1.000000000000000000 ) ) ;
#10151=CARTESIAN_POINT ( 'NONE',  ( -244.2512373980594305, 8.280505324206091089, 8.336413190213974644 ) ) ;
#10152=ORIENTED_EDGE ( 'NONE', *, *, #9658, .F. ) ;
#10154=ORIENTED_EDGE ( 'NONE', *, *, #12911, .T. ) ;
#10155=DIRECTION ( 'NONE',  ( 0.000000000000000000, 0.000000000000000000, -1.000000000000000000 ) ) ;
#10156=VERTEX_POINT ( 'NONE', #12247 ) ;
#10157=CONICAL_SURFACE ( 'NONE', #11872, 5.500000000000005329, 0.7853981633974461696 ) ;
#10159=CARTESIAN_POINT ( 'NONE',  ( 0.000000000000000000, 30.00000000000000000, 213.5000000000000000 ) ) ;
#10164=DIRECTION ( 'NONE',  ( 0.000000000000000000, 0.000000000000000000, 1.000000000000000000 ) ) ;
#10167=CARTESIAN_POINT ( 'NONE',  ( -239.3871161074123961, -1.704640323733336738, -11.62580261113903468 ) ) ;
#10170=CARTESIAN_POINT ( 'NONE',  ( -249.3819455666839531, 10.64000139048411597, -4.985720160764467224 ) ) ;
#10172=CARTESIAN_POINT ( 'NONE',  ( -249.7928741341071088, -11.67611540586379526, 1.322401171455369173 ) ) ;
#10175=CONICAL_SURFACE ( 'NONE', #4428, 248.7999999999999829, 0.7853981633974348453 ) ;
#10180=CARTESIAN_POINT ( 'NONE',  ( -247.2571636909562756, -9.642662942724268049, -6.714255738455707778 ) ) ;
#10182=DIRECTION ( 'NONE',  ( 0.000000000000000000, 1.000000000000000000, 0.000000000000000000 ) ) ;
#10185=CARTESIAN_POINT ( 'NONE',  ( 0.000000000000000000, 29.00000000000000000, 195.0000000000000000 ) ) ;
#10191=VERTEX_POINT ( 'NONE', #7311 ) ;
#10192=ORIENTED_EDGE ( 'NONE', *, *, #4594, .T. ) ;
#10195=FACE_OUTER_BOUND ( 'NONE', #12318, .T. ) ;
#10196=EDGE_CURVE ( 'NONE', #10050, #612, #2180, .T. ) ;
#10198=CARTESIAN_POINT ( 'NONE',  ( 239.4581646394902918, -1.471889791916103807, -3.175461175216562459 ) ) ;
#10200=CARTESIAN_POINT ( 'NONE',  ( 0.000000000000000000, 11.79660968244690089, 0.000000000000000000 ) ) ;
#10204=CARTESIAN_POINT ( 'NONE',  ( -244.4597039952343493, -8.419215818243479532, 8.199143447567463383 ) ) ;
#10207=FACE_BOUND ( 'NONE', #11621, .T. ) ;
#10209=CARTESIAN_POINT ( 'NONE',  ( 229.9733680233429993, 8.492964294626340574E-17, 3.499999999999964917 ) ) ;
#10210=ORIENTED_EDGE ( 'NONE', *, *, #2012, .F. ) ;
#10211=ORIENTED_EDGE ( 'NONE', *, *, #1678, .F. ) ;
#10216=ADVANCED_FACE ( 'NONE', ( #12111 ), #9621, .F. ) ;
#10218=DIRECTION ( 'NONE',  ( 0.000000000000000000, 1.000000000000000000, 0.000000000000000000 ) ) ;
#10220=CARTESIAN_POINT ( 'NONE',  ( -241.3883989929918528, 5.445712471069635185, 10.41186067220156097 ) ) ;
#10221=EDGE_CURVE ( 'NONE', #9610, #4744, #1757, .T. ) ;
#10227=CARTESIAN_POINT ( 'NONE',  ( 0.000000000000000000, 1.848645179567965036, 0.000000000000000000 ) ) ;
#10228=ORIENTED_EDGE ( 'NONE', *, *, #1396, .F. ) ;
#10229=CARTESIAN_POINT ( 'NONE',  ( -210.0000000000000000, 30.00000000000000000, 5.100000000000000533 ) ) ;
#10230=CARTESIAN_POINT ( 'NONE',  ( 0.000000000000000000, 2.772967769359004908, 0.000000000000000000 ) ) ;
#10231=EDGE_CURVE ( 'NONE', #4889, #3488, #180, .T. ) ;
#10232=CARTESIAN_POINT ( 'NONE',  ( 238.9743710625075721, 0.08886714786327083726, 3.499996468585938381 ) ) ;
#10233=CARTESIAN_POINT ( 'NONE',  ( 71.82423009839129691, 28.60000000000000142, 192.2354503650404922 ) ) ;
#10235=DIRECTION ( 'NONE',  ( 0.000000000000000000, 1.000000000000000000, 0.000000000000000000 ) ) ;
#10242=DIRECTION ( 'NONE',  ( 0.000000000000000000, 0.000000000000000000, 1.000000000000000000 ) ) ;
#10250=CARTESIAN_POINT ( 'NONE',  ( -242.2664987713461926, -6.571392929281715922, -9.740637196460863123 ) ) ;
#10253=AXIS2_PLACEMENT_3D ( 'NONE', #6248, #11232, #12173 ) ;
#10254=CARTESIAN_POINT ( 'NONE',  ( 239.2626306338483460, -1.161280184411060956, 3.302084438360472607 ) ) ;
#10256=DIRECTION ( 'NONE',  ( 0.000000000000000000, 0.000000000000000000, 1.000000000000000000 ) ) ;
#10257=DIRECTION ( 'NONE',  ( 0.000000000000000000, 0.000000000000000000, 1.000000000000000000 ) ) ;
#10264=ADVANCED_FACE ( 'NONE', ( #10107 ), #10303, .F. ) ;
#10265=EDGE_CURVE ( 'NONE', #8360, #8155, #3880, .T. ) ;
#10266=CARTESIAN_POINT ( 'NONE',  ( 239.4538130491200150, -1.465952997496189347, -3.178207852357353591 ) ) ;
#10267=DIRECTION ( 'NONE',  ( 0.000000000000000000, 1.000000000000000000, 0.000000000000000000 ) ) ;
#10269=DIRECTION ( 'NONE',  ( 0.000000000000000000, -1.000000000000000000, 0.000000000000000000 ) ) ;
#10272=CARTESIAN_POINT ( 'NONE',  ( -241.3198063618514482, -5.342363202628128249, 10.46527477498059255 ) ) ;
#10273=EDGE_LOOP ( 'NONE', ( #12497, #7513, #5213, #7018 ) ) ;
#10276=FACE_OUTER_BOUND ( 'NONE', #9888, .T. ) ;
#10277=ORIENTED_EDGE ( 'NONE', *, *, #870, .T. ) ;
#10279=DIRECTION ( 'NONE',  ( 0.000000000000000000, 0.000000000000000000, -1.000000000000000000 ) ) ;
#10281=AXIS2_PLACEMENT_3D ( 'NONE', #10473, #1340, #5409 ) ;
#10282=AXIS2_PLACEMENT_3D ( 'NONE', #921, #4978, #10915 ) ;
#10283=CIRCLE ( 'NONE', #11359, 5.500000000000005329 ) ;
#10285=CYLINDRICAL_SURFACE ( 'NONE', #12613, 5.500000000000005329 ) ;
#10288=CARTESIAN_POINT ( 'NONE',  ( -241.2214908397801594, 5.194817167650287892, 10.54181336101382271 ) ) ;
#10289=ORIENTED_EDGE ( 'NONE', *, *, #1008, .F. ) ;
#10292=ORIENTED_EDGE ( 'NONE', *, *, #11212, .F. ) ;
#10294=FACE_OUTER_BOUND ( 'NONE', #5387, .T. ) ;
#10295=ORIENTED_EDGE ( 'NONE', *, *, #3107, .F. ) ;
#10298=DIRECTION ( 'NONE',  ( 0.000000000000000000, 0.000000000000000000, 1.000000000000000000 ) ) ;
#10299=CARTESIAN_POINT ( 'NONE',  ( 239.4470891770647825, 1.456698945264939260, 3.182458632605157600 ) ) ;
#10300=CARTESIAN_POINT ( 'NONE',  ( 71.82423009839129691, 30.00000000000000000, -197.3354503650404865 ) ) ;
#10301=AXIS2_PLACEMENT_3D ( 'NONE', #11233, #2101, #6979 ) ;
#10303=CYLINDRICAL_SURFACE ( 'NONE', #9835, 5.500000000000005329 ) ;
#10304=ORIENTED_EDGE ( 'NONE', *, *, #6213, .T. ) ;
#10307=ORIENTED_EDGE ( 'NONE', *, *, #10551, .F. ) ;
#10309=CARTESIAN_POINT ( 'NONE',  ( -197.8197553893924976, 18.00000000000000000, -64.27553482998719403 ) ) ;
#10310=CARTESIAN_POINT ( 'NONE',  ( 197.8197553893915028, 30.00000000000000000, -64.27553482998990830 ) ) ;
#10312=CARTESIAN_POINT ( 'NONE',  ( -249.7865125415112857, -11.62303781240828648, 1.723091335424036696 ) ) ;
#10314=EDGE_CURVE ( 'NONE', #11942, #9651, #1982, .T. ) ;
#10317=CARTESIAN_POINT ( 'NONE',  ( -240.1208361041844910, 2.772967769358974710, 11.41810622433049893 ) ) ;
#10318=CARTESIAN_POINT ( 'NONE',  ( -243.3200464599152042, -7.587187367930753545, -8.972284967273612466 ) ) ;
#10319=VECTOR ( 'NONE', #2921, 1000.000000000000000 ) ;
#10320=CARTESIAN_POINT ( 'NONE',  ( 239.1625895583289605, -0.9513411441973714799, 3.369326940719206576 ) ) ;
#10323=CARTESIAN_POINT ( 'NONE',  ( 240.6264023546065971, 3.484414313184070355, -0.3842028184769861743 ) ) ;
#10329=CARTESIAN_POINT ( 'NONE',  ( 197.8197553893915028, 18.00000000000000000, -64.27553482998990830 ) ) ;
#10331=CARTESIAN_POINT ( 'NONE',  ( -248.9866437200756764, 10.23506903978361038, 5.772678316702733348 ) ) ;
#10332=CARTESIAN_POINT ( 'NONE',  ( 239.1683641398495013, -0.9613626713077001451, -3.365491595546588055 ) ) ;
#10333=CARTESIAN_POINT ( 'NONE',  ( 197.8197553893915028, 19.00000000000000000, -64.27553482998990830 ) ) ;
#10335=CARTESIAN_POINT ( 'NONE',  ( 71.82423009839129691, 18.00000000000000000, -203.8354503650404581 ) ) ;
#10341=DIRECTION ( 'NONE',  ( 0.000000000000000000, 0.000000000000000000, 1.000000000000000000 ) ) ;
#10342=EDGE_CURVE ( 'NONE', #12286, #6697, #9108, .T. ) ;
#10343=CARTESIAN_POINT ( 'NONE',  ( 229.9737195918793873, -0.4604175462015974718, -3.477110600454007994 ) ) ;
#10345=ORIENTED_EDGE ( 'NONE', *, *, #6665, .F. ) ;
#10346=CARTESIAN_POINT ( 'NONE',  ( 240.3826708216974737, -2.772967769359219847, 2.135567781667135012 ) ) ;
#10347=DIRECTION ( 'NONE',  ( 0.000000000000000000, -1.000000000000000000, 0.000000000000000000 ) ) ;
#10349=DIRECTION ( 'NONE',  ( 0.000000000000000000, 1.000000000000000000, 0.000000000000000000 ) ) ;
#10351=LINE ( 'NONE', #4543, #7106 ) ;
#10356=EDGE_LOOP ( 'NONE', ( #9252, #8419 ) ) ;
#10357=CARTESIAN_POINT ( 'NONE',  ( 2.394184492333075617E-14, 19.00000000000000000, 195.0000000000000000 ) ) ;
#10358=EDGE_LOOP ( 'NONE', ( #12250, #11080, #11095, #924 ) ) ;
#10359=EDGE_LOOP ( 'NONE', ( #1950, #9563, #6187, #2229 ) ) ;
#10361=CARTESIAN_POINT ( 'NONE',  ( 6.735557395310442023E-16, 30.00000000000000000, -213.5000000000000000 ) ) ;
#10362=DIRECTION ( 'NONE',  ( 0.000000000000000000, 0.000000000000000000, -1.000000000000000000 ) ) ;
#10365=CARTESIAN_POINT ( 'NONE',  ( 239.2173603368574959, 1.070082898007238326, -3.332413334892890155 ) ) ;
#10366=CARTESIAN_POINT ( 'NONE',  ( -239.1331760277428771, 1.386671646218362808, -11.66814526318957412 ) ) ;
#10367=CARTESIAN_POINT ( 'NONE',  ( 0.000000000000000000, -1.848645179579245124, 0.000000000000000000 ) ) ;
#10369=ORIENTED_EDGE ( 'NONE', *, *, #12357, .F. ) ;
#10372=EDGE_LOOP ( 'NONE', ( #6582, #10154 ) ) ;
#10381=CARTESIAN_POINT ( 'NONE',  ( -245.9694114599930401, -9.199502187900977290, -7.310239086664601871 ) ) ;
#10382=EDGE_CURVE ( 'NONE', #7222, #3384, #7304, .T. ) ;
#10384=SURFACE_STYLE_FILL_AREA ( #11398 ) ;
#10390=ORIENTED_EDGE ( 'NONE', *, *, #6249, .F. ) ;
#10392=DIRECTION ( 'NONE',  ( 0.000000000000000000, 1.000000000000000000, 0.000000000000000000 ) ) ;
#10393=CARTESIAN_POINT ( 'NONE',  ( 122.2593324768346008, 19.00000000000000000, 173.7755348299889988 ) ) ;
#10394=DIRECTION ( 'NONE',  ( 0.000000000000000000, 0.000000000000000000, 1.000000000000000000 ) ) ;
#10395=EDGE_CURVE ( 'NONE', #368, #11287, #9625, .T. ) ;
#10397=AXIS2_PLACEMENT_3D ( 'NONE', #2813, #12757, #5630 ) ;
#10404=AXIS2_PLACEMENT_3D ( 'NONE', #12421, #3208, #10279 ) ;
#10406=ORIENTED_EDGE ( 'NONE', *, *, #3454, .T. ) ;
#10407=CONICAL_SURFACE ( 'NONE', #2319, 6.500000000000000000, 0.7853981633974518317 ) ;
#10408=CARTESIAN_POINT ( 'NONE',  ( 240.5378997430557035, -3.246179722999635864, -1.312253685521740598 ) ) ;
#10409=AXIS2_PLACEMENT_3D ( 'NONE', #8127, #9187, #10051 ) ;
#10410=CARTESIAN_POINT ( 'NONE',  ( 229.9996576396049193, -3.477719343325218038, 0.4566469936247985473 ) ) ;
#10412=ORIENTED_EDGE ( 'NONE', *, *, #13037, .T. ) ;
#10414=CARTESIAN_POINT ( 'NONE',  ( -122.2593324768359935, 18.00000000000000000, -174.7755348299880040 ) ) ;
#10420=LINE ( 'NONE', #8434, #5607 ) ;
#10421=CIRCLE ( 'NONE', #11497, 10.00000000000000888 ) ;
#10425=ORIENTED_EDGE ( 'NONE', *, *, #2626, .F. ) ;
#10426=DIRECTION ( 'NONE',  ( 0.000000000000000000, -1.000000000000000000, 0.000000000000000000 ) ) ;
#10428=EDGE_LOOP ( 'NONE', ( #1902, #6566, #5042, #4762 ) ) ;
#10430=DIRECTION ( 'NONE',  ( 0.000000000000000000, 1.000000000000000000, 0.000000000000000000 ) ) ;
#10431=DIRECTION ( 'NONE',  ( 0.000000000000000000, -1.000000000000000000, 0.000000000000000000 ) ) ;
#10433=CARTESIAN_POINT ( 'NONE',  ( 3.053044470274350904E-14, -20.00000000000000000, -248.7999999999999829 ) ) ;
#10435=ADVANCED_FACE ( 'NONE', ( #7571 ), #11644, .F. ) ;
#10436=CARTESIAN_POINT ( 'NONE',  ( 239.0427084576656114, 0.5779638302498498748, -3.452011086619390934 ) ) ;
#10443=CARTESIAN_POINT ( 'NONE',  ( 0.000000000000000000, 18.00000000000000000, -208.0000000000000000 ) ) ;
#10446=CYLINDRICAL_SURFACE ( 'NONE', #6180, 5.100000000000000533 ) ;
#10451=CYLINDRICAL_SURFACE ( 'NONE', #1276, 195.0000000000000000 ) ;
#10457=CARTESIAN_POINT ( 'NONE',  ( 239.2304539310932512, -1.097329039956110419, 3.323615143768106073 ) ) ;
#10460=EDGE_CURVE ( 'NONE', #1965, #5629, #6674, .T. ) ;
#10462=ADVANCED_FACE ( 'NONE', ( #8641, #12697 ), #12446, .F. ) ;
#10473=CARTESIAN_POINT ( 'NONE',  ( 0.000000000000000000, -2.926905849962176352E-14, 0.000000000000000000 ) ) ;
#10475=DIRECTION ( 'NONE',  ( 0.000000000000000000, 0.000000000000000000, 1.000000000000000000 ) ) ;
#10477=ORIENTED_EDGE ( 'NONE', *, *, #4837, .F. ) ;
#10478=TOROIDAL_SURFACE ( 'NONE', #10253, 241.5000000000000000, 2.500000000000000000 ) ;
#10479=DIRECTION ( 'NONE',  ( 0.000000000000000000, -1.000000000000000000, 0.000000000000000000 ) ) ;
#10485=CARTESIAN_POINT ( 'NONE',  ( 0.000000000000000000, 25.00000000000000000, 0.000000000000000000 ) ) ;
#10494=CARTESIAN_POINT ( 'NONE',  ( -210.0000000000000000, 19.40000000000000213, -5.100000000000000533 ) ) ;
#10498=VERTEX_POINT ( 'NONE', #3696 ) ;
#10500=ORIENTED_EDGE ( 'NONE', *, *, #10836, .T. ) ;
#10501=VERTEX_POINT ( 'NONE', #6906 ) ;
#10508=ORIENTED_EDGE ( 'NONE', *, *, #10537, .T. ) ;
#10509=AXIS2_PLACEMENT_3D ( 'NONE', #12764, #6712, #5699 ) ;
#10510=DIRECTION ( 'NONE',  ( 0.000000000000000000, 0.000000000000000000, 1.000000000000000000 ) ) ;
#10511=ORIENTED_EDGE ( 'NONE', *, *, #1724, .T. ) ;
#10513=DIRECTION ( 'NONE',  ( 0.000000000000000000, 1.000000000000000000, 0.000000000000000000 ) ) ;
#10521=AXIS2_PLACEMENT_3D ( 'NONE', #5528, #1404, #1271 ) ;
#10528=ADVANCED_FACE ( 'NONE', ( #6774 ), #3890, .F. ) ;
#10535=AXIS2_PLACEMENT_3D ( 'NONE', #3251, #8337, #10256 ) ;
#10537=EDGE_CURVE ( 'NONE', #7619, #4563, #6835, .T. ) ;
#10539=CYLINDRICAL_SURFACE ( 'NONE', #5167, 5.499999999999998224 ) ;
#10541=CARTESIAN_POINT ( 'NONE',  ( -246.5049976566707812, -9.406509141698599308, 7.041467213310991013 ) ) ;
#10546=DIRECTION ( 'NONE',  ( 0.000000000000000000, 0.000000000000000000, 1.000000000000000000 ) ) ;
#10551=EDGE_CURVE ( 'NONE', #2233, #3500, #2608, .T. ) ;
#10559=VERTEX_POINT ( 'NONE', #5899 ) ;
#10561=ADVANCED_FACE ( 'NONE', ( #9897 ), #12426, .F. ) ;
#10562=ORIENTED_EDGE ( 'NONE', *, *, #12061, .T. ) ;
#10567=CARTESIAN_POINT ( 'NONE',  ( 0.000000000000000000, 19.00000000000000000, 0.000000000000000000 ) ) ;
#10568=CARTESIAN_POINT ( 'NONE',  ( 0.000000000000000000, 25.00000000000000000, 249.2999999999999829 ) ) ;
#10577=DIRECTION ( 'NONE',  ( 0.000000000000000000, 1.000000000000000000, 0.000000000000000000 ) ) ;
#10579=CARTESIAN_POINT ( 'NONE',  ( -197.8197553893909912, 19.00000000000000000, 69.77553482999131518 ) ) ;
#10580=CARTESIAN_POINT ( 'NONE',  ( -229.7581126986659399, 5.193038857911240314, 10.54715260651565067 ) ) ;
#10581=EDGE_CURVE ( 'NONE', #4800, #12659, #5511, .T. ) ;
#10587=CARTESIAN_POINT ( 'NONE',  ( 0.000000000000000000, 29.00000000000000000, 0.000000000000000000 ) ) ;
#10588=EDGE_LOOP ( 'NONE', ( #485, #3778, #11392, #12164 ) ) ;
#10590=CARTESIAN_POINT ( 'NONE',  ( 0.000000000000000000, -2.926905849962176352E-14, -239.0000000000000000 ) ) ;
#10593=LINE ( 'NONE', #1468, #1582 ) ;
#10594=ADVANCED_FACE ( 'NONE', ( #1487 ), #7523, .F. ) ;
#10596=CARTESIAN_POINT ( 'NONE',  ( 0.000000000000000000, 30.00000000000000000, 196.0000000000000000 ) ) ;
#10598=CARTESIAN_POINT ( 'NONE',  ( 0.000000000000000000, 25.00000000000000000, 0.000000000000000000 ) ) ;
#10603=ORIENTED_EDGE ( 'NONE', *, *, #2479, .T. ) ;
#10605=EDGE_CURVE ( 'NONE', #10156, #7690, #9491, .T. ) ;
#10607=CARTESIAN_POINT ( 'NONE',  ( -197.8197553893909912, 19.00000000000000000, 64.27553482999130097 ) ) ;
#10608=AXIS2_PLACEMENT_3D ( 'NONE', #2149, #892, #6229 ) ;
#10610=AXIS2_PLACEMENT_3D ( 'NONE', #2723, #8809, #10940 ) ;
#10617=CARTESIAN_POINT ( 'NONE',  ( -240.7431671954870183, 4.340241520815121490, 10.91924886820501683 ) ) ;
#10620=FACE_BOUND ( 'NONE', #7169, .T. ) ;
#10622=ORIENTED_EDGE ( 'NONE', *, *, #11108, .F. ) ;
#10625=ORIENTED_EDGE ( 'NONE', *, *, #1183, .F. ) ;
#10626=EDGE_CURVE ( 'NONE', #12676, #789, #10351, .T. ) ;
#10627=EDGE_CURVE ( 'NONE', #1045, #2184, #1295, .T. ) ;
#10632=CARTESIAN_POINT ( 'NONE',  ( 239.7229759539578140, 1.780302303981533552, -3.014465403428259194 ) ) ;
#10634=CARTESIAN_POINT ( 'NONE',  ( -238.9359252207569853, 1.030933083257997707, -11.70468920303632743 ) ) ;
#10635=DIRECTION ( 'NONE',  ( 1.000000000000000000, 0.000000000000000000, 0.000000000000000000 ) ) ;
#10636=DIRECTION ( 'NONE',  ( 0.000000000000000000, 0.000000000000000000, 1.000000000000000000 ) ) ;
#10638=CARTESIAN_POINT ( 'NONE',  ( -238.9184900493855821, -0.9919588255939099097, 11.70805706110242106 ) ) ;
#10639=ORIENTED_EDGE ( 'NONE', *, *, #10551, .T. ) ;
#10640=CARTESIAN_POINT ( 'NONE',  ( -240.7240246250781013, 4.307698618653014400, -10.93373802373241688 ) ) ;
#10641=LINE ( 'NONE', #12704, #4069 ) ;
#10642=AXIS2_PLACEMENT_3D ( 'NONE', #4684, #10694, #7761 ) ;
#10643=ADVANCED_FACE ( 'NONE', ( #12553 ), #4751, .F. ) ;
#10647=CARTESIAN_POINT ( 'NONE',  ( -229.8886654188676744, 9.323152609548129632, 7.161763144159140282 ) ) ;
#10656=EDGE_LOOP ( 'NONE', ( #11087, #11100, #827, #8834 ) ) ;
#10662=FACE_BOUND ( 'NONE', #6027, .T. ) ;
#10665=CARTESIAN_POINT ( 'NONE',  ( -229.9163773335792484, -9.982439288020907853, -6.209883811240605844 ) ) ;
#10666=CARTESIAN_POINT ( 'NONE',  ( 0.000000000000000000, 29.00000000000000000, 0.000000000000000000 ) ) ;
#10668=AXIS2_PLACEMENT_3D ( 'NONE', #10807, #5746, #9802 ) ;
#10672=ORIENTED_EDGE ( 'NONE', *, *, #1874, .F. ) ;
#10673=EDGE_CURVE ( 'NONE', #7200, #12258, #10283, .T. ) ;
#10677=DIRECTION ( 'NONE',  ( 0.000000000000000000, 0.000000000000000000, 1.000000000000000000 ) ) ;
#10681=DIRECTION ( 'NONE',  ( 0.000000000000000000, 0.000000000000000000, 1.000000000000000000 ) ) ;
#10685=DIRECTION ( 'NONE',  ( -0.000000000000000000, 1.000000000000000000, 0.000000000000000000 ) ) ;
#10688=VERTEX_POINT ( 'NONE', #3481 ) ;
#10693=FACE_OUTER_BOUND ( 'NONE', #8889, .T. ) ;
#10694=DIRECTION ( 'NONE',  ( 0.000000000000000000, 1.000000000000000000, 0.000000000000000000 ) ) ;
#10698=CYLINDRICAL_SURFACE ( 'NONE', #528, 249.7999999999999829 ) ;
#10703=ORIENTED_EDGE ( 'NONE', *, *, #6665, .T. ) ;
#10705=AXIS2_PLACEMENT_3D ( 'NONE', #4202, #7474, #11547 ) ;
#10706=VERTEX_POINT ( 'NONE', #6363 ) ;
#10708=CARTESIAN_POINT ( 'NONE',  ( -244.2081860509996716, 8.251870590816803741, -8.364754207297883326 ) ) ;
#10709=FACE_OUTER_BOUND ( 'NONE', #1843, .T. ) ;
#10715=VECTOR ( 'NONE', #3167, 1000.000000000000000 ) ;
#10716=AXIS2_PLACEMENT_3D ( 'NONE', #8879, #12942, #3811 ) ;
#10718=EDGE_CURVE ( 'NONE', #5331, #5784, #10420, .T. ) ;
#10726=CARTESIAN_POINT ( 'NONE',  ( -248.0831933713610056, 9.830508068705238856, 6.436117704883899115 ) ) ;
#10727=EDGE_LOOP ( 'NONE', ( #13022, #10277 ) ) ;
#10729=CARTESIAN_POINT ( 'NONE',  ( 122.2593324768346008, 29.00000000000000000, 162.7755348299889988 ) ) ;
#10735=CARTESIAN_POINT ( 'NONE',  ( 229.9784876240037477, 1.548910481047297560, -3.146875811102413767 ) ) ;
#10737=CARTESIAN_POINT ( 'NONE',  ( -248.9847817899753295, 10.23580904479008602, -5.770128482949556492 ) ) ;
#10739=CARTESIAN_POINT ( 'NONE',  ( -197.8197553893909912, 18.00000000000000000, 57.77553482999131518 ) ) ;
#10742=AXIS2_PLACEMENT_3D ( 'NONE', #12653, #5654, #9849 ) ;
#10743=FACE_OUTER_BOUND ( 'NONE', #6911, .T. ) ;
#10746=CARTESIAN_POINT ( 'NONE',  ( -239.8125244184153644, -2.098251440017480540, -11.56389750598835953 ) ) ;
#10748=DIRECTION ( 'NONE',  ( 0.000000000000000000, 0.000000000000000000, 1.000000000000000000 ) ) ;
#10749=CARTESIAN_POINT ( 'NONE',  ( 197.8197553893915028, 30.00000000000000000, -57.77553482998990830 ) ) ;
#10750=EDGE_CURVE ( 'NONE', #6828, #3737, #6432, .T. ) ;
#10755=ORIENTED_EDGE ( 'NONE', *, *, #12101, .T. ) ;
#10763=DIRECTION ( 'NONE',  ( 0.000000000000000000, 1.000000000000000000, 0.000000000000000000 ) ) ;
#10765=DIRECTION ( 'NONE',  ( 0.000000000000000000, 0.000000000000000000, 1.000000000000000000 ) ) ;
#10769=FACE_OUTER_BOUND ( 'NONE', #2890, .T. ) ;
#10770=ORIENTED_EDGE ( 'NONE', *, *, #5754, .T. ) ;
#10771=CARTESIAN_POINT ( 'NONE',  ( 122.2593324768346008, 19.00000000000000000, 168.2755348299889988 ) ) ;
#10774=CARTESIAN_POINT ( 'NONE',  ( 240.3826708216964789, -2.772967769359314882, -2.135567781667015108 ) ) ;
#10777=FACE_OUTER_BOUND ( 'NONE', #8231, .T. ) ;
#10780=ORIENTED_EDGE ( 'NONE', *, *, #946, .F. ) ;
#10782=EDGE_LOOP ( 'NONE', ( #9922, #8919, #10304, #9760 ) ) ;
#10784=CARTESIAN_POINT ( 'NONE',  ( -249.6387411365544438, -11.08439570779736805, -3.900217601532822265 ) ) ;
#10786=ADVANCED_FACE ( 'NONE', ( #560 ), #759, .F. ) ;
#10788=ADVANCED_FACE ( 'NONE', ( #8818 ), #8803, .F. ) ;
#10789=DIRECTION ( 'NONE',  ( 0.000000000000000000, 0.000000000000000000, -1.000000000000000000 ) ) ;
#10791=DIRECTION ( 'NONE',  ( 0.000000000000000000, 0.000000000000000000, 1.000000000000000000 ) ) ;
#10792=CARTESIAN_POINT ( 'NONE',  ( 0.000000000000000000, -11.79660968244690089, 0.000000000000000000 ) ) ;
#10794=LINE ( 'NONE', #742, #11327 ) ;
#10796=CARTESIAN_POINT ( 'NONE',  ( -229.9251749084369010, -10.18240290800271808, -5.876142929606890775 ) ) ;
#10799=CARTESIAN_POINT ( 'NONE',  ( -248.8285144558675768, 10.12619208588392716, -5.960099103720946978 ) ) ;
#10802=CARTESIAN_POINT ( 'NONE',  ( 122.2593324768346008, 30.00000000000000000, 173.7755348299889988 ) ) ;
#10803=ORIENTED_EDGE ( 'NONE', *, *, #2626, .T. ) ;
#10805=DIRECTION ( 'NONE',  ( 0.000000000000000000, -1.000000000000000000, 0.000000000000000000 ) ) ;
#10807=CARTESIAN_POINT ( 'NONE',  ( 71.82423009839129691, 19.40000000000000213, 197.3354503650404865 ) ) ;
#10811=DIRECTION ( 'NONE',  ( 0.000000000000000000, 0.000000000000000000, 1.000000000000000000 ) ) ;
#10822=CARTESIAN_POINT ( 'NONE',  ( -122.2593324768359935, 30.00000000000000000, -168.2755348299880040 ) ) ;
#10825=DIRECTION ( 'NONE',  ( 0.000000000000000000, 0.000000000000000000, 1.000000000000000000 ) ) ;
#10827=VECTOR ( 'NONE', #5346, 1000.000000000000000 ) ;
#10828=ORIENTED_EDGE ( 'NONE', *, *, #9412, .F. ) ;
#10829=CIRCLE ( 'NONE', #4226, 249.2999999999999829 ) ;
#10831=ORIENTED_EDGE ( 'NONE', *, *, #9987, .F. ) ;
#10832=CARTESIAN_POINT ( 'NONE',  ( -241.8128863246191997, 6.047237977407489140, -10.08137159590333276 ) ) ;
#10833=ORIENTED_EDGE ( 'NONE', *, *, #4365, .T. ) ;
#10836=EDGE_CURVE ( 'NONE', #9692, #7101, #295, .T. ) ;
#10837=ADVANCED_FACE ( 'NONE', ( #3611 ), #3467, .F. ) ;
#10840=DIRECTION ( 'NONE',  ( 8.659560562354926695E-17, 0.7071067811865480168, -0.7071067811865470176 ) ) ;
#10842=CARTESIAN_POINT ( 'NONE',  ( -229.9999671744778880, 11.74935745764778261, 0.7847617075409144549 ) ) ;
#10843=CIRCLE ( 'NONE', #12336, 6.500000000000005329 ) ;
#10849=ORIENTED_EDGE ( 'NONE', *, *, #763, .T. ) ;
#10852=CARTESIAN_POINT ( 'NONE',  ( -249.1881502584881787, -10.41621036620467677, -5.437499737166764824 ) ) ;
#10856=DIRECTION ( 'NONE',  ( 0.000000000000000000, 1.000000000000000000, 0.000000000000000000 ) ) ;
#10857=DIRECTION ( 'NONE',  ( 0.000000000000000000, 0.000000000000000000, -1.000000000000000000 ) ) ;
#10860=DIRECTION ( 'NONE',  ( 0.000000000000000000, 0.000000000000000000, 1.000000000000000000 ) ) ;
#10863=CARTESIAN_POINT ( 'NONE',  ( 122.2593324768334071, 19.00000000000000000, -162.7755348299894820 ) ) ;
#10864=B_SPLINE_CURVE_WITH_KNOTS ( 'NONE', 3,
 ( #1472, #7665, #8736, #5535, #12796, #1538, #8612, #3660, #12669, #7731, #5604, #12866, #7602, #6745, #11677, #10665, #10796, #1665, #672, #4723, #8801, #3730, #7796, #7138, #6999, #5051, #3930, #10001, #10997, #1063, #12007, #9002, #8209, #869, #8939, #10065, #6132, #9128, #937, #1809, #73, #4929, #4128, #12132, #3115, #5120, #11194, #2914, #2000 ),
 .UNSPECIFIED., .F., .F.,
 ( 4, 2, 2, 2, 2, 2, 2, 2, 2, 1, 2, 2, 2, 2, 2, 2, 2, 2, 2, 2, 2, 2, 2, 2, 4 ),
 ( 6.997332055170240228E-20, 0.002296365050924792459, 0.003444547576387190207, 0.004592730101849587521, 0.006889095152774382148, 0.008037277678236776426, 0.009185460203699171572, 0.01148182525462396186, 0.01263000778008635874, 0.01377819030554875562, 0.01492637283101115250, 0.01607455535647354938, 0.01837092040739833967, 0.01951910293286073655, 0.02066728545832313343, 0.02296365050924792373, 0.02411183303471032408, 0.02526001556017272442, 0.02755638061109752512, 0.02985274566202231541, 0.03100092818748471230, 0.03214911071294710571, 0.03444547576387189253, 0.03559365828933428594, 0.03674184081479667241 ),
 .UNSPECIFIED. ) ;
#10865=ADVANCED_FACE ( 'NONE', ( #6759 ), #9017, .T. ) ;
#10866=AXIS2_PLACEMENT_3D ( 'NONE', #1283, #4275, #7350 ) ;
#10867=CARTESIAN_POINT ( 'NONE',  ( -249.7763361845706527, 11.55065150977181787, -2.186104012435922339 ) ) ;
#10870=VERTEX_POINT ( 'NONE', #5822 ) ;
#10878=CARTESIAN_POINT ( 'NONE',  ( -197.8197553893924976, 30.00000000000000000, -64.27553482998719403 ) ) ;
#10883=ORIENTED_EDGE ( 'NONE', *, *, #3426, .T. ) ;
#10886=VERTEX_POINT ( 'NONE', #687 ) ;
#10887=ADVANCED_FACE ( 'NONE', ( #12880 ), #1134, .F. ) ;
#10889=CARTESIAN_POINT ( 'NONE',  ( 240.0429366796232387, -2.111384149273799249, 2.791848677268702339 ) ) ;
#10890=ORIENTED_EDGE ( 'NONE', *, *, #12261, .F. ) ;
#10894=DIRECTION ( 'NONE',  ( 0.000000000000000000, 1.000000000000000000, 0.000000000000000000 ) ) ;
#10896=DIRECTION ( 'NONE',  ( 1.000000000000000000, 0.000000000000000000, 0.000000000000000000 ) ) ;
#10897=ORIENTED_EDGE ( 'NONE', *, *, #7366, .T. ) ;
#10900=CARTESIAN_POINT ( 'NONE',  ( -238.9443119646329876, 1.049071724482780299, 11.70307552132215534 ) ) ;
#10902=AXIS2_PLACEMENT_3D ( 'NONE', #1374, #9558, #5440 ) ;
#10907=CARTESIAN_POINT ( 'NONE',  ( -229.9961257339021188, 11.67486194030054847, -1.531634783006589950 ) ) ;
#10915=DIRECTION ( 'NONE',  ( 0.000000000000000000, 0.000000000000000000, 1.000000000000000000 ) ) ;
#10916=EDGE_CURVE ( 'NONE', #12887, #12366, #5170, .T. ) ;
#10919=CARTESIAN_POINT ( 'NONE',  ( -249.7544427812662775, -11.44486579096268386, -2.664765659934758002 ) ) ;
#10921=AXIS2_PLACEMENT_3D ( 'NONE', #4141, #2070, #812 ) ;
#10931=DIRECTION ( 'NONE',  ( 0.000000000000000000, 1.000000000000000000, 0.000000000000000000 ) ) ;
#10932=ADVANCED_FACE ( 'NONE', ( #2800 ), #6625, .F. ) ;
#10935=CARTESIAN_POINT ( 'NONE',  ( -249.2724874750445281, 10.50618518648595590, -5.261424415981784897 ) ) ;
#10938=VERTEX_POINT ( 'NONE', #12744 ) ;
#10939=ORIENTED_EDGE ( 'NONE', *, *, #4505, .F. ) ;
#10940=DIRECTION ( 'NONE',  ( 0.000000000000000000, 0.000000000000000000, 1.000000000000000000 ) ) ;
#10941=DIRECTION ( 'NONE',  ( 0.000000000000000000, 0.000000000000000000, -1.000000000000000000 ) ) ;
#10947=DIRECTION ( 'NONE',  ( 0.000000000000000000, 0.7071067811865480168, 0.7071067811865470176 ) ) ;
#10953=DIRECTION ( 'NONE',  ( 0.000000000000000000, 0.000000000000000000, 1.000000000000000000 ) ) ;
#10955=CIRCLE ( 'NONE', #1385, 6.500000000000005329 ) ;
#10959=CARTESIAN_POINT ( 'NONE',  ( 240.1560849993302611, -2.274296953689764145, 2.660406300277259994 ) ) ;
#10964=DIRECTION ( 'NONE',  ( 0.000000000000000000, 0.000000000000000000, 1.000000000000000000 ) ) ;
#10966=FACE_OUTER_BOUND ( 'NONE', #2662, .T. ) ;
#10968=EDGE_CURVE ( 'NONE', #11921, #2672, #404, .T. ) ;
#10970=CARTESIAN_POINT ( 'NONE',  ( -239.1225034092054500, -1.367596997490950539, 11.67014394435902958 ) ) ;
#10971=ORIENTED_EDGE ( 'NONE', *, *, #12395, .T. ) ;
#10972=CARTESIAN_POINT ( 'NONE',  ( -239.5361044668155159, 1.848645179572584896, 11.60366368868220022 ) ) ;
#10975=CARTESIAN_POINT ( 'NONE',  ( 240.2344515802417959, -2.410164965830901451, -2.538069655751040266 ) ) ;
#10977=CARTESIAN_POINT ( 'NONE',  ( 0.000000000000000000, 19.00000000000000000, -195.0000000000000000 ) ) ;
#10978=CARTESIAN_POINT ( 'NONE',  ( -229.9849491715392844, 11.45184952815656310, -2.657836336733081950 ) ) ;
#10979=FACE_BOUND ( 'NONE', #551, .T. ) ;
#10984=CARTESIAN_POINT ( 'NONE',  ( -238.9324305500051651, -1.023275421966679311, -11.70536273065333965 ) ) ;
#10985=AXIS2_PLACEMENT_3D ( 'NONE', #11271, #9011, #9074 ) ;
#10988=CARTESIAN_POINT ( 'NONE',  ( -248.6772030005851093, -10.03733143289317908, -6.108624101512084792 ) ) ;
#10993=DIRECTION ( 'NONE',  ( 0.000000000000000000, 1.000000000000000000, 0.000000000000000000 ) ) ;
#10994=CARTESIAN_POINT ( 'NONE',  ( -197.8197553893924976, 29.00000000000000000, -69.77553482998720824 ) ) ;
#10995=DIRECTION ( 'NONE',  ( 0.000000000000000000, -1.000000000000000000, 0.000000000000000000 ) ) ;
#10997=CARTESIAN_POINT ( 'NONE',  ( -229.9810369278718554, -11.37375499241069754, 3.048046500125209501 ) ) ;
#10998=DIRECTION ( 'NONE',  ( 0.000000000000000000, 0.000000000000000000, 1.000000000000000000 ) ) ;
#11000=ORIENTED_EDGE ( 'NONE', *, *, #8234, .F. ) ;
#11008=CARTESIAN_POINT ( 'NONE',  ( -245.3907676188946994, -8.935007734252014444, 7.630737089623142566 ) ) ;
#11016=ORIENTED_EDGE ( 'NONE', *, *, #7704, .F. ) ;
#11019=ORIENTED_EDGE ( 'NONE', *, *, #3171, .T. ) ;
#11021=CARTESIAN_POINT ( 'NONE',  ( -248.8121438751408334, 10.11580272837505667, 5.977715408700031929 ) ) ;
#11024=DIRECTION ( 'NONE',  ( 0.000000000000000000, 0.000000000000000000, 1.000000000000000000 ) ) ;
#11026=CARTESIAN_POINT ( 'NONE',  ( -239.5361044668159991, -1.848645179572815156, 11.60366368868215758 ) ) ;
#11027=EDGE_CURVE ( 'NONE', #10501, #1505, #3456, .T. ) ;
#11031=CARTESIAN_POINT ( 'NONE',  ( -238.9571479212536076, 1.076402573844281951, 11.70061130409436778 ) ) ;
#11032=ORIENTED_EDGE ( 'NONE', *, *, #816, .F. ) ;
#11033=CARTESIAN_POINT ( 'NONE',  ( 239.7985776503645354, -1.848645179573700004, -2.971954070984049956 ) ) ;
#11035=CARTESIAN_POINT ( 'NONE',  ( -210.0000000000000000, 19.40000000000000213, 5.100000000000000533 ) ) ;
#11036=CONICAL_SURFACE ( 'NONE', #5937, 5.500000000000005329, 0.7853981633974461696 ) ;
#11037=AXIS2_PLACEMENT_3D ( 'NONE', #10309, #3105, #8390 ) ;
#11038=CARTESIAN_POINT ( 'NONE',  ( -229.9803371157412641, 11.35915247731612254, -3.029940864557863378 ) ) ;
#11039=CARTESIAN_POINT ( 'NONE',  ( 238.9743710777160857, 8.519355453646930632E-11, 3.499999942258626984 ) ) ;
#11045=ORIENTED_EDGE ( 'NONE', *, *, #12738, .F. ) ;
#11046=AXIS2_PLACEMENT_3D ( 'NONE', #7656, #7593, #3724 ) ;
#11047=CARTESIAN_POINT ( 'NONE',  ( 0.000000000000000000, -1.848645179579245124, -239.8169934640529846 ) ) ;
#11048=ORIENTED_EDGE ( 'NONE', *, *, #4013, .T. ) ;
#11051=VERTEX_POINT ( 'NONE', #9587 ) ;
#11053=CARTESIAN_POINT ( 'NONE',  ( -248.9237871404848761, -10.19078078235692431, 5.849051583267943499 ) ) ;
#11054=VERTEX_POINT ( 'NONE', #12720 ) ;
#11061=AXIS2_PLACEMENT_3D ( 'NONE', #7308, #5496, #10362 ) ;
#11062=CYLINDRICAL_SURFACE ( 'NONE', #7900, 249.7999999999999829 ) ;
#11068=ORIENTED_EDGE ( 'NONE', *, *, #4013, .F. ) ;
#11072=CARTESIAN_POINT ( 'NONE',  ( 3.010181832304193602E-14, 22.00000000000000000, 245.7999999999999829 ) ) ;
#11075=CARTESIAN_POINT ( 'NONE',  ( -197.8197553893909912, 30.00000000000000000, 58.77553482999130807 ) ) ;
#11080=ORIENTED_EDGE ( 'NONE', *, *, #6699, .T. ) ;
#11081=ADVANCED_FACE ( 'NONE', ( #5596 ), #88, .F. ) ;
#11086=ORIENTED_EDGE ( 'NONE', *, *, #11781, .F. ) ;
#11087=ORIENTED_EDGE ( 'NONE', *, *, #8511, .F. ) ;
#11090=CARTESIAN_POINT ( 'NONE',  ( -249.6587182941822221, 11.13358978266949961, 3.756204109565398852 ) ) ;
#11094=CARTESIAN_POINT ( 'NONE',  ( -245.4195491717965751, 8.949151682147107323, 7.614144253907443094 ) ) ;
#11095=ORIENTED_EDGE ( 'NONE', *, *, #11459, .F. ) ;
#11096=CARTESIAN_POINT ( 'NONE',  ( -239.0623374290204595, -1.272322106364155214, 11.68094603905051088 ) ) ;
#11099=CARTESIAN_POINT ( 'NONE',  ( -238.7109915808064500, 2.244475480116206709E-14, 11.74999999995203126 ) ) ;
#11100=ORIENTED_EDGE ( 'NONE', *, *, #1899, .F. ) ;
#11101=CIRCLE ( 'NONE', #2154, 6.500000000000005329 ) ;
#11105=CARTESIAN_POINT ( 'NONE',  ( 238.9743710777160857, 8.519355453646930632E-11, 3.499999942258626984 ) ) ;
#11108=EDGE_CURVE ( 'NONE', #1185, #6448, #11468, .T. ) ;
#11110=CARTESIAN_POINT ( 'NONE',  ( 0.000000000000000000, 19.00000000000000000, -213.5000000000000000 ) ) ;
#11113=CARTESIAN_POINT ( 'NONE',  ( -238.7322540142980927, -0.3343210646034411870, -11.74538300442941541 ) ) ;
#11116=CARTESIAN_POINT ( 'NONE',  ( -249.6893775633026848, -11.21617121157748542, 3.501676138744457933 ) ) ;
#11118=CIRCLE ( 'NONE', #12398, 6.500000000000005329 ) ;
#11120=DIRECTION ( 'NONE',  ( 0.000000000000000000, -1.000000000000000000, 0.000000000000000000 ) ) ;
#11122=CIRCLE ( 'NONE', #8152, 6.499999999999999112 ) ;
#11123=CARTESIAN_POINT ( 'NONE',  ( -241.3731105455979389, -5.422910281729395265, -10.42375653607661334 ) ) ;
#11124=EDGE_CURVE ( 'NONE', #7072, #12496, #5930, .T. ) ;
#11137=CARTESIAN_POINT ( 'NONE',  ( 71.82423009839129691, 30.00000000000000000, 190.8354503650404865 ) ) ;
#11138=CYLINDRICAL_SURFACE ( 'NONE', #7209, 5.500000000000005329 ) ;
#11139=LINE ( 'NONE', #7693, #8722 ) ;
#11141=CARTESIAN_POINT ( 'NONE',  ( 239.7985776503625175, 1.848645179571945185, -2.971954070985139751 ) ) ;
#11146=CARTESIAN_POINT ( 'NONE',  ( -241.2291919110257368, -5.202024195681614671, 10.53597307945316963 ) ) ;
#11147=ORIENTED_EDGE ( 'NONE', *, *, #2555, .F. ) ;
#11148=FACE_BOUND ( 'NONE', #10356, .T. ) ;
#11149=CARTESIAN_POINT ( 'NONE',  ( 229.9737165936600718, -0.4586479115007087159, 3.477305464001514412 ) ) ;
#11150=VERTEX_POINT ( 'NONE', #737 ) ;
#11151=EDGE_LOOP ( 'NONE', ( #7051, #12067, #1595, #4609 ) ) ;
#11154=CONICAL_SURFACE ( 'NONE', #7117, 5.500000000000005329, 0.7853981633974461696 ) ;
#11155=CARTESIAN_POINT ( 'NONE',  ( -248.2181897916257185, 9.855491095746206298, 6.397958699693558238 ) ) ;
#11156=SHAPE_REPRESENTATION ( 'Internal Mounting Flange Ring', ( #805 ), #1235 ) ;
#11160=CARTESIAN_POINT ( 'NONE',  ( -243.1833766791151277, 7.470616520408806416, 9.069320236312849559 ) ) ;
#11165=CARTESIAN_POINT ( 'NONE',  ( 0.000000000000000000, 0.000000000000000000, 0.000000000000000000 ) ) ;
#11167=AXIS2_PLACEMENT_3D ( 'NONE', #463, #588, #1592 ) ;
#11169=CARTESIAN_POINT ( 'NONE',  ( 240.1881190900947445, 2.326983775934756693, 2.614448608538753938 ) ) ;
#11178=CARTESIAN_POINT ( 'NONE',  ( -239.0839813682398187, -1.310043317831860010, -11.67696021831089759 ) ) ;
#11179=ORIENTED_EDGE ( 'NONE', *, *, #6959, .F. ) ;
#11180=CARTESIAN_POINT ( 'NONE',  ( -249.6782235448949905, 11.18495322599711450, -3.599910145184412436 ) ) ;
#11181=CARTESIAN_POINT ( 'NONE',  ( -122.2593324768321992, 19.00000000000000000, 173.7755348299905052 ) ) ;
#11183=CARTESIAN_POINT ( 'NONE',  ( -249.6782235448939389, -11.18495322599737740, 3.599910145183604193 ) ) ;
#11184=VERTEX_POINT ( 'NONE', #7858 ) ;
#11188=CARTESIAN_POINT ( 'NONE',  ( -246.7375545308477456, -9.485935069199962655, -6.933947691877577313 ) ) ;
#11192=DIRECTION ( 'NONE',  ( 0.000000000000000000, -1.000000000000000000, 0.000000000000000000 ) ) ;
#11194=CARTESIAN_POINT ( 'NONE',  ( -229.7006282228656744, -0.7680959398531020943, 11.73127646695761506 ) ) ;
#11198=DIRECTION ( 'NONE',  ( 0.000000000000000000, 1.000000000000000000, 0.000000000000000000 ) ) ;
#11202=CARTESIAN_POINT ( 'NONE',  ( 0.000000000000000000, 2.772967769359004908, 0.000000000000000000 ) ) ;
#11204=CARTESIAN_POINT ( 'NONE',  ( 71.82423009839129691, 30.00000000000000000, 190.8354503650404865 ) ) ;
#11205=DIRECTION ( 'NONE',  ( 0.000000000000000000, 0.000000000000000000, 1.000000000000000000 ) ) ;
#11208=CARTESIAN_POINT ( 'NONE',  ( -244.0310755556703270, -8.130894646083811850, 8.482269560327180713 ) ) ;
#11212=EDGE_CURVE ( 'NONE', #4889, #3851, #8698, .T. ) ;
#11219=VECTOR ( 'NONE', #2725, 1000.000000000000000 ) ;
#11223=CARTESIAN_POINT ( 'NONE',  ( -241.6806182397082807, 5.858727364634749968, 10.18566440554176289 ) ) ;
#11231=CARTESIAN_POINT ( 'NONE',  ( 239.4141849554329724, 1.410389959096011392, 3.203344682971027702 ) ) ;
#11232=DIRECTION ( 'NONE',  ( 0.000000000000000000, -1.000000000000000000, 0.000000000000000000 ) ) ;
#11233=CARTESIAN_POINT ( 'NONE',  ( -197.8197553893909912, 30.00000000000000000, 64.27553482999130097 ) ) ;
#11235=DIRECTION ( 'NONE',  ( 0.000000000000000000, 0.000000000000000000, 1.000000000000000000 ) ) ;
#11240=LINE ( 'NONE', #9450, #10715 ) ;
#11244=EDGE_CURVE ( 'NONE', #9162, #4030, #8730, .T. ) ;
#11249=CIRCLE ( 'NONE', #11037, 6.499999999999999112 ) ;
#11250=VECTOR ( 'NONE', #3402, 1000.000000000000000 ) ;
#11256=AXIS2_PLACEMENT_3D ( 'NONE', #6826, #1690, #10084 ) ;
#11257=CARTESIAN_POINT ( 'NONE',  ( -243.6022064637596145, -7.815160977192930680, -8.774769252031678235 ) ) ;
#11265=TOROIDAL_SURFACE ( 'NONE', #11901, 247.7999999999999829, 2.000000000000000000 ) ;
#11266=DIRECTION ( 'NONE',  ( 0.000000000000000000, 1.000000000000000000, 0.000000000000000000 ) ) ;
#11267=ORIENTED_EDGE ( 'NONE', *, *, #9962, .F. ) ;
#11269=AXIS2_PLACEMENT_3D ( 'NONE', #7530, #4325, #12716 ) ;
#11271=CARTESIAN_POINT ( 'NONE',  ( -197.8197553893909912, 30.00000000000000000, 64.27553482999130097 ) ) ;
#11273=CARTESIAN_POINT ( 'NONE',  ( 239.1385365879861524, -0.8886010998478790501, -3.385772393335910291 ) ) ;
#11274=AXIS2_PLACEMENT_3D ( 'NONE', #845, #6722, #1585 ) ;
#11275=FACE_OUTER_BOUND ( 'NONE', #10782, .T. ) ;
#11279=CARTESIAN_POINT ( 'NONE',  ( 0.000000000000000000, 0.000000000000000000, 0.000000000000000000 ) ) ;
#11281=CARTESIAN_POINT ( 'NONE',  ( -242.6830939053905638, -7.008887182000894889, 9.430537150680942560 ) ) ;
#11283=CARTESIAN_POINT ( 'NONE',  ( 240.4181131690832558, -2.891045149246452617, -1.982248008101765935 ) ) ;
#11285=LINE ( 'NONE', #9352, #3372 ) ;
#11287=VERTEX_POINT ( 'NONE', #796 ) ;
#11289=DIRECTION ( 'NONE',  ( 0.000000000000000000, -1.000000000000000000, 0.000000000000000000 ) ) ;
#11291=EDGE_CURVE ( 'NONE', #6697, #12416, #7225, .T. ) ;
#11294=CARTESIAN_POINT ( 'NONE',  ( -246.7375545285866849, 9.485935068452450381, 6.933947692770260574 ) ) ;
#11297=CARTESIAN_POINT ( 'NONE',  ( -197.8197553893924976, 19.00000000000000000, -64.27553482998719403 ) ) ;
#11298=EDGE_CURVE ( 'NONE', #552, #4800, #835, .T. ) ;
#11302=EDGE_LOOP ( 'NONE', ( #3209, #8023 ) ) ;
#11303=ORIENTED_EDGE ( 'NONE', *, *, #4594, .F. ) ;
#11305=CARTESIAN_POINT ( 'NONE',  ( -197.8197553893909912, 19.00000000000000000, 69.77553482999131518 ) ) ;
#11315=CIRCLE ( 'NONE', #7479, 240.3921568627444856 ) ;
#11320=CARTESIAN_POINT ( 'NONE',  ( -248.8244828231703138, -10.12360735459863115, 5.964490512234371877 ) ) ;
#11321=ORIENTED_EDGE ( 'NONE', *, *, #9993, .F. ) ;
#11325=CARTESIAN_POINT ( 'NONE',  ( -245.4374131367196696, -8.957880036294859849, -7.603877363506748921 ) ) ;
#11327=VECTOR ( 'NONE', #6677, 1000.000000000000000 ) ;
#11329=CARTESIAN_POINT ( 'NONE',  ( 239.2050160255199955, -1.043887935101727393, 3.340720568042238714 ) ) ;
#11331=CARTESIAN_POINT ( 'NONE',  ( 240.6324715326043702, 3.499918298005177952, 0.3875926901506949740 ) ) ;
#11334=ORIENTED_EDGE ( 'NONE', *, *, #3606, .F. ) ;
#11337=LINE ( 'NONE', #342, #8284 ) ;
#11339=CARTESIAN_POINT ( 'NONE',  ( -122.2593324768321992, 30.00000000000000000, 168.2755348299905052 ) ) ;
#11342=EDGE_CURVE ( 'NONE', #8497, #12659, #4854, .T. ) ;
#11346=DIRECTION ( 'NONE',  ( 0.000000000000000000, 0.000000000000000000, 1.000000000000000000 ) ) ;
#11348=VECTOR ( 'NONE', #8897, 1000.000000000000000 ) ;
#11350=CARTESIAN_POINT ( 'NONE',  ( 229.9973412510026662, -3.321846415627111693, -1.126016662849602223 ) ) ;
#11354=EDGE_CURVE ( 'NONE', #13033, #982, #24, .T. ) ;
#11356=CARTESIAN_POINT ( 'NONE',  ( 0.000000000000000000, 29.00000000000000000, 208.0000000000000000 ) ) ;
#11358=CIRCLE ( 'NONE', #6254, 195.0000000000000000 ) ;
#11359=AXIS2_PLACEMENT_3D ( 'NONE', #5485, #301, #12618 ) ;
#11361=CARTESIAN_POINT ( 'NONE',  ( 0.000000000000000000, -3.327561323230890267, 0.000000000000000000 ) ) ;
#11364=CARTESIAN_POINT ( 'NONE',  ( -243.3200464879880371, 7.587187391486287069, 8.972284947528141430 ) ) ;
#11366=DIRECTION ( 'NONE',  ( 1.000000000000000000, 0.000000000000000000, 0.000000000000000000 ) ) ;
#11370=ORIENTED_EDGE ( 'NONE', *, *, #10395, .T. ) ;
#11372=EDGE_CURVE ( 'NONE', #3155, #1462, #8066, .T. ) ;
#11377=DIRECTION ( 'NONE',  ( 8.659560562354913137E-17, -0.7071067811865489050, 0.7071067811865460184 ) ) ;
#11380=CARTESIAN_POINT ( 'NONE',  ( 2.394184492333075617E-14, 29.00000000000000000, -195.0000000000000000 ) ) ;
#11391=CARTESIAN_POINT ( 'NONE',  ( 240.3826708216964789, -2.772967769359314882, -2.135567781667015108 ) ) ;
#11392=ORIENTED_EDGE ( 'NONE', *, *, #5154, .T. ) ;
#11396=CARTESIAN_POINT ( 'NONE',  ( -244.0507507057079977, -8.147415050172172712, -8.468315434781628070 ) ) ;
#11397=CIRCLE ( 'NONE', #12882, 248.1666666666679930 ) ;
#11398=FILL_AREA_STYLE ('',( #261 ) ) ;
#11406=FACE_OUTER_BOUND ( 'NONE', #3223, .T. ) ;
#11409=CARTESIAN_POINT ( 'NONE',  ( 6.735557395310435121E-16, 19.00000000000000000, -213.5000000000000000 ) ) ;
#11412=FACE_OUTER_BOUND ( 'NONE', #6946, .T. ) ;
#11416=CARTESIAN_POINT ( 'NONE',  ( 122.2593324768346008, 30.00000000000000000, 162.7755348299889988 ) ) ;
#11417=CARTESIAN_POINT ( 'NONE',  ( 229.9785086005968537, -1.552204380456203348, 3.145362046007984080 ) ) ;
#11419=EDGE_CURVE ( 'NONE', #6421, #2427, #1890, .T. ) ;
#11420=ORIENTED_EDGE ( 'NONE', *, *, #6606, .T. ) ;
#11421=EDGE_CURVE ( 'NONE', #12564, #4415, #8265, .T. ) ;
#11423=DIRECTION ( 'NONE',  ( 0.000000000000000000, -1.000000000000000000, 0.000000000000000000 ) ) ;
#11428=ADVANCED_FACE ( 'NONE', ( #3047 ), #992, .F. ) ;
#11430=DIRECTION ( 'NONE',  ( -1.000000000000000000, 0.000000000000000000, 0.000000000000000000 ) ) ;
#11435=DIRECTION ( 'NONE',  ( 0.000000000000000000, 1.000000000000000000, 0.000000000000000000 ) ) ;
#11438=CARTESIAN_POINT ( 'NONE',  ( 0.000000000000000000, 19.00000000000000000, 202.4999999999999716 ) ) ;
#11439=CARTESIAN_POINT ( 'NONE',  ( -238.7146392957941430, 0.1450841617578550458, -11.74918863377693690 ) ) ;
#11448=VERTEX_POINT ( 'NONE', #1928 ) ;
#11452=DIRECTION ( 'NONE',  ( 0.000000000000000000, 1.000000000000000000, 0.000000000000000000 ) ) ;
#11457=CARTESIAN_POINT ( 'NONE',  ( -197.8197553893924976, 30.00000000000000000, -70.77553482998720824 ) ) ;
#11459=EDGE_CURVE ( 'NONE', #11287, #5843, #7001, .T. ) ;
#11464=CARTESIAN_POINT ( 'NONE',  ( -210.0000000000000000, 30.00000000000000000, 0.000000000000000000 ) ) ;
#11465=EDGE_LOOP ( 'NONE', ( #3894, #2685, #12189, #10939 ) ) ;
#11468=LINE ( 'NONE', #2397, #3806 ) ;
#11469=CARTESIAN_POINT ( 'NONE',  ( 197.8197553893920144, 30.00000000000000000, 64.27553482998850143 ) ) ;
#11474=CYLINDRICAL_SURFACE ( 'NONE', #11522, 249.7999999999999829 ) ;
#11476=CIRCLE ( 'NONE', #8067, 5.500000000000005329 ) ;
#11482=CARTESIAN_POINT ( 'NONE',  ( 240.5163796274145511, -3.187645493303870037, 1.494965077496835049 ) ) ;
#11483=CONICAL_SURFACE ( 'NONE', #6161, 6.500000000000005329, 0.7853981633974476129 ) ;
#11486=ORIENTED_EDGE ( 'NONE', *, *, #3438, .T. ) ;
#11488=CARTESIAN_POINT ( 'NONE',  ( -122.2593324768359935, 29.00000000000000000, -168.2755348299880040 ) ) ;
#11497=AXIS2_PLACEMENT_3D ( 'NONE', #4553, #4477, #11771 ) ;
#11498=ORIENTED_EDGE ( 'NONE', *, *, #4895, .F. ) ;
#11499=DIRECTION ( 'NONE',  ( 0.000000000000000000, 0.000000000000000000, 1.000000000000000000 ) ) ;
#11502=CARTESIAN_POINT ( 'NONE',  ( -197.8197553893924976, 30.00000000000000000, -58.77553482998720114 ) ) ;
#11504=ORIENTED_EDGE ( 'NONE', *, *, #3938, .T. ) ;
#11505=CIRCLE ( 'NONE', #2971, 6.500000000000005329 ) ;
#11506=DIRECTION ( 'NONE',  ( 0.000000000000000000, 1.000000000000000000, 0.000000000000000000 ) ) ;
#11511=CARTESIAN_POINT ( 'NONE',  ( -238.8528788548577779, 0.8456725619206635347, -11.72072902431185959 ) ) ;
#11514=EDGE_CURVE ( 'NONE', #2818, #6490, #2187, .T. ) ;
#11516=VECTOR ( 'NONE', #8481, 1000.000000000000000 ) ;
#11520=CARTESIAN_POINT ( 'NONE',  ( 0.000000000000000000, 30.00000000000000000, 196.0000000000000000 ) ) ;
#11522=AXIS2_PLACEMENT_3D ( 'NONE', #11279, #5204, #9279 ) ;
#11530=CARTESIAN_POINT ( 'NONE',  ( -240.6798348123905669, -4.210664053393288420, -10.96963869240667755 ) ) ;
#11531=ORIENTED_EDGE ( 'NONE', *, *, #10342, .T. ) ;
#11532=CARTESIAN_POINT ( 'NONE',  ( 239.4717458110699226, -1.490203034777392022, 3.166904956833142215 ) ) ;
#11534=CARTESIAN_POINT ( 'NONE',  ( 240.3826708216974737, 2.772967769358989809, 2.135567781667440102 ) ) ;
#11537=CARTESIAN_POINT ( 'NONE',  ( 7.960204194457791533E-16, 18.00000000000000000, 214.5000000000000000 ) ) ;
#11538=ORIENTED_EDGE ( 'NONE', *, *, #10125, .T. ) ;
#11539=CARTESIAN_POINT ( 'NONE',  ( -249.7931653183007086, -11.67801679920997593, -1.333825740846608321 ) ) ;
#11544=CARTESIAN_POINT ( 'NONE',  ( 0.000000000000000000, 0.000000000000000000, 0.000000000000000000 ) ) ;
#11545=DIRECTION ( 'NONE',  ( 0.000000000000000000, 0.000000000000000000, 1.000000000000000000 ) ) ;
#11546=EDGE_CURVE ( 'NONE', #4563, #982, #2735, .T. ) ;
#11547=DIRECTION ( 'NONE',  ( 0.000000000000000000, 0.000000000000000000, -1.000000000000000000 ) ) ;
#11549=DIRECTION ( 'NONE',  ( 0.000000000000000000, -1.000000000000000000, 0.000000000000000000 ) ) ;
#11552=DIRECTION ( 'NONE',  ( 0.000000000000000000, 0.000000000000000000, 1.000000000000000000 ) ) ;
#11553=VECTOR ( 'NONE', #3494, 1000.000000000000000 ) ;
#11558=AXIS2_PLACEMENT_3D ( 'NONE', #3736, #940, #10998 ) ;
#11568=DIRECTION ( 'NONE',  ( 0.000000000000000000, 1.000000000000000000, 0.000000000000000000 ) ) ;
#11571=VECTOR ( 'NONE', #3742, 1000.000000000000114 ) ;
#11575=CARTESIAN_POINT ( 'NONE',  ( -197.8197553893924976, 19.00000000000000000, -64.27553482998719403 ) ) ;
#11576=CARTESIAN_POINT ( 'NONE',  ( -239.3871000706272696, 1.704623200064774302, -11.62580518457323642 ) ) ;
#11579=CIRCLE ( 'NONE', #6253, 195.0000000000000000 ) ;
#11582=VERTEX_POINT ( 'NONE', #4383 ) ;
#11586=CARTESIAN_POINT ( 'NONE',  ( -241.3198063618330877, 5.342363202599722527, -10.46527477498853820 ) ) ;
#11588=EDGE_CURVE ( 'NONE', #1904, #4880, #9559, .T. ) ;
#11591=FACE_OUTER_BOUND ( 'NONE', #5811, .T. ) ;
#11594=VECTOR ( 'NONE', #12340, 1000.000000000000114 ) ;
#11595=CARTESIAN_POINT ( 'NONE',  ( -229.7148150354796314, 2.664985348179264690, 11.45030177774321167 ) ) ;
#11597=CARTESIAN_POINT ( 'NONE',  ( -210.0000000000000000, 19.40000000000000213, 0.000000000000000000 ) ) ;
#11599=ADVANCED_FACE ( 'NONE', ( #719 ), #7640, .T. ) ;
#11600=CARTESIAN_POINT ( 'NONE',  ( 0.000000000000000000, 19.00000000000000000, 208.0000000000000000 ) ) ;
#11603=CARTESIAN_POINT ( 'NONE',  ( -122.2593324768359935, 30.00000000000000000, -168.2755348299880040 ) ) ;
#11604=ORIENTED_EDGE ( 'NONE', *, *, #1008, .T. ) ;
#11606=DIRECTION ( 'NONE',  ( 0.000000000000000000, -1.000000000000000000, 0.000000000000000000 ) ) ;
#11609=AXIS2_PLACEMENT_3D ( 'NONE', #3201, #6287, #11346 ) ;
#11611=DIRECTION ( 'NONE',  ( 0.000000000000000000, -1.000000000000000000, 0.000000000000000000 ) ) ;
#11618=CIRCLE ( 'NONE', #2247, 249.7999999999999829 ) ;
#11620=ORIENTED_EDGE ( 'NONE', *, *, #5568, .T. ) ;
#11621=EDGE_LOOP ( 'NONE', ( #6041, #1528 ) ) ;
#11626=FACE_OUTER_BOUND ( 'NONE', #2080, .T. ) ;
#11629=DIRECTION ( 'NONE',  ( 0.000000000000000000, 0.000000000000000000, -1.000000000000000000 ) ) ;
#11632=EDGE_CURVE ( 'NONE', #1648, #7179, #4246, .T. ) ;
#11633=ORIENTED_EDGE ( 'NONE', *, *, #11459, .T. ) ;
#11639=DIRECTION ( 'NONE',  ( 0.000000000000000000, 0.000000000000000000, 1.000000000000000000 ) ) ;
#11641=CARTESIAN_POINT ( 'NONE',  ( 239.4717458111675228, 1.490203034907673807, -3.166904956765172141 ) ) ;
#11644=CYLINDRICAL_SURFACE ( 'NONE', #9439, 5.099999999999993427 ) ;
#11646=CARTESIAN_POINT ( 'NONE',  ( -238.8031819202592487, -0.6747694104200937515, 11.73074746694206283 ) ) ;
#11649=CARTESIAN_POINT ( 'NONE',  ( -243.0711418334325629, 7.372150985330255146, -9.149572406936686164 ) ) ;
#11650=CARTESIAN_POINT ( 'NONE',  ( 122.2593324768334071, 30.00000000000000000, -168.2755348299895104 ) ) ;
#11651=B_SPLINE_CURVE_WITH_KNOTS ( 'NONE', 3,
 ( #2904, #5721, #792, #12855, #6734, #10988, #9781, #8858, #3721, #11856, #2703, #8726, #7851, #12919, #9710, #10852, #858, #3648, #5792, #5925, #4710, #6988, #1860, #1726, #9852, #732, #4782, #10784, #3919, #2772, #3780, #11923, #6861, #4641, #2841, #1596, #10919, #1796, #4847, #8925, #1655, #3850, #6928, #9990, #4916, #8991, #12053, #11539, #7719, #7993, #5657, #12784, #11801, #10172, #8261, #4247, #10312, #925, #3240, #8328, #12316, #5248, #1052, #7255, #7126, #5176, #4049, #10114, #11116, #1192, #12120, #6120, #12257, #11183, #8198, #2976, #2049, #988, #5041, #5775, #9115, #12386, #3108, #3978, #248, #1986, #9257, #8053, #5111, #3174, #11053, #9317, #4982, #1924, #5994, #11320, #6263, #2114, #2183 ),
 .UNSPECIFIED., .F., .F.,
 ( 4, 2, 2, 1, 1, 2, 2, 2, 2, 1, 1, 1, 2, 2, 2, 2, 1, 1, 1, 1, 2, 2, 2, 2, 1, 1, 1, 1, 2, 2, 2, 2, 2, 2, 1, 1, 1, 1, 2, 2, 2, 2, 1, 1, 1, 1, 2, 2, 2, 2, 1, 1, 1, 1, 2, 2, 2, 2, 1, 1, 2, 2, 4 ),
 ( 0.000000000000000000, 0.03125000000005733608, 0.04687500000008829742, 0.05468750000010186990, 0.05859375000010871165, 0.06054687500011050189, 0.06250000000011228518, 0.09375000000013149204, 0.1093750000001398603, 0.1171875000001438988, 0.1210937500001458555, 0.1230468750001459111, 0.1240234375001469658, 0.1250000000001480205, 0.1875000000001324496, 0.2187500000001246225, 0.2343750000001203482, 0.2421875000001185441, 0.2460937500001179057, 0.2480468750001177947, 0.2490234375001177114, 0.2500000000001176281, 0.3125000000001167400, 0.3437500000001161293, 0.3593750000001158518, 0.3671875000001156297, 0.3710937500001154077, 0.3730468750001152967, 0.3740234375001151856, 0.3750000000001150746, 0.4375000000001111333, 0.5000000000001071365, 0.5625000000001032507, 0.5937500000001012523, 0.6093750000001003642, 0.6171875000000999201, 0.6210937500000995870, 0.6230468750000994760, 0.6240234375000994760, 0.6250000000000993650, 0.6875000000000954792, 0.7187500000000934808, 0.7343750000000922595, 0.7421875000000917044, 0.7460937500000911493, 0.7480468750000904832, 0.7490234375000901501, 0.7500000000000898170, 0.8125000000000358602, 0.8437500000000095479, 0.8593749999999962252, 0.8671874999999906741, 0.8710937499999866773, 0.8730468749999857891, 0.8740234374999852340, 0.8749999999999846789, 0.9062499999999700240, 0.9218749999999626965, 0.9296874999999605871, 0.9335937499999594769, 0.9355468749999606981, 0.9374999999999619194, 1.000000000000000000 ),
 .UNSPECIFIED. ) ;
#11652=DIRECTION ( 'NONE',  ( 0.000000000000000000, 0.000000000000000000, 1.000000000000000000 ) ) ;
#11656=CARTESIAN_POINT ( 'NONE',  ( -229.8594613498277397, 8.573669842083557313, 8.043715334378049420 ) ) ;
#11663=EDGE_CURVE ( 'NONE', #12029, #12239, #7775, .T. ) ;
#11665=ORIENTED_EDGE ( 'NONE', *, *, #2051, .F. ) ;
#11667=ORIENTED_EDGE ( 'NONE', *, *, #11354, .F. ) ;
#11673=DIRECTION ( 'NONE',  ( 0.000000000000000000, -1.000000000000000000, 0.000000000000000000 ) ) ;
#11675=DIRECTION ( 'NONE',  ( 0.000000000000000000, 1.000000000000000000, 0.000000000000000000 ) ) ;
#11677=CARTESIAN_POINT ( 'NONE',  ( -229.8890080036733821, -9.338233916645270583, -7.173345918784452380 ) ) ;
#11680=LINE ( 'NONE', #3398, #8148 ) ;
#11686=VECTOR ( 'NONE', #4377, 1000.000000000000000 ) ;
#11688=AXIS2_PLACEMENT_3D ( 'NONE', #5612, #11820, #3474 ) ;
#11690=EDGE_CURVE ( 'NONE', #7101, #808, #1480, .T. ) ;
#11692=DIRECTION ( 'NONE',  ( 0.000000000000000000, 1.000000000000000000, 0.000000000000000000 ) ) ;
#11695=AXIS2_PLACEMENT_3D ( 'NONE', #1599, #2709, #5865 ) ;
#11703=ORIENTED_EDGE ( 'NONE', *, *, #9370, .F. ) ;
#11706=ADVANCED_FACE ( 'NONE', ( #8777 ), #11906, .F. ) ;
#11707=FACE_OUTER_BOUND ( 'NONE', #4949, .T. ) ;
#11710=DIRECTION ( 'NONE',  ( 0.000000000000000000, -0.7071067811865489050, -0.7071067811865460184 ) ) ;
#11714=CARTESIAN_POINT ( 'NONE',  ( -238.9237350116528660, -1.003861713588480420, 11.70704244028693886 ) ) ;
#11716=CARTESIAN_POINT ( 'NONE',  ( -244.1571280506203152, 8.217568834458665705, -8.398466971310503126 ) ) ;
#11723=CARTESIAN_POINT ( 'NONE',  ( -122.2593324768321992, 30.00000000000000000, 162.7755348299905052 ) ) ;
#11728=ORIENTED_EDGE ( 'NONE', *, *, #7250, .T. ) ;
#11737=EDGE_LOOP ( 'NONE', ( #7852, #3007, #7608, #7575 ) ) ;
#11738=CARTESIAN_POINT ( 'NONE',  ( -122.2593324768321992, 19.00000000000000000, 168.2755348299905052 ) ) ;
#11741=CARTESIAN_POINT ( 'NONE',  ( 229.9983344328827286, 3.389070926892647773, 0.9034159009639075588 ) ) ;
#11747=DIRECTION ( 'NONE',  ( 0.000000000000000000, 1.000000000000000000, 0.000000000000000000 ) ) ;
#11749=ORIENTED_EDGE ( 'NONE', *, *, #9220, .T. ) ;
#11750=DIRECTION ( 'NONE',  ( -1.000000000000000000, 0.000000000000000000, 0.000000000000000000 ) ) ;
#11751=LINE ( 'NONE', #5678, #11219 ) ;
#11757=DIRECTION ( 'NONE',  ( 0.000000000000000000, 0.000000000000000000, -1.000000000000000000 ) ) ;
#11759=FACE_OUTER_BOUND ( 'NONE', #1083, .T. ) ;
#11760=ORIENTED_EDGE ( 'NONE', *, *, #579, .F. ) ;
#11771=DIRECTION ( 'NONE',  ( -1.224646799147349509E-16, 0.000000000000000000, -1.000000000000000000 ) ) ;
#11772=AXIS2_PLACEMENT_3D ( 'NONE', #5949, #5004, #9077 ) ;
#11777=DIRECTION ( 'NONE',  ( 0.000000000000000000, 0.000000000000000000, 1.000000000000000000 ) ) ;
#11779=EDGE_CURVE ( 'NONE', #2818, #12564, #5958, .T. ) ;
#11781=EDGE_CURVE ( 'NONE', #8160, #10938, #2795, .T. ) ;
#11794=DIRECTION ( 'NONE',  ( 0.000000000000000000, 1.000000000000000000, 0.000000000000000000 ) ) ;
#11801=CARTESIAN_POINT ( 'NONE',  ( -249.7944461408548307, -11.69162236593179927, 1.179780703821899479 ) ) ;
#11802=ORIENTED_EDGE ( 'NONE', *, *, #2529, .F. ) ;
#11807=CARTESIAN_POINT ( 'NONE',  ( -197.8197553893924976, 29.00000000000000000, -64.27553482998719403 ) ) ;
#11812=CARTESIAN_POINT ( 'NONE',  ( 229.9799616755531133, 1.752001039403962013, -3.038685965070802908 ) ) ;
#11814=CARTESIAN_POINT ( 'NONE',  ( -249.7838850256576393, 11.60404975224821911, 1.846229155174516023 ) ) ;
#11818=ORIENTED_EDGE ( 'NONE', *, *, #4920, .F. ) ;
#11820=DIRECTION ( 'NONE',  ( 0.000000000000000000, 1.000000000000000000, 0.000000000000000000 ) ) ;
#11824=DIRECTION ( 'NONE',  ( 0.000000000000000000, 1.000000000000000000, 0.000000000000000000 ) ) ;
#11826=AXIS2_PLACEMENT_3D ( 'NONE', #6996, #1998, #12998 ) ;
#11829=EDGE_CURVE ( 'NONE', #5993, #10052, #8182, .T. ) ;
#11835=DIRECTION ( 'NONE',  ( 0.000000000000000000, 1.000000000000000000, 0.000000000000000000 ) ) ;
#11836=DIRECTION ( 'NONE',  ( 0.000000000000000000, 0.000000000000000000, 1.000000000000000000 ) ) ;
#11838=CARTESIAN_POINT ( 'NONE',  ( -122.2593324768359935, 19.00000000000000000, -173.7755348299880040 ) ) ;
#11839=ORIENTED_EDGE ( 'NONE', *, *, #11419, .F. ) ;
#11840=FACE_OUTER_BOUND ( 'NONE', #3060, .T. ) ;
#11841=VERTEX_POINT ( 'NONE', #5980 ) ;
#11842=CARTESIAN_POINT ( 'NONE',  ( -241.1122039833427380, 5.014049992556535607, -10.62747927431669837 ) ) ;
#11844=CARTESIAN_POINT ( 'NONE',  ( 240.1928509381488368, -2.335100009099129181, -2.607195044886591706 ) ) ;
#11846=DIRECTION ( 'NONE',  ( 0.000000000000000000, -1.000000000000000000, 0.000000000000000000 ) ) ;
#11848=DIRECTION ( 'NONE',  ( 0.000000000000000000, 0.000000000000000000, -1.000000000000000000 ) ) ;
#11849=ADVANCED_FACE ( 'NONE', ( #4035 ), #49, .T. ) ;
#11853=VERTEX_POINT ( 'NONE', #3027 ) ;
#11855=ORIENTED_EDGE ( 'NONE', *, *, #1769, .T. ) ;
#11856=CARTESIAN_POINT ( 'NONE',  ( -248.8038635818411421, -10.11061836954485926, -5.986481948888957128 ) ) ;
#11860=DIRECTION ( 'NONE',  ( 0.000000000000000000, 0.000000000000000000, 1.000000000000000000 ) ) ;
#11861=CARTESIAN_POINT ( 'NONE',  ( -197.8197553893909912, 30.00000000000000000, 70.77553482999131518 ) ) ;
#11864=LINE ( 'NONE', #10596, #7073 ) ;
#11866=CARTESIAN_POINT ( 'NONE',  ( 229.9733680233430562, 0.2283798993542111577, -3.499999999999966693 ) ) ;
#11870=CARTESIAN_POINT ( 'NONE',  ( -249.7865125416454362, 11.62303781398087921, -1.723091324902960242 ) ) ;
#11872=AXIS2_PLACEMENT_3D ( 'NONE', #11738, #8864, #7928 ) ;
#11876=ORIENTED_EDGE ( 'NONE', *, *, #218, .T. ) ;
#11881=DIRECTION ( 'NONE',  ( 0.000000000000000000, -1.000000000000000000, 0.000000000000000000 ) ) ;
#11888=AXIS2_PLACEMENT_3D ( 'NONE', #8011, #7011, #2133 ) ;
#11890=CARTESIAN_POINT ( 'NONE',  ( 239.9471905437635826, -1.993882481329591450, 2.878173188141093686 ) ) ;
#11896=CARTESIAN_POINT ( 'NONE',  ( -247.4267604609593718, 9.686619269043202252, 6.650504617425251119 ) ) ;
#11900=CARTESIAN_POINT ( 'NONE',  ( 2.816687638038912194E-14, 18.00000000000000000, 230.0000000000000000 ) ) ;
#11901=AXIS2_PLACEMENT_3D ( 'NONE', #11959, #3885, #12086 ) ;
#11903=CARTESIAN_POINT ( 'NONE',  ( -247.6398763875693021, 9.748465891793076210, -6.561428695001272793 ) ) ;
#11906=CONICAL_SURFACE ( 'NONE', #5731, 5.500000000000005329, 0.7853981633974461696 ) ;
#11908=LINE ( 'NONE', #10159, #9400 ) ;
#11909=DIRECTION ( 'NONE',  ( 0.000000000000000000, 0.000000000000000000, 1.000000000000000000 ) ) ;
#11912=FACE_BOUND ( 'NONE', #10130, .T. ) ;
#11915=VERTEX_POINT ( 'NONE', #1435 ) ;
#11920=CIRCLE ( 'NONE', #9794, 6.500000000000005329 ) ;
#11921=VERTEX_POINT ( 'NONE', #10433 ) ;
#11923=CARTESIAN_POINT ( 'NONE',  ( -249.6746543472006294, -11.17527903296180902, -3.629830555839320017 ) ) ;
#11933=CARTESIAN_POINT ( 'NONE',  ( 229.9832377166102333, 2.139172145189874641, 2.779699421282463945 ) ) ;
#11935=CIRCLE ( 'NONE', #10866, 6.500000000000005329 ) ;
#11936=CARTESIAN_POINT ( 'NONE',  ( -249.7846912503109422, 11.60973349265466581, -1.810138449587363807 ) ) ;
#11941=ORIENTED_EDGE ( 'NONE', *, *, #9465, .T. ) ;
#11942=VERTEX_POINT ( 'NONE', #5439 ) ;
#11943=CARTESIAN_POINT ( 'NONE',  ( -239.4550142755241779, -1.775421017243286492, -11.61532944342562956 ) ) ;
#11944=CARTESIAN_POINT ( 'NONE',  ( 0.000000000000000000, -11.79660968244690089, 249.7999999999999829 ) ) ;
#11946=ADVANCED_FACE ( 'NONE', ( #7566 ), #8305, .F. ) ;
#11951=DIRECTION ( 'NONE',  ( 0.000000000000000000, 0.000000000000000000, -1.000000000000000000 ) ) ;
#11956=EDGE_LOOP ( 'NONE', ( #10803, #8436 ) ) ;
#11958=AXIS2_PLACEMENT_3D ( 'NONE', #5559, #12630, #4421 ) ;
#11959=CARTESIAN_POINT ( 'NONE',  ( 0.000000000000000000, -11.79660968244690089, 0.000000000000000000 ) ) ;
#11960=EDGE_LOOP ( 'NONE', ( #3156, #2811, #8230, #5436 ) ) ;
#11961=DIRECTION ( 'NONE',  ( 0.000000000000000000, 1.000000000000000000, 0.000000000000000000 ) ) ;
#11966=ORIENTED_EDGE ( 'NONE', *, *, #3938, .F. ) ;
#11970=CARTESIAN_POINT ( 'NONE',  ( -239.2756941055121445, 1.575846662935195042, 11.64383230858651075 ) ) ;
#11972=CONICAL_SURFACE ( 'NONE', #7925, 6.500000000000005329, 0.7853981633974518317 ) ;
#11974=AXIS2_PLACEMENT_3D ( 'NONE', #3033, #3163, #10164 ) ;
#11978=DIRECTION ( 'NONE',  ( 0.000000000000000000, 0.000000000000000000, 1.000000000000000000 ) ) ;
#11979=FACE_BOUND ( 'NONE', #6322, .T. ) ;
#11986=ORIENTED_EDGE ( 'NONE', *, *, #12177, .T. ) ;
#11989=ORIENTED_EDGE ( 'NONE', *, *, #2230, .T. ) ;
#11995=AXIS2_PLACEMENT_3D ( 'NONE', #150, #12344, #211 ) ;
#11996=AXIS2_PLACEMENT_3D ( 'NONE', #2292, #6377, #2430 ) ;
#12000=AXIS2_PLACEMENT_3D ( 'NONE', #8369, #4410, #228 ) ;
#12003=CARTESIAN_POINT ( 'NONE',  ( -122.2593324768321992, 18.00000000000000000, 174.7755348299905052 ) ) ;
#12007=CARTESIAN_POINT ( 'NONE',  ( -229.9491826271834327, -10.71030805289945853, 4.847677504751631616 ) ) ;
#12010=ORIENTED_EDGE ( 'NONE', *, *, #12791, .T. ) ;
#12012=DIRECTION ( 'NONE',  ( 0.000000000000000000, 0.000000000000000000, -1.000000000000000000 ) ) ;
#12021=CARTESIAN_POINT ( 'NONE',  ( -243.8540711424298024, -8.004651151255652408, 8.601279216952042006 ) ) ;
#12024=CIRCLE ( 'NONE', #11609, 6.500000000000000000 ) ;
#12026=ORIENTED_EDGE ( 'NONE', *, *, #1466, .F. ) ;
#12029=VERTEX_POINT ( 'NONE', #9500 ) ;
#12030=CARTESIAN_POINT ( 'NONE',  ( -249.6197023356864406, 11.04161720034240268, 4.018949318582678565 ) ) ;
#12037=CARTESIAN_POINT ( 'NONE',  ( -239.2060324291192615, 1.486384971936542065, 11.65560575465026538 ) ) ;
#12039=VECTOR ( 'NONE', #9492, 1000.000000000000000 ) ;
#12042=CARTESIAN_POINT ( 'NONE',  ( 240.3318468625426476, 2.620158398681741829, 2.323190430345948521 ) ) ;
#12044=CARTESIAN_POINT ( 'NONE',  ( -229.9960196359727433, 11.67278588814162532, 1.547559380408666252 ) ) ;
#12050=CARTESIAN_POINT ( 'NONE',  ( -238.9707249641996611, -1.103996724206196323, -11.69802420276602462 ) ) ;
#12052=EDGE_LOOP ( 'NONE', ( #10095, #3843 ) ) ;
#12053=CARTESIAN_POINT ( 'NONE',  ( -249.7894049738271178, -11.64306034850750571, -1.598052574140636839 ) ) ;
#12061=EDGE_CURVE ( 'NONE', #2233, #8497, #5531, .T. ) ;
#12065=ADVANCED_BREP_SHAPE_REPRESENTATION ( '', ( #5959, #805 ), #1235 ) ;
#12067=ORIENTED_EDGE ( 'NONE', *, *, #9538, .T. ) ;
#12072=CARTESIAN_POINT ( 'NONE',  ( 239.0740262672602796, -0.7008254641704574350, -3.430151065624111428 ) ) ;
#12080=CARTESIAN_POINT ( 'NONE',  ( 3.034674768287141263E-14, 11.79660968244690089, -247.7999999999999829 ) ) ;
#12083=ORIENTED_EDGE ( 'NONE', *, *, #12898, .T. ) ;
#12086=DIRECTION ( 'NONE',  ( 0.000000000000000000, 0.000000000000000000, 1.000000000000000000 ) ) ;
#12089=CARTESIAN_POINT ( 'NONE',  ( -248.8038635818159889, 10.11061836954053739, 5.986481948896264171 ) ) ;
#12093=CARTESIAN_POINT ( 'NONE',  ( -244.2656328542583424, 8.290010952302944602, 8.326962424296340259 ) ) ;
#12098=EDGE_LOOP ( 'NONE', ( #12620, #10508, #4965, #10228 ) ) ;
#12099=CARTESIAN_POINT ( 'NONE',  ( -246.6344430665329810, 9.451372532324468168, -6.980988235906895767 ) ) ;
#12101=EDGE_CURVE ( 'NONE', #11051, #3781, #12352, .T. ) ;
#12103=CARTESIAN_POINT ( 'NONE',  ( 239.9543636724889382, 1.989473563526599875, 2.884354563413217942 ) ) ;
#12106=CARTESIAN_POINT ( 'NONE',  ( 0.000000000000000000, 30.00000000000000000, -208.0000000000000000 ) ) ;
#12107=ADVANCED_FACE ( 'NONE', ( #11707 ), #1699, .F. ) ;
#12108=AXIS2_PLACEMENT_3D ( 'NONE', #8862, #7791, #11860 ) ;
#12110=VECTOR ( 'NONE', #6762, 1000.000000000000000 ) ;
#12111=FACE_OUTER_BOUND ( 'NONE', #1727, .T. ) ;
#12115=ORIENTED_EDGE ( 'NONE', *, *, #1916, .T. ) ;
#12116=CIRCLE ( 'NONE', #5945, 5.499999999999998224 ) ;
#12117=CARTESIAN_POINT ( 'NONE',  ( -239.2756941175678662, -1.575846677702103404, -11.64383230647870882 ) ) ;
#12120=CARTESIAN_POINT ( 'NONE',  ( -249.6805863676327135, -11.19144319997654691, 3.579693128109238121 ) ) ;
#12123=DIRECTION ( 'NONE',  ( 0.000000000000000000, 0.000000000000000000, -1.000000000000000000 ) ) ;
#12124=CIRCLE ( 'NONE', #8299, 5.500000000000005329 ) ;
#12125=DIRECTION ( 'NONE',  ( 1.000000000000000000, 0.000000000000000000, 0.000000000000000000 ) ) ;
#12126=CARTESIAN_POINT ( 'NONE',  ( -241.6806182408534198, -5.858727366165308759, -10.18566440464593192 ) ) ;
#12130=CARTESIAN_POINT ( 'NONE',  ( 239.7985776503645354, -1.848645179573700004, 2.971954070984049956 ) ) ;
#12132=CARTESIAN_POINT ( 'NONE',  ( -229.7187050399571149, -3.051684812259986224, 11.37273813590071114 ) ) ;
#12133=CIRCLE ( 'NONE', #2965, 248.1666666666679930 ) ;
#12136=EDGE_LOOP ( 'NONE', ( #2348, #8091, #5122, #12754, #11760, #11665 ) ) ;
#12137=ORIENTED_EDGE ( 'NONE', *, *, #6654, .T. ) ;
#12142=CARTESIAN_POINT ( 'NONE',  ( -122.2593324768359935, 19.00000000000000000, -173.7755348299880040 ) ) ;
#12147=AXIS2_PLACEMENT_3D ( 'NONE', #10310, #1191, #5246 ) ;
#12148=CARTESIAN_POINT ( 'NONE',  ( -241.1122039834657471, -5.014049992762013019, 10.62747927426260830 ) ) ;
#12153=ORIENTED_EDGE ( 'NONE', *, *, #4288, .T. ) ;
#12154=EDGE_LOOP ( 'NONE', ( #841, #2770, #1566, #2677 ) ) ;
#12162=CARTESIAN_POINT ( 'NONE',  ( -246.7156022632958354, 9.478660875630390947, 6.943882024157772115 ) ) ;
#12164=ORIENTED_EDGE ( 'NONE', *, *, #1805, .F. ) ;
#12165=CARTESIAN_POINT ( 'NONE',  ( -239.1649934585021526, -1.429824766643149392, 11.66268491156429299 ) ) ;
#12166=EDGE_LOOP ( 'NONE', ( #4358, #1136, #10672, #5961 ) ) ;
#12167=CARTESIAN_POINT ( 'NONE',  ( -238.9324305446047561, 1.023275410052343792, 11.70536273167116015 ) ) ;
#12168=ORIENTED_EDGE ( 'NONE', *, *, #7960, .F. ) ;
#12172=CARTESIAN_POINT ( 'NONE',  ( 0.000000000000000000, 0.000000000000000000, 0.000000000000000000 ) ) ;
#12173=DIRECTION ( 'NONE',  ( 0.000000000000000000, 0.000000000000000000, -1.000000000000000000 ) ) ;
#12177=EDGE_CURVE ( 'NONE', #3851, #5207, #11139, .T. ) ;
#12180=ORIENTED_EDGE ( 'NONE', *, *, #12657, .T. ) ;
#12182=AXIS2_PLACEMENT_3D ( 'NONE', #10300, #6179, #4171 ) ;
#12184=VECTOR ( 'NONE', #9409, 1000.000000000000000 ) ;
#12185=CARTESIAN_POINT ( 'NONE',  ( -249.6805863676831336, 11.19144320009710469, -3.579693127732738400 ) ) ;
#12187=EDGE_CURVE ( 'NONE', #3500, #552, #10421, .T. ) ;
#12189=ORIENTED_EDGE ( 'NONE', *, *, #4259, .T. ) ;
#12193=DIRECTION ( 'NONE',  ( 0.000000000000000000, 1.000000000000000000, 0.000000000000000000 ) ) ;
#12195=CARTESIAN_POINT ( 'NONE',  ( -247.4267604613398532, -9.686619269140154032, -6.650504617316419953 ) ) ;
#12196=AXIS2_PLACEMENT_3D ( 'NONE', #9748, #3623, #7890 ) ;
#12198=ADVANCED_FACE ( 'NONE', ( #7012 ), #3997, .F. ) ;
#12200=B_SPLINE_CURVE_WITH_KNOTS ( 'NONE', 3,
 ( #3011, #11155, #10089, #962, #1894, #9406, #12407, #6279, #2264, #12089, #11021, #207, #10331, #5966, #4953, #8027, #2946, #3258, #7028, #273, #4330, #8409, #7338, #12470, #5019, #7963, #12030, #3193, #11090, #1957, #6032, #1207, #9091, #5266, #9869, #8738, #9722, #12255, #2718, #6809, #4658, #674, #746, #11814, #8942, #5808, #804, #7735, #7122, #8868, #4046, #5875, #4794, #12868, #4866, #3732, #11870, #2047, #13002, #11936, #3798, #7798, #10867, #9930, #12931, #1740, #1812, #7865, #2787, #8125, #12185, #2657, #6684, #11180, #5670, #9795, #3039, #6116, #10170, #8804, #1049, #6873, #4114, #12798, #10935, #5107, #9185, #61, #8194, #10737, #1608, #3664, #608, #6748, #10799, #1668, #5738, #4727, #5313 ),
 .UNSPECIFIED., .F., .F.,
 ( 4, 2, 2, 1, 1, 2, 2, 2, 2, 1, 1, 1, 2, 2, 2, 2, 1, 1, 1, 1, 2, 2, 2, 2, 1, 1, 1, 1, 2, 2, 2, 2, 2, 2, 1, 1, 1, 1, 2, 2, 2, 2, 1, 1, 1, 1, 2, 2, 2, 2, 1, 1, 1, 1, 2, 2, 2, 2, 1, 1, 2, 2, 4 ),
 ( 0.000000000000000000, 0.03124999999991832922, 0.04687499999987972815, 0.05468749999986047272, 0.05859374999984917620, 0.06054687499984517940, 0.06249999999984116872, 0.09374999999978388121, 0.1093749999997537803, 0.1171874999997375294, 0.1210937499997304517, 0.1230468749997259831, 0.1240234374997236794, 0.1249999999997213895, 0.1874999999997175870, 0.2187499999997155886, 0.2343749999997146727, 0.2421874999997142286, 0.2460937499997137290, 0.2480468749997132016, 0.2490234374997132294, 0.2499999999997132294, 0.3124999999997412070, 0.3437499999997550848, 0.3593749999997621347, 0.3671874999997655764, 0.3710937499997672973, 0.3730468749997681299, 0.3740234374997685185, 0.3749999999997689071, 0.4374999999997900013, 0.4999999999998111511, 0.5624999999998323563, 0.5937499999998429034, 0.6093749999998482325, 0.6171874999998508970, 0.6210937499998521183, 0.6230468749998526734, 0.6240234374998528954, 0.6249999999998531175, 0.6874999999998686606, 0.7187499999998766542, 0.7343749999998807620, 0.7421874999998827604, 0.7460937499998835376, 0.7480468749998843148, 0.7490234374998846478, 0.7499999999998849809, 0.8124999999999326095, 0.8437499999999562572, 0.8593749999999672484, 0.8671874999999736877, 0.8710937499999769074, 0.8730468749999797939, 0.8740234374999813483, 0.8749999999999829026, 0.9062499999999995559, 0.9218750000000092149, 0.9296875000000139888, 0.9335937500000182077, 0.9355468750000203171, 0.9375000000000224265, 1.000000000000000000 ),
 .UNSPECIFIED. ) ;
#12202=DIRECTION ( 'NONE',  ( 0.000000000000000000, 0.000000000000000000, 1.000000000000000000 ) ) ;
#12204=CIRCLE ( 'NONE', #11995, 248.1666666666679930 ) ;
#12206=CARTESIAN_POINT ( 'NONE',  ( -229.6996680450366171, 1.438960022146944131E-15, 11.75000000000000000 ) ) ;
#12211=FACE_OUTER_BOUND ( 'NONE', #1688, .T. ) ;
#12212=CYLINDRICAL_SURFACE ( 'NONE', #430, 5.500000000000005329 ) ;
#12214=DIRECTION ( 'NONE',  ( 0.000000000000000000, 1.000000000000000000, 0.000000000000000000 ) ) ;
#12218=AXIS2_PLACEMENT_3D ( 'NONE', #5751, #11881, #11757 ) ;
#12219=CARTESIAN_POINT ( 'NONE',  ( -243.2974363556361084, -7.571041504521477172, 8.986772704220435060 ) ) ;
#12220=VERTEX_POINT ( 'NONE', #947 ) ;
#12221=DIRECTION ( 'NONE',  ( 8.659560562354939021E-17, 0.7071067811865470176, -0.7071067811865480168 ) ) ;
#12226=CARTESIAN_POINT ( 'NONE',  ( -122.2593324768359935, 30.00000000000000000, -168.2755348299880040 ) ) ;
#12227=DIRECTION ( 'NONE',  ( 0.000000000000000000, 0.000000000000000000, -1.000000000000000000 ) ) ;
#12231=CARTESIAN_POINT ( 'NONE',  ( -242.2247058965207316, 6.524571383469930375, 9.772025480168560208 ) ) ;
#12233=EDGE_CURVE ( 'NONE', #9495, #3412, #8368, .T. ) ;
#12239=VERTEX_POINT ( 'NONE', #1627 ) ;
#12241=EDGE_LOOP ( 'NONE', ( #6089, #3857 ) ) ;
#12244=DIRECTION ( 'NONE',  ( 0.000000000000000000, -1.000000000000000000, 0.000000000000000000 ) ) ;
#12245=FACE_OUTER_BOUND ( 'NONE', #8885, .T. ) ;
#12247=CARTESIAN_POINT ( 'NONE',  ( -210.0000000000000000, 19.40000000000000213, -5.100000000000000533 ) ) ;
#12248=CARTESIAN_POINT ( 'NONE',  ( 122.2593324768334071, 29.00000000000000000, -173.7755348299895104 ) ) ;
#12250=ORIENTED_EDGE ( 'NONE', *, *, #9658, .T. ) ;
#12255=CARTESIAN_POINT ( 'NONE',  ( -249.7621493471160363, 11.48044694377630925, 2.508021713178596013 ) ) ;
#12257=CARTESIAN_POINT ( 'NONE',  ( -249.6784491604580296, -11.18557168011258618, 3.597985675147115980 ) ) ;
#12258=VERTEX_POINT ( 'NONE', #12142 ) ;
#12261=EDGE_CURVE ( 'NONE', #11582, #9692, #4685, .T. ) ;
#12263=DIRECTION ( 'NONE',  ( 0.000000000000000000, 1.000000000000000000, 0.000000000000000000 ) ) ;
#12264=CARTESIAN_POINT ( 'NONE',  ( -245.5121636064574773, -8.994012747014300757, -7.561165846882150987 ) ) ;
#12270=VERTEX_POINT ( 'NONE', #274 ) ;
#12271=EDGE_LOOP ( 'NONE', ( #5278, #10833, #4625, #5242 ) ) ;
#12273=EDGE_CURVE ( 'NONE', #5446, #2165, #636, .T. ) ;
#12275=CARTESIAN_POINT ( 'NONE',  ( 239.1910253111499287, -1.013189013416512463, -3.350157823600272700 ) ) ;
#12285=ORIENTED_EDGE ( 'NONE', *, *, #579, .T. ) ;
#12286=VERTEX_POINT ( 'NONE', #11409 ) ;
#12293=CARTESIAN_POINT ( 'NONE',  ( -246.4924783649346125, 9.403937930409544066, 7.045599365780679690 ) ) ;
#12294=ORIENTED_EDGE ( 'NONE', *, *, #6723, .T. ) ;
#12299=ORIENTED_EDGE ( 'NONE', *, *, #2286, .F. ) ;
#12300=CIRCLE ( 'NONE', #6769, 240.3921568627444856 ) ;
#12305=CARTESIAN_POINT ( 'NONE',  ( 239.0740262672538563, 0.7008254641484221725, 3.430151065625266060 ) ) ;
#12308=DIRECTION ( 'NONE',  ( 0.000000000000000000, 0.000000000000000000, 1.000000000000000000 ) ) ;
#12313=CARTESIAN_POINT ( 'NONE',  ( 122.2593324768334071, 30.00000000000000000, -162.7755348299894820 ) ) ;
#12316=CARTESIAN_POINT ( 'NONE',  ( -249.7845350862966995, -11.60862138559210877, 1.817256862172399234 ) ) ;
#12317=CIRCLE ( 'NONE', #5288, 249.2999999999999829 ) ;
#12318=EDGE_LOOP ( 'NONE', ( #765, #310, #1490, #11303 ) ) ;
#12322=CIRCLE ( 'NONE', #398, 239.8169934640564804 ) ;
#12326=DIRECTION ( 'NONE',  ( 0.000000000000000000, 0.000000000000000000, -1.000000000000000000 ) ) ;
#12329=CARTESIAN_POINT ( 'NONE',  ( -242.3794917446704460, -6.695067658966850743, -9.656064786588574478 ) ) ;
#12330=CARTESIAN_POINT ( 'NONE',  ( 239.2930894855859947, -1.216635601170958036, 3.281912597181230407 ) ) ;
#12332=ADVANCED_FACE ( 'NONE', ( #82 ), #5093, .F. ) ;
#12333=CARTESIAN_POINT ( 'NONE',  ( 0.000000000000000000, 19.00000000000000000, -202.4999999999999716 ) ) ;
#12336=AXIS2_PLACEMENT_3D ( 'NONE', #5208, #5345, #12351 ) ;
#12337=CARTESIAN_POINT ( 'NONE',  ( 0.000000000000000000, -2.957522019940860139E-14, 0.000000000000000000 ) ) ;
#12338=ORIENTED_EDGE ( 'NONE', *, *, #2415, .T. ) ;
#12340=DIRECTION ( 'NONE',  ( 0.000000000000000000, -0.7071067811865489050, -0.7071067811865460184 ) ) ;
#12344=DIRECTION ( 'NONE',  ( 0.000000000000000000, 1.000000000000000000, 0.000000000000000000 ) ) ;
#12351=DIRECTION ( 'NONE',  ( 0.000000000000000000, 0.000000000000000000, 1.000000000000000000 ) ) ;
#12352=CIRCLE ( 'NONE', #10642, 6.499999999999999112 ) ;
#12354=CARTESIAN_POINT ( 'NONE',  ( 229.9849328834052926, -2.312147543537095729, -2.637679212737643386 ) ) ;
#12356=ORIENTED_EDGE ( 'NONE', *, *, #2529, .T. ) ;
#12357=EDGE_CURVE ( 'NONE', #7179, #5643, #12409, .T. ) ;
#12359=LINE ( 'NONE', #2083, #3148 ) ;
#12363=CARTESIAN_POINT ( 'NONE',  ( -244.5179878702206793, 8.451416885157774672, 8.163389686018202696 ) ) ;
#12365=ADVANCED_FACE ( 'NONE', ( #8147 ), #12212, .F. ) ;
#12366=VERTEX_POINT ( 'NONE', #11204 ) ;
#12368=EDGE_LOOP ( 'NONE', ( #2569, #4741, #694, #7740 ) ) ;
#12369=CARTESIAN_POINT ( 'NONE',  ( 0.000000000000000000, 22.00000000000000000, 0.000000000000000000 ) ) ;
#12370=ORIENTED_EDGE ( 'NONE', *, *, #1916, .F. ) ;
#12371=ORIENTED_EDGE ( 'NONE', *, *, #7250, .F. ) ;
#12372=DIRECTION ( 'NONE',  ( 0.000000000000000000, 0.000000000000000000, 1.000000000000000000 ) ) ;
#12375=LINE ( 'NONE', #5982, #3654 ) ;
#12376=CARTESIAN_POINT ( 'NONE',  ( -238.7110722354929067, 0.02061376086992028692, -11.74998185356844438 ) ) ;
#12379=ORIENTED_EDGE ( 'NONE', *, *, #9825, .T. ) ;
#12381=CIRCLE ( 'NONE', #3856, 5.100000000000000533 ) ;
#12383=ORIENTED_EDGE ( 'NONE', *, *, #4271, .F. ) ;
#12386=CARTESIAN_POINT ( 'NONE',  ( -249.2901971947345032, -10.52637179445247284, 5.220957665109235535 ) ) ;
#12387=ORIENTED_EDGE ( 'NONE', *, *, #5038, .T. ) ;
#12391=CARTESIAN_POINT ( 'NONE',  ( -241.4660365540256635, -5.559932090034945595, -10.35152193387608044 ) ) ;
#12392=CIRCLE ( 'NONE', #8144, 6.500000000000005329 ) ;
#12393=CARTESIAN_POINT ( 'NONE',  ( 238.9937480945849018, -0.3586231069789287407, 3.486222115773272900 ) ) ;
#12395=EDGE_CURVE ( 'NONE', #1017, #7886, #5267, .T. ) ;
#12398=AXIS2_PLACEMENT_3D ( 'NONE', #8615, #9598, #6420 ) ;
#12400=CARTESIAN_POINT ( 'NONE',  ( 0.000000000000000000, 29.00000000000000000, -249.7999999999999829 ) ) ;
#12402=B_SPLINE_CURVE_WITH_KNOTS ( 'NONE', 3,
 ( #7661, #4588, #2849, #8733, #3593, #4719, #4855, #5870 ),
 .UNSPECIFIED., .F., .F.,
 ( 4, 2, 2, 4 ),
 ( 0.000000000000000000, 0.2500000000000098255, 0.5000000000000196509, 1.000000000000000000 ),
 .UNSPECIFIED. ) ;
#12406=CIRCLE ( 'NONE', #12196, 5.500000000000005329 ) ;
#12407=CARTESIAN_POINT ( 'NONE',  ( -248.7201528608048307, 10.06060527423840334, 6.070293049067540636 ) ) ;
#12409=LINE ( 'NONE', #4070, #8312 ) ;
#12410=DIRECTION ( 'NONE',  ( 0.000000000000000000, 0.000000000000000000, 1.000000000000000000 ) ) ;
#12412=DIRECTION ( 'NONE',  ( 0.000000000000000000, 1.000000000000000000, 0.000000000000000000 ) ) ;
#12415=CARTESIAN_POINT ( 'NONE',  ( 71.82423009839129691, 19.40000000000000213, -192.2354503650404922 ) ) ;
#12416=VERTEX_POINT ( 'NONE', #9526 ) ;
#12421=CARTESIAN_POINT ( 'NONE',  ( 71.82423009839129691, 19.40000000000000213, 197.3354503650404865 ) ) ;
#12423=CIRCLE ( 'NONE', #5396, 6.500000000000005329 ) ;
#12424=CIRCLE ( 'NONE', #12844, 230.0000000000000000 ) ;
#12426=CONICAL_SURFACE ( 'NONE', #10509, 6.500000000000005329, 0.7853981633974490562 ) ;
#12430=CARTESIAN_POINT ( 'NONE',  ( -240.6673884781993706, 4.184756593251726997, 10.97954905608461118 ) ) ;
#12433=VERTEX_POINT ( 'NONE', #2399 ) ;
#12434=DIRECTION ( 'NONE',  ( 8.659560562354913137E-17, -0.7071067811865489050, 0.7071067811865460184 ) ) ;
#12439=ADVANCED_FACE ( 'NONE', ( #3458 ), #405, .F. ) ;
#12440=FACE_BOUND ( 'NONE', #11956, .T. ) ;
#12441=DIRECTION ( 'NONE',  ( 0.000000000000000000, 0.000000000000000000, -1.000000000000000000 ) ) ;
#12442=CARTESIAN_POINT ( 'NONE',  ( 239.2087834362114052, 1.051957556968997842, -3.338183402669812505 ) ) ;
#12444=CARTESIAN_POINT ( 'NONE',  ( -238.9571511871961320, 1.076409201234731272, -11.70061098712747594 ) ) ;
#12446=PLANE ( 'NONE',  #12835 ) ;
#12448=EDGE_LOOP ( 'NONE', ( #6058, #309, #3102, #6971 ) ) ;
#12449=DIRECTION ( 'NONE',  ( 0.000000000000000000, 0.000000000000000000, 1.000000000000000000 ) ) ;
#12450=EDGE_LOOP ( 'NONE', ( #9684, #9088, #2302, #249 ) ) ;
#12451=CARTESIAN_POINT ( 'NONE',  ( 0.000000000000000000, 2.772967769359004908, 240.3921568627449972 ) ) ;
#12455=VERTEX_POINT ( 'NONE', #8475 ) ;
#12460=SURFACE_SIDE_STYLE ('',( #10384 ) ) ;
#12463=FACE_OUTER_BOUND ( 'NONE', #6969, .T. ) ;
#12464=ORIENTED_EDGE ( 'NONE', *, *, #3004, .T. ) ;
#12468=AXIS2_PLACEMENT_3D ( 'NONE', #5509, #9569, #3503 ) ;
#12470=CARTESIAN_POINT ( 'NONE',  ( -249.4468820691694759, 10.72473315980031394, 4.809560401053397882 ) ) ;
#12476=CARTESIAN_POINT ( 'NONE',  ( -248.0831933713610056, -9.830508068705269054, 6.436117704883859147 ) ) ;
#12477=ORIENTED_EDGE ( 'NONE', *, *, #4479, .F. ) ;
#12478=DIRECTION ( 'NONE',  ( 0.000000000000000000, 0.000000000000000000, 1.000000000000000000 ) ) ;
#12481=ORIENTED_EDGE ( 'NONE', *, *, #1628, .T. ) ;
#12483=DIRECTION ( 'NONE',  ( 1.000000000000000000, 0.000000000000000000, -1.224646799147353207E-16 ) ) ;
#12485=FACE_OUTER_BOUND ( 'NONE', #437, .T. ) ;
#12488=CARTESIAN_POINT ( 'NONE',  ( -240.6798348123334108, 4.210664053274118857, 10.96963869245110601 ) ) ;
#12490=EDGE_LOOP ( 'NONE', ( #516, #12026 ) ) ;
#12491=FACE_OUTER_BOUND ( 'NONE', #4279, .T. ) ;
#12492=ADVANCED_FACE ( 'NONE', ( #1467 ), #1908, .F. ) ;
#12494=ADVANCED_FACE ( 'NONE', ( #1407 ), #7458, .F. ) ;
#12496=VERTEX_POINT ( 'NONE', #8731 ) ;
#12497=ORIENTED_EDGE ( 'NONE', *, *, #7872, .F. ) ;
#12498=CARTESIAN_POINT ( 'NONE',  ( 0.000000000000000000, 30.00000000000000000, 0.000000000000000000 ) ) ;
#12499=CARTESIAN_POINT ( 'NONE',  ( -197.8197553893924976, 19.00000000000000000, -58.77553482998720114 ) ) ;
#12501=CARTESIAN_POINT ( 'NONE',  ( 238.9743709119393316, 0.1785824617006206982, -3.500006748978118587 ) ) ;
#12506=EDGE_LOOP ( 'NONE', ( #3722, #3993, #3220, #486 ) ) ;
#12509=EDGE_LOOP ( 'NONE', ( #2900, #6288 ) ) ;
#12515=EDGE_CURVE ( 'NONE', #534, #7886, #11505, .T. ) ;
#12516=DIRECTION ( 'NONE',  ( -1.000000000000000000, -0.000000000000000000, -0.000000000000000000 ) ) ;
#12519=CARTESIAN_POINT ( 'NONE',  ( -240.6673884782285029, -4.184756593312895845, -10.97954905606168907 ) ) ;
#12522=CARTESIAN_POINT ( 'NONE',  ( 239.5494890104657770, -1.589230969769584556, 3.118420702999415095 ) ) ;
#12523=CARTESIAN_POINT ( 'NONE',  ( 240.5500529090693078, 3.279976618980518843, 1.225241158572545785 ) ) ;
#12527=ORIENTED_EDGE ( 'NONE', *, *, #306, .F. ) ;
#12540=CIRCLE ( 'NONE', #6801, 249.7999999999999829 ) ;
#12543=ORIENTED_EDGE ( 'NONE', *, *, #1510, .T. ) ;
#12553=FACE_OUTER_BOUND ( 'NONE', #762, .T. ) ;
#12563=ORIENTED_EDGE ( 'NONE', *, *, #4159, .T. ) ;
#12564=VERTEX_POINT ( 'NONE', #6541 ) ;
#12572=CARTESIAN_POINT ( 'NONE',  ( -239.1938287653389636, 1.469862578567988853, -11.65770166428045584 ) ) ;
#12574=VECTOR ( 'NONE', #7604, 1000.000000000000000 ) ;
#12576=CYLINDRICAL_SURFACE ( 'NONE', #6471, 3.499999999999964917 ) ;
#12578=CARTESIAN_POINT ( 'NONE',  ( -244.0310755671143284, 8.130894654072220007, -8.482269552766895870 ) ) ;
#12584=DIRECTION ( 'NONE',  ( 8.659560562354913137E-17, -0.7071067811865489050, 0.7071067811865460184 ) ) ;
#12586=CARTESIAN_POINT ( 'NONE',  ( 197.8197553893920144, 19.00000000000000000, 64.27553482998850143 ) ) ;
#12589=DIRECTION ( 'NONE',  ( 0.000000000000000000, -0.7071067811865489050, -0.7071067811865460184 ) ) ;
#12591=ADVANCED_FACE ( 'NONE', ( #8662, #3592 ), #6802, .F. ) ;
#12592=AXIS2_PLACEMENT_3D ( 'NONE', #646, #4698, #7832 ) ;
#12602=CARTESIAN_POINT ( 'NONE',  ( 71.82423009839129691, 30.00000000000000000, 192.2354503650404922 ) ) ;
#12605=AXIS2_PLACEMENT_3D ( 'NONE', #8604, #3589, #7657 ) ;
#12610=VERTEX_POINT ( 'NONE', #11861 ) ;
#12611=CARTESIAN_POINT ( 'NONE',  ( 0.000000000000000000, 4.286263797015693701E-16, -3.499999999999964917 ) ) ;
#12613=AXIS2_PLACEMENT_3D ( 'NONE', #4408, #10349, #5482 ) ;
#12615=LINE ( 'NONE', #3479, #906 ) ;
#12618=DIRECTION ( 'NONE',  ( 0.000000000000000000, 0.000000000000000000, 1.000000000000000000 ) ) ;
#12620=ORIENTED_EDGE ( 'NONE', *, *, #200, .F. ) ;
#12624=ORIENTED_EDGE ( 'NONE', *, *, #12061, .F. ) ;
#12625=ORIENTED_EDGE ( 'NONE', *, *, #4801, .T. ) ;
#12627=TOROIDAL_SURFACE ( 'NONE', #7946, 238.4705882352940307, 2.000000000000000000 ) ;
#12628=AXIS2_PLACEMENT_3D ( 'NONE', #7679, #4605, #8680 ) ;
#12630=DIRECTION ( 'NONE',  ( 0.000000000000000000, -1.000000000000000000, 0.000000000000000000 ) ) ;
#12634=EDGE_CURVE ( 'NONE', #8176, #12433, #5323, .T. ) ;
#12635=CARTESIAN_POINT ( 'NONE',  ( -122.2593324768359935, 30.00000000000000000, -162.7755348299880040 ) ) ;
#12639=EDGE_LOOP ( 'NONE', ( #8009, #3683 ) ) ;
#12641=CARTESIAN_POINT ( 'NONE',  ( -238.7275296710179191, -0.3340951308803304376, 11.74628516890670760 ) ) ;
#12642=ORIENTED_EDGE ( 'NONE', *, *, #3708, .T. ) ;
#12649=CARTESIAN_POINT ( 'NONE',  ( -240.1208361041844910, -2.772967769359084844, -11.41810622433049893 ) ) ;
#12650=VECTOR ( 'NONE', #68, 1000.000000000000000 ) ;
#12651=DIRECTION ( 'NONE',  ( 0.000000000000000000, 0.000000000000000000, -1.000000000000000000 ) ) ;
#12653=CARTESIAN_POINT ( 'NONE',  ( 0.000000000000000000, 29.00000000000000000, 0.000000000000000000 ) ) ;
#12656=EDGE_CURVE ( 'NONE', #1432, #7625, #7030, .T. ) ;
#12657=EDGE_CURVE ( 'NONE', #4193, #3121, #12300, .T. ) ;
#12658=LINE ( 'NONE', #7590, #12972 ) ;
#12659=VERTEX_POINT ( 'NONE', #739 ) ;
#12662=DIRECTION ( 'NONE',  ( 0.000000000000000000, 1.000000000000000000, 0.000000000000000000 ) ) ;
#12663=CARTESIAN_POINT ( 'NONE',  ( 3.046921236278614777E-14, -20.00000000000000000, -248.7999999999999829 ) ) ;
#12667=DIRECTION ( 'NONE',  ( 0.000000000000000000, 0.000000000000000000, 1.000000000000000000 ) ) ;
#12669=CARTESIAN_POINT ( 'NONE',  ( -229.7741891532738236, -5.886256761507725699, -10.19824341982703331 ) ) ;
#12671=DIRECTION ( 'NONE',  ( 0.000000000000000000, -1.000000000000000000, 0.000000000000000000 ) ) ;
#12676=VERTEX_POINT ( 'NONE', #4716 ) ;
#12687=ORIENTED_EDGE ( 'NONE', *, *, #3607, .F. ) ;
#12689=ORIENTED_EDGE ( 'NONE', *, *, #5789, .F. ) ;
#12694=CARTESIAN_POINT ( 'NONE',  ( 239.0028278883881399, -0.3789072388328452168, -3.479912193147403521 ) ) ;
#12697=FACE_OUTER_BOUND ( 'NONE', #574, .T. ) ;
#12699=ORIENTED_EDGE ( 'NONE', *, *, #12916, .F. ) ;
#12700=B_SPLINE_CURVE_WITH_KNOTS ( 'NONE', 3,
 ( #4923, #9996, #3725, #7792, #6067, #12195, #3048, #9324, #10180, #4055, #196, #7133, #3983, #11188, #8134, #2189, #10120, #3113, #1197, #10381, #3246, #4253, #2055, #12264, #5183, #11325, #993, #5045, #71, #6269, #1058, #6125, #7327, #4123, #9122, #2982, #1259, #5117, #1996, #7190, #11396, #8204, #11257, #9263, #10318, #9193, #5322, #136, #6197, #2119, #9392, #8060, #8266, #12329, #4186, #10250, #5255, #2256, #8333, #1126, #6330, #3179, #12126, #7261, #12391, #7063, #13040, #11123, #5453, #7390, #4507, #7644, #2448, #5580, #1517, #11530, #12519, #390, #8592, #7456, #12649 ),
 .UNSPECIFIED., .F., .F.,
 ( 4, 1, 1, 1, 2, 2, 2, 1, 1, 1, 2, 2, 2, 2, 1, 1, 1, 1, 2, 2, 2, 2, 1, 1, 1, 2, 2, 2, 1, 1, 1, 2, 2, 2, 2, 1, 1, 1, 2, 2, 2, 1, 1, 1, 2, 2, 2, 1, 1, 1, 2, 2, 4 ),
 ( 0.000000000000000000, 0.03125000000017429114, 0.04687500000026457309, 0.05468750000030974528, 0.05859375000032932684, 0.06250000000034891534, 0.09375000000051852966, 0.1093750000006062650, 0.1171875000006501188, 0.1210937500006691869, 0.1230468750006787210, 0.1250000000006882550, 0.1875000000008141265, 0.2187500000008799350, 0.2343750000009128254, 0.2421875000009293399, 0.2460937500009350576, 0.2480468750009355017, 0.2490234375009333367, 0.2500000000009311441, 0.3125000000007751577, 0.3437500000006971645, 0.3593750000006558087, 0.3671875000006373790, 0.3710937500006282752, 0.3730468750006217249, 0.3750000000006151746, 0.4375000000005053180, 0.4687500000004528045, 0.4843750000004288792, 0.4921875000004191647, 0.4960937500004121703, 0.5000000000004051204, 0.5625000000002996492, 0.5937500000002491340, 0.6093750000002217115, 0.6171875000002102762, 0.6210937500002069456, 0.6230468750002076117, 0.6250000000002082778, 0.6875000000001613154, 0.7187500000001358913, 0.7343750000001232348, 0.7421875000001169065, 0.7460937500001155742, 0.7500000000001142419, 0.8125000000000828226, 0.8437500000000686118, 0.8593750000000600631, 0.8671875000000571765, 0.8710937500000570655, 0.8750000000000569544, 1.000000000000000000 ),
 .UNSPECIFIED. ) ;
#12701=CARTESIAN_POINT ( 'NONE',  ( -238.8961190158434817, -0.9395161414439207048, 11.71239737841137796 ) ) ;
#12703=CARTESIAN_POINT ( 'NONE',  ( -240.8355308712237104, 4.526241345699689944, -10.84528472040825875 ) ) ;
#12704=CARTESIAN_POINT ( 'NONE',  ( 0.000000000000000000, 30.00000000000000000, -201.4999999999999716 ) ) ;
#12709=DIRECTION ( 'NONE',  ( 0.000000000000000000, -1.000000000000000000, 0.000000000000000000 ) ) ;
#12716=DIRECTION ( 'NONE',  ( 0.000000000000000000, 0.000000000000000000, 1.000000000000000000 ) ) ;
#12720=CARTESIAN_POINT ( 'NONE',  ( -248.0831933713610056, -9.830508068705269054, 6.436117704883859147 ) ) ;
#12727=DIRECTION ( 'NONE',  ( 8.659560562354913137E-17, -0.7071067811865489050, 0.7071067811865460184 ) ) ;
#12729=FACE_OUTER_BOUND ( 'NONE', #2142, .T. ) ;
#12730=CARTESIAN_POINT ( 'NONE',  ( 122.2593324768346008, 30.00000000000000000, 161.7755348299889988 ) ) ;
#12738=EDGE_CURVE ( 'NONE', #10046, #5784, #799, .T. ) ;
#12742=CARTESIAN_POINT ( 'NONE',  ( -197.8197553893924976, 19.00000000000000000, -64.27553482998719403 ) ) ;
#12744=CARTESIAN_POINT ( 'NONE',  ( 239.7985776503625175, 1.848645179571945185, 2.971954070985139751 ) ) ;
#12746=CARTESIAN_POINT ( 'NONE',  ( 239.9471905437599730, 1.993882481326073375, -2.878173188143535732 ) ) ;
#12749=CARTESIAN_POINT ( 'NONE',  ( 0.000000000000000000, -11.79660968244690089, 0.000000000000000000 ) ) ;
#12751=AXIS2_PLACEMENT_3D ( 'NONE', #12172, #12244, #3095 ) ;
#12753=ORIENTED_EDGE ( 'NONE', *, *, #2479, .F. ) ;
#12754=ORIENTED_EDGE ( 'NONE', *, *, #6457, .F. ) ;
#12756=AXIS2_PLACEMENT_3D ( 'NONE', #9215, #6893, #12478 ) ;
#12757=DIRECTION ( 'NONE',  ( 0.000000000000000000, 1.000000000000000000, 0.000000000000000000 ) ) ;
#12760=AXIS2_PLACEMENT_3D ( 'NONE', #2679, #6640, #5695 ) ;
#12762=CARTESIAN_POINT ( 'NONE',  ( -239.5361044668155159, 1.848645179572584896, 11.60366368868220022 ) ) ;
#12764=CARTESIAN_POINT ( 'NONE',  ( 0.000000000000000000, 30.00000000000000000, 208.0000000000000000 ) ) ;
#12769=DIRECTION ( 'NONE',  ( 0.000000000000000000, 0.000000000000000000, 1.000000000000000000 ) ) ;
#12772=CARTESIAN_POINT ( 'NONE',  ( 239.9543636722321764, -1.989473563294940961, -2.884354563557201434 ) ) ;
#12775=DIRECTION ( 'NONE',  ( 0.000000000000000000, 1.000000000000000000, 0.000000000000000000 ) ) ;
#12776=CONICAL_SURFACE ( 'NONE', #3200, 6.500000000000005329, 0.7853981633974490562 ) ;
#12777=LINE ( 'NONE', #3640, #12184 ) ;
#12778=CARTESIAN_POINT ( 'NONE',  ( 0.000000000000000000, 19.00000000000000000, 208.0000000000000000 ) ) ;
#12783=ORIENTED_EDGE ( 'NONE', *, *, #10460, .T. ) ;
#12784=CARTESIAN_POINT ( 'NONE',  ( -249.7982158286841639, -11.73176039257149661, 0.7224695965638833206 ) ) ;
#12788=DIRECTION ( 'NONE',  ( 0.000000000000000000, 0.7071067811865450192, 0.7071067811865500152 ) ) ;
#12791=EDGE_CURVE ( 'NONE', #4005, #2425, #12700, .T. ) ;
#12792=LINE ( 'NONE', #800, #1443 ) ;
#12794=LINE ( 'NONE', #12602, #13024 ) ;
#12796=CARTESIAN_POINT ( 'NONE',  ( -229.7194722698235125, -3.038862843935012936, -11.35678684944393346 ) ) ;
#12798=CARTESIAN_POINT ( 'NONE',  ( -249.2754563888320547, 10.50954084450174975, -5.254718384040748091 ) ) ;
#12800=CARTESIAN_POINT ( 'NONE',  ( 0.000000000000000000, 22.00000000000000000, 0.000000000000000000 ) ) ;
#12809=CARTESIAN_POINT ( 'NONE',  ( 0.000000000000000000, 9.830508068699479907, 0.000000000000000000 ) ) ;
#12817=ADVANCED_FACE ( 'NONE', ( #7522 ), #4570, .F. ) ;
#12819=ADVANCED_FACE ( 'NONE', ( #331 ), #9942, .F. ) ;
#12821=ORIENTED_EDGE ( 'NONE', *, *, #5302, .T. ) ;
#12823=CIRCLE ( 'NONE', #1971, 5.499999999999998224 ) ;
#12824=CARTESIAN_POINT ( 'NONE',  ( -197.8197553893924976, 30.00000000000000000, -64.27553482998719403 ) ) ;
#12825=DIRECTION ( 'NONE',  ( 0.000000000000000000, 1.000000000000000000, 0.000000000000000000 ) ) ;
#12833=CONICAL_SURFACE ( 'NONE', #917, 6.500000000000005329, 0.7853981633974518317 ) ;
#12835=AXIS2_PLACEMENT_3D ( 'NONE', #12960, #5839, #10896 ) ;
#12836=CARTESIAN_POINT ( 'NONE',  ( -243.1363860134830759, 7.429686608631851819, -9.102873391464031627 ) ) ;
#12837=EDGE_LOOP ( 'NONE', ( #4113, #4495, #11941, #9727 ) ) ;
#12839=CARTESIAN_POINT ( 'NONE',  ( 240.2635760545757933, -2.467011615924421974, -2.483268943700265741 ) ) ;
#12843=DIRECTION ( 'NONE',  ( 0.000000000000000000, -1.000000000000000000, 0.000000000000000000 ) ) ;
#12844=AXIS2_PLACEMENT_3D ( 'NONE', #3103, #2303, #8454 ) ;
#12848=VERTEX_POINT ( 'NONE', #1390 ) ;
#12851=EDGE_LOOP ( 'NONE', ( #11703, #5361, #12285, #3699 ) ) ;
#12855=CARTESIAN_POINT ( 'NONE',  ( -248.5304950467331082, -9.965644880995725430, -6.224989825265568655 ) ) ;
#12861=CARTESIAN_POINT ( 'NONE',  ( 3.059167704270088292E-14, 29.00000000000000000, 249.7999999999999829 ) ) ;
#12865=AXIS2_PLACEMENT_3D ( 'NONE', #1863, #11120, #12123 ) ;
#12866=CARTESIAN_POINT ( 'NONE',  ( -229.8303177822455439, -7.754159524086684740, -8.836599804383647339 ) ) ;
#12868=CARTESIAN_POINT ( 'NONE',  ( -249.7928741345566834, 11.67611540995070207, -1.322401136026368107 ) ) ;
#12871=EDGE_LOOP ( 'NONE', ( #2647, #5944, #12137, #2364 ) ) ;
#12880=FACE_OUTER_BOUND ( 'NONE', #339, .T. ) ;
#12882=AXIS2_PLACEMENT_3D ( 'NONE', #3858, #4927, #5125 ) ;
#12886=VERTEX_POINT ( 'NONE', #11457 ) ;
#12887=VERTEX_POINT ( 'NONE', #9640 ) ;
#12890=VERTEX_POINT ( 'NONE', #5392 ) ;
#12891=AXIS2_PLACEMENT_3D ( 'NONE', #2802, #8681, #5685 ) ;
#12893=CARTESIAN_POINT ( 'NONE',  ( 239.0510843050431617, -0.6173067666910034834, -3.446156762516083383 ) ) ;
#12895=LINE ( 'NONE', #11838, #5623 ) ;
#12898=EDGE_CURVE ( 'NONE', #4565, #1001, #2847, .T. ) ;
#12900=ORIENTED_EDGE ( 'NONE', *, *, #10673, .T. ) ;
#12903=CARTESIAN_POINT ( 'NONE',  ( -246.5915682062262988, 9.436693423219887578, -7.000847393187709322 ) ) ;
#12904=ORIENTED_EDGE ( 'NONE', *, *, #3195, .T. ) ;
#12905=DIRECTION ( 'NONE',  ( 1.224646799147349509E-16, 0.000000000000000000, -1.000000000000000000 ) ) ;
#12908=CARTESIAN_POINT ( 'NONE',  ( -229.7036030501511732, 1.544435828463907923, -11.67381294332149011 ) ) ;
#12911=EDGE_CURVE ( 'NONE', #468, #12676, #3131, .T. ) ;
#12913=ORIENTED_EDGE ( 'NONE', *, *, #9890, .T. ) ;
#12915=ORIENTED_EDGE ( 'NONE', *, *, #6502, .T. ) ;
#12916=EDGE_CURVE ( 'NONE', #4958, #678, #3838, .T. ) ;
#12917=ORIENTED_EDGE ( 'NONE', *, *, #9709, .F. ) ;
#12919=CARTESIAN_POINT ( 'NONE',  ( -249.0998459883950318, -10.33180199792140819, -5.596503888595450782 ) ) ;
#12926=CARTESIAN_POINT ( 'NONE',  ( 0.000000000000000000, 0.000000000000000000, 0.000000000000000000 ) ) ;
#12928=CARTESIAN_POINT ( 'NONE',  ( 229.9785170508817487, 1.553259044379982301, 3.144732723172867672 ) ) ;
#12931=CARTESIAN_POINT ( 'NONE',  ( -249.7367190369228069, 11.37209550732486640, -2.959943707653969636 ) ) ;
#12942=DIRECTION ( 'NONE',  ( 0.000000000000000000, 1.000000000000000000, 0.000000000000000000 ) ) ;
#12943=CARTESIAN_POINT ( 'NONE',  ( 240.1157413331974908, 2.212437690464817308, -2.712157915439629363 ) ) ;
#12944=ADVANCED_FACE ( 'NONE', ( #10777 ), #6549, .F. ) ;
#12947=LINE ( 'NONE', #1886, #7428 ) ;
#12952=CIRCLE ( 'NONE', #1458, 240.3921568627449687 ) ;
#12954=CARTESIAN_POINT ( 'NONE',  ( 240.0731061099998271, -2.151402440700775909, 2.761193928001421050 ) ) ;
#12957=CARTESIAN_POINT ( 'NONE',  ( -240.1208361041834962, -2.772967769359314882, 11.41810622433041900 ) ) ;
#12960=CARTESIAN_POINT ( 'NONE',  ( -249.7999999999999829, -20.00000000000000000, 0.000000000000000000 ) ) ;
#12961=EDGE_CURVE ( 'NONE', #10559, #10688, #4057, .T. ) ;
#12962=ADVANCED_FACE ( 'NONE', ( #782 ), #7396, .F. ) ;
#12968=ORIENTED_EDGE ( 'NONE', *, *, #3356, .F. ) ;
#12969=CARTESIAN_POINT ( 'NONE',  ( 239.1818646735695211, 0.9924701939458496769, 3.356351167333999630 ) ) ;
#12970=DIRECTION ( 'NONE',  ( 0.000000000000000000, 0.000000000000000000, 1.000000000000000000 ) ) ;
#12972=VECTOR ( 'NONE', #662, 1000.000000000000000 ) ;
#12974=AXIS2_PLACEMENT_3D ( 'NONE', #10567, #2293, #12441 ) ;
#12983=CARTESIAN_POINT ( 'NONE',  ( -238.7112179666109739, -0.03612072660172950533, -11.74994901723889384 ) ) ;
#12986=EDGE_LOOP ( 'NONE', ( #10890, #2523, #7912, #2065, #10143, #8827, #12370, #8389 ) ) ;
#12998=DIRECTION ( 'NONE',  ( 0.000000000000000000, 0.000000000000000000, 1.000000000000000000 ) ) ;
#13002=CARTESIAN_POINT ( 'NONE',  ( -249.7849245721639591, 11.61140107782044240, -1.799432315875151733 ) ) ;
#13003=CARTESIAN_POINT ( 'NONE',  ( 71.82423009839129691, 19.40000000000000213, -197.3354503650404865 ) ) ;
#13004=ORIENTED_EDGE ( 'NONE', *, *, #7193, .T. ) ;
#13005=ORIENTED_EDGE ( 'NONE', *, *, #2878, .T. ) ;
#13008=ADVANCED_FACE ( 'NONE', ( #1804 ), #10157, .F. ) ;
#13011=DIRECTION ( 'NONE',  ( 0.000000000000000000, 1.000000000000000000, 0.000000000000000000 ) ) ;
#13013=CARTESIAN_POINT ( 'NONE',  ( -245.3661487643706209, -8.922833484614967503, 7.644980496220819433 ) ) ;
#13017=FACE_BOUND ( 'NONE', #3646, .T. ) ;
#13019=ORIENTED_EDGE ( 'NONE', *, *, #1030, .T. ) ;
#13020=ORIENTED_EDGE ( 'NONE', *, *, #1466, .T. ) ;
#13022=ORIENTED_EDGE ( 'NONE', *, *, #3747, .T. ) ;
#13023=FACE_OUTER_BOUND ( 'NONE', #12098, .T. ) ;
#13024=VECTOR ( 'NONE', #3658, 1000.000000000000000 ) ;
#13031=VERTEX_POINT ( 'NONE', #12003 ) ;
#13032=CARTESIAN_POINT ( 'NONE',  ( 0.000000000000000000, -19.00000000000000000, 0.000000000000000000 ) ) ;
#13033=VERTEX_POINT ( 'NONE', #12861 ) ;
#13037=EDGE_CURVE ( 'NONE', #3121, #10050, #12402, .T. ) ;
#13039=CARTESIAN_POINT ( 'NONE',  ( 240.0821326533886975, -2.149019271346159776, -2.771577408434056533 ) ) ;
#13040=CARTESIAN_POINT ( 'NONE',  ( -241.3883989931630083, -5.445712471323459702, -10.41186067205816812 ) ) ;
ENDSEC;
END-ISO-10303-21;
